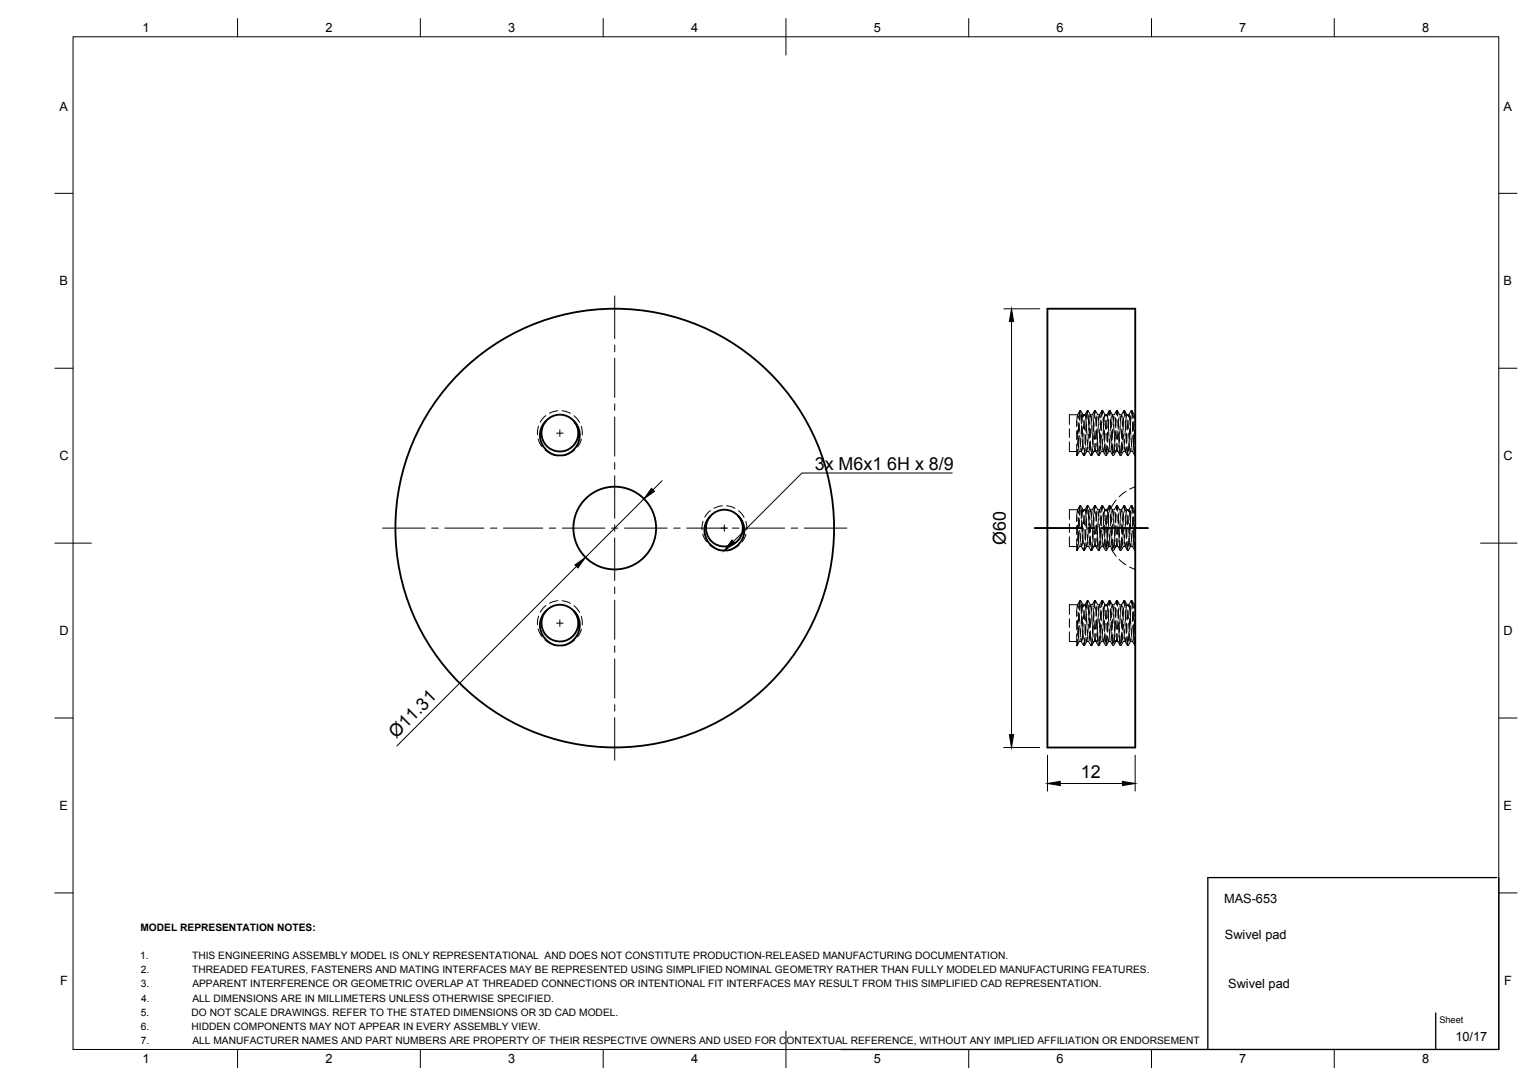
ISO-10303-21;
HEADER;
/* Generated by software containing ST-Developer
 * from STEP Tools, Inc. (www.steptools.com) 
 */

FILE_DESCRIPTION(
/* description */ ('Independent compact industrial fixture table, bolted aluminum worktop
 on connected adjustable support base. Whole-mm nominal dimensions. No
 load rating assigned.'),
/* implementation_level */ '2;1');

FILE_NAME(
/* name */ 'Swivel pad.step',
/* time_stamp */ '2026-11-07T17:47:58-08:00',
/* author */ (''),
/* organization */ (''),
/* preprocessor_version */ 'ST-DEVELOPER v20.2',
/* originating_system */ 'Autodesk Translation Framework v15.17.0.0',
/* authorisation */ '');

FILE_SCHEMA (('AUTOMOTIVE_DESIGN { 1 0 10303 214 3 1 1 }'));
ENDSEC;

DATA;
#10=MECHANICAL_DESIGN_GEOMETRIC_PRESENTATION_REPRESENTATION('',(#2259),#97475);
#11=SPHERICAL_SURFACE('',#22780,6.);
#350=B_SPLINE_SURFACE_WITH_KNOTS('',3,3,((#58329,#58330,#58331,#58332,#58333,
#58334,#58335,#58336,#58337,#58338,#58339,#58340,#58341,#58342,#58343,#58344,
#58345,#58346,#58347,#58348,#58349,#58350,#58351,#58352,#58353,#58354,#58355,
#58356,#58357,#58358,#58359,#58360,#58361,#58362,#58363,#58364,#58365,#58366,
#58367,#58368,#58369,#58370,#58371,#58372,#58373,#58374,#58375,#58376,#58377,
#58378,#58379,#58380,#58381,#58382,#58383,#58384),(#58385,#58386,#58387,
#58388,#58389,#58390,#58391,#58392,#58393,#58394,#58395,#58396,#58397,#58398,
#58399,#58400,#58401,#58402,#58403,#58404,#58405,#58406,#58407,#58408,#58409,
#58410,#58411,#58412,#58413,#58414,#58415,#58416,#58417,#58418,#58419,#58420,
#58421,#58422,#58423,#58424,#58425,#58426,#58427,#58428,#58429,#58430,#58431,
#58432,#58433,#58434,#58435,#58436,#58437,#58438,#58439,#58440),(#58441,
#58442,#58443,#58444,#58445,#58446,#58447,#58448,#58449,#58450,#58451,#58452,
#58453,#58454,#58455,#58456,#58457,#58458,#58459,#58460,#58461,#58462,#58463,
#58464,#58465,#58466,#58467,#58468,#58469,#58470,#58471,#58472,#58473,#58474,
#58475,#58476,#58477,#58478,#58479,#58480,#58481,#58482,#58483,#58484,#58485,
#58486,#58487,#58488,#58489,#58490,#58491,#58492,#58493,#58494,#58495,#58496),
(#58497,#58498,#58499,#58500,#58501,#58502,#58503,#58504,#58505,#58506,
#58507,#58508,#58509,#58510,#58511,#58512,#58513,#58514,#58515,#58516,#58517,
#58518,#58519,#58520,#58521,#58522,#58523,#58524,#58525,#58526,#58527,#58528,
#58529,#58530,#58531,#58532,#58533,#58534,#58535,#58536,#58537,#58538,#58539,
#58540,#58541,#58542,#58543,#58544,#58545,#58546,#58547,#58548,#58549,#58550,
#58551,#58552)),.UNSPECIFIED.,.F.,.F.,.F.,(4,4),(4,1,1,1,1,1,1,1,1,1,1,
1,1,1,1,1,1,1,1,1,1,1,1,1,1,1,1,1,1,1,1,1,1,1,1,1,1,1,1,1,1,1,1,1,1,1,1,
1,1,1,1,1,1,4),(0.,0.0642013499338863),(11.8589888623078,12.8454497557128,
13.8319106491178,14.8183715425228,15.8048324359278,16.7912933293328,17.7777542227378,
18.7642151161429,19.7506760095479,20.7371369029529,21.7235977963579,22.7100586897629,
23.6965195831679,24.6829804765729,25.6694413699779,26.6559022633829,27.6423631567879,
28.6288240501929,29.6152849435979,30.6017458370029,31.5882067304079,32.5746676238129,
33.5611285172179,34.5475894106229,35.5340503040279,36.5205111974329,37.5069720908379,
38.4934329842429,39.4798938776479,40.4663547710529,41.4528156644579,42.4392765578629,
43.4257374512679,44.4121983446729,45.3986592380779,46.3851201314829,47.3715810248879,
48.3580419182929,49.3445028116979,50.3309637051029,51.3174245985079,52.3038854919129,
53.2903463853179,54.2768072787229,55.2632681721279,56.2497290655329,57.2361899589379,
58.222650852343,59.209111745748,60.195572639153,61.182033532558,62.168494425963,
63.154955319368,64.141416212773),.UNSPECIFIED.);
#351=B_SPLINE_SURFACE_WITH_KNOTS('',3,3,((#58669,#58670,#58671,#58672,#58673,
#58674,#58675,#58676,#58677,#58678,#58679,#58680,#58681,#58682,#58683,#58684,
#58685,#58686,#58687,#58688,#58689,#58690,#58691,#58692,#58693,#58694,#58695,
#58696,#58697,#58698,#58699,#58700,#58701,#58702,#58703,#58704,#58705,#58706,
#58707,#58708,#58709,#58710,#58711,#58712,#58713,#58714,#58715,#58716,#58717,
#58718,#58719,#58720,#58721,#58722,#58723,#58724),(#58725,#58726,#58727,
#58728,#58729,#58730,#58731,#58732,#58733,#58734,#58735,#58736,#58737,#58738,
#58739,#58740,#58741,#58742,#58743,#58744,#58745,#58746,#58747,#58748,#58749,
#58750,#58751,#58752,#58753,#58754,#58755,#58756,#58757,#58758,#58759,#58760,
#58761,#58762,#58763,#58764,#58765,#58766,#58767,#58768,#58769,#58770,#58771,
#58772,#58773,#58774,#58775,#58776,#58777,#58778,#58779,#58780),(#58781,
#58782,#58783,#58784,#58785,#58786,#58787,#58788,#58789,#58790,#58791,#58792,
#58793,#58794,#58795,#58796,#58797,#58798,#58799,#58800,#58801,#58802,#58803,
#58804,#58805,#58806,#58807,#58808,#58809,#58810,#58811,#58812,#58813,#58814,
#58815,#58816,#58817,#58818,#58819,#58820,#58821,#58822,#58823,#58824,#58825,
#58826,#58827,#58828,#58829,#58830,#58831,#58832,#58833,#58834,#58835,#58836),
(#58837,#58838,#58839,#58840,#58841,#58842,#58843,#58844,#58845,#58846,
#58847,#58848,#58849,#58850,#58851,#58852,#58853,#58854,#58855,#58856,#58857,
#58858,#58859,#58860,#58861,#58862,#58863,#58864,#58865,#58866,#58867,#58868,
#58869,#58870,#58871,#58872,#58873,#58874,#58875,#58876,#58877,#58878,#58879,
#58880,#58881,#58882,#58883,#58884,#58885,#58886,#58887,#58888,#58889,#58890,
#58891,#58892)),.UNSPECIFIED.,.F.,.F.,.F.,(4,4),(4,1,1,1,1,1,1,1,1,1,1,
1,1,1,1,1,1,1,1,1,1,1,1,1,1,1,1,1,1,1,1,1,1,1,1,1,1,1,1,1,1,1,1,1,1,1,1,
1,1,1,1,1,1,4),(0.,0.0642013499338863),(14.3984001269719,15.3848610203769,
16.3713219137819,17.3577828071869,18.3442437005919,19.3307045939969,20.3171654874019,
21.3036263808069,22.2900872742119,23.2765481676169,24.2630090610219,25.2494699544269,
26.2359308478319,27.2223917412369,28.2088526346419,29.1953135280469,30.1817744214519,
31.1682353148569,32.1546962082619,33.1411571016669,34.1276179950719,35.1140788884769,
36.1005397818819,37.0870006752869,38.0734615686919,39.0599224620969,40.0463833555019,
41.0328442489069,42.0193051423119,43.0057660357169,43.9922269291219,44.978687822527,
45.965148715932,46.951609609337,47.938070502742,48.924531396147,49.910992289552,
50.897453182957,51.883914076362,52.870374969767,53.856835863172,54.843296756577,
55.829757649982,56.816218543387,57.802679436792,58.789140330197,59.775601223602,
60.762062117007,61.748523010412,62.734983903817,63.721444797222,64.707905690627,
65.694366584032,66.680827477437),.UNSPECIFIED.);
#352=B_SPLINE_SURFACE_WITH_KNOTS('',3,3,((#59221,#59222,#59223,#59224,#59225,
#59226,#59227,#59228,#59229,#59230,#59231,#59232,#59233,#59234,#59235,#59236,
#59237,#59238,#59239,#59240,#59241,#59242,#59243,#59244,#59245,#59246,#59247,
#59248,#59249,#59250,#59251,#59252,#59253,#59254,#59255,#59256,#59257,#59258,
#59259,#59260,#59261,#59262,#59263,#59264,#59265,#59266,#59267,#59268,#59269,
#59270,#59271,#59272,#59273,#59274,#59275,#59276),(#59277,#59278,#59279,
#59280,#59281,#59282,#59283,#59284,#59285,#59286,#59287,#59288,#59289,#59290,
#59291,#59292,#59293,#59294,#59295,#59296,#59297,#59298,#59299,#59300,#59301,
#59302,#59303,#59304,#59305,#59306,#59307,#59308,#59309,#59310,#59311,#59312,
#59313,#59314,#59315,#59316,#59317,#59318,#59319,#59320,#59321,#59322,#59323,
#59324,#59325,#59326,#59327,#59328,#59329,#59330,#59331,#59332),(#59333,
#59334,#59335,#59336,#59337,#59338,#59339,#59340,#59341,#59342,#59343,#59344,
#59345,#59346,#59347,#59348,#59349,#59350,#59351,#59352,#59353,#59354,#59355,
#59356,#59357,#59358,#59359,#59360,#59361,#59362,#59363,#59364,#59365,#59366,
#59367,#59368,#59369,#59370,#59371,#59372,#59373,#59374,#59375,#59376,#59377,
#59378,#59379,#59380,#59381,#59382,#59383,#59384,#59385,#59386,#59387,#59388),
(#59389,#59390,#59391,#59392,#59393,#59394,#59395,#59396,#59397,#59398,
#59399,#59400,#59401,#59402,#59403,#59404,#59405,#59406,#59407,#59408,#59409,
#59410,#59411,#59412,#59413,#59414,#59415,#59416,#59417,#59418,#59419,#59420,
#59421,#59422,#59423,#59424,#59425,#59426,#59427,#59428,#59429,#59430,#59431,
#59432,#59433,#59434,#59435,#59436,#59437,#59438,#59439,#59440,#59441,#59442,
#59443,#59444)),.UNSPECIFIED.,.F.,.F.,.F.,(4,4),(4,1,1,1,1,1,1,1,1,1,1,
1,1,1,1,1,1,1,1,1,1,1,1,1,1,1,1,1,1,1,1,1,1,1,1,1,1,1,1,1,1,1,1,1,1,1,1,
1,1,1,1,1,1,4),(0.,0.0642013499338863),(11.8589888623078,12.8454497557128,
13.8319106491178,14.8183715425228,15.8048324359278,16.7912933293328,17.7777542227378,
18.7642151161428,19.7506760095478,20.7371369029528,21.7235977963578,22.7100586897628,
23.6965195831678,24.6829804765729,25.6694413699779,26.6559022633829,27.6423631567879,
28.6288240501929,29.6152849435979,30.6017458370029,31.5882067304079,32.5746676238129,
33.5611285172179,34.5475894106229,35.5340503040279,36.5205111974329,37.5069720908379,
38.4934329842429,39.4798938776479,40.4663547710529,41.4528156644579,42.4392765578629,
43.4257374512679,44.4121983446729,45.3986592380779,46.3851201314829,47.3715810248879,
48.3580419182929,49.3445028116979,50.3309637051029,51.3174245985079,52.3038854919129,
53.2903463853179,54.2768072787229,55.2632681721279,56.2497290655329,57.2361899589379,
58.2226508523429,59.2091117457479,60.1955726391529,61.1820335325579,62.1684944259629,
63.154955319368,64.141416212773),.UNSPECIFIED.);
#353=B_SPLINE_SURFACE_WITH_KNOTS('',3,3,((#59561,#59562,#59563,#59564,#59565,
#59566,#59567,#59568,#59569,#59570,#59571,#59572,#59573,#59574,#59575,#59576,
#59577,#59578,#59579,#59580,#59581,#59582,#59583,#59584,#59585,#59586,#59587,
#59588,#59589,#59590,#59591,#59592,#59593,#59594,#59595,#59596,#59597,#59598,
#59599,#59600,#59601,#59602,#59603,#59604,#59605,#59606,#59607,#59608,#59609,
#59610,#59611,#59612,#59613,#59614,#59615,#59616),(#59617,#59618,#59619,
#59620,#59621,#59622,#59623,#59624,#59625,#59626,#59627,#59628,#59629,#59630,
#59631,#59632,#59633,#59634,#59635,#59636,#59637,#59638,#59639,#59640,#59641,
#59642,#59643,#59644,#59645,#59646,#59647,#59648,#59649,#59650,#59651,#59652,
#59653,#59654,#59655,#59656,#59657,#59658,#59659,#59660,#59661,#59662,#59663,
#59664,#59665,#59666,#59667,#59668,#59669,#59670,#59671,#59672),(#59673,
#59674,#59675,#59676,#59677,#59678,#59679,#59680,#59681,#59682,#59683,#59684,
#59685,#59686,#59687,#59688,#59689,#59690,#59691,#59692,#59693,#59694,#59695,
#59696,#59697,#59698,#59699,#59700,#59701,#59702,#59703,#59704,#59705,#59706,
#59707,#59708,#59709,#59710,#59711,#59712,#59713,#59714,#59715,#59716,#59717,
#59718,#59719,#59720,#59721,#59722,#59723,#59724,#59725,#59726,#59727,#59728),
(#59729,#59730,#59731,#59732,#59733,#59734,#59735,#59736,#59737,#59738,
#59739,#59740,#59741,#59742,#59743,#59744,#59745,#59746,#59747,#59748,#59749,
#59750,#59751,#59752,#59753,#59754,#59755,#59756,#59757,#59758,#59759,#59760,
#59761,#59762,#59763,#59764,#59765,#59766,#59767,#59768,#59769,#59770,#59771,
#59772,#59773,#59774,#59775,#59776,#59777,#59778,#59779,#59780,#59781,#59782,
#59783,#59784)),.UNSPECIFIED.,.F.,.F.,.F.,(4,4),(4,1,1,1,1,1,1,1,1,1,1,
1,1,1,1,1,1,1,1,1,1,1,1,1,1,1,1,1,1,1,1,1,1,1,1,1,1,1,1,1,1,1,1,1,1,1,1,
1,1,1,1,1,1,4),(0.,0.0642013499338863),(14.3984001269719,15.3848610203769,
16.3713219137819,17.3577828071869,18.3442437005919,19.3307045939969,20.3171654874019,
21.3036263808069,22.2900872742119,23.2765481676169,24.2630090610219,25.2494699544269,
26.2359308478319,27.2223917412369,28.2088526346419,29.1953135280469,30.1817744214519,
31.1682353148569,32.1546962082619,33.1411571016669,34.1276179950719,35.1140788884769,
36.1005397818819,37.0870006752869,38.0734615686919,39.0599224620969,40.0463833555019,
41.0328442489069,42.0193051423119,43.0057660357169,43.9922269291219,44.9786878225269,
45.9651487159319,46.9516096093369,47.9380705027419,48.9245313961469,49.9109922895519,
50.897453182957,51.883914076362,52.870374969767,53.856835863172,54.843296756577,
55.829757649982,56.816218543387,57.802679436792,58.789140330197,59.775601223602,
60.762062117007,61.748523010412,62.734983903817,63.721444797222,64.707905690627,
65.694366584032,66.680827477437),.UNSPECIFIED.);
#354=B_SPLINE_SURFACE_WITH_KNOTS('',3,3,((#60113,#60114,#60115,#60116,#60117,
#60118,#60119,#60120,#60121,#60122,#60123,#60124,#60125,#60126,#60127,#60128,
#60129,#60130,#60131,#60132,#60133,#60134,#60135,#60136,#60137,#60138,#60139,
#60140,#60141,#60142,#60143,#60144,#60145,#60146,#60147,#60148,#60149,#60150,
#60151,#60152,#60153,#60154,#60155,#60156,#60157,#60158,#60159,#60160,#60161,
#60162,#60163,#60164,#60165,#60166,#60167,#60168),(#60169,#60170,#60171,
#60172,#60173,#60174,#60175,#60176,#60177,#60178,#60179,#60180,#60181,#60182,
#60183,#60184,#60185,#60186,#60187,#60188,#60189,#60190,#60191,#60192,#60193,
#60194,#60195,#60196,#60197,#60198,#60199,#60200,#60201,#60202,#60203,#60204,
#60205,#60206,#60207,#60208,#60209,#60210,#60211,#60212,#60213,#60214,#60215,
#60216,#60217,#60218,#60219,#60220,#60221,#60222,#60223,#60224),(#60225,
#60226,#60227,#60228,#60229,#60230,#60231,#60232,#60233,#60234,#60235,#60236,
#60237,#60238,#60239,#60240,#60241,#60242,#60243,#60244,#60245,#60246,#60247,
#60248,#60249,#60250,#60251,#60252,#60253,#60254,#60255,#60256,#60257,#60258,
#60259,#60260,#60261,#60262,#60263,#60264,#60265,#60266,#60267,#60268,#60269,
#60270,#60271,#60272,#60273,#60274,#60275,#60276,#60277,#60278,#60279,#60280),
(#60281,#60282,#60283,#60284,#60285,#60286,#60287,#60288,#60289,#60290,
#60291,#60292,#60293,#60294,#60295,#60296,#60297,#60298,#60299,#60300,#60301,
#60302,#60303,#60304,#60305,#60306,#60307,#60308,#60309,#60310,#60311,#60312,
#60313,#60314,#60315,#60316,#60317,#60318,#60319,#60320,#60321,#60322,#60323,
#60324,#60325,#60326,#60327,#60328,#60329,#60330,#60331,#60332,#60333,#60334,
#60335,#60336)),.UNSPECIFIED.,.F.,.F.,.F.,(4,4),(4,1,1,1,1,1,1,1,1,1,1,
1,1,1,1,1,1,1,1,1,1,1,1,1,1,1,1,1,1,1,1,1,1,1,1,1,1,1,1,1,1,1,1,1,1,1,1,
1,1,1,1,1,1,4),(0.,0.0642013499338865),(11.8589888623078,12.8454497557128,
13.8319106491178,14.8183715425228,15.8048324359278,16.7912933293328,17.7777542227378,
18.7642151161428,19.7506760095478,20.7371369029528,21.7235977963578,22.7100586897628,
23.6965195831678,24.6829804765729,25.6694413699779,26.6559022633829,27.6423631567879,
28.6288240501929,29.6152849435979,30.6017458370029,31.5882067304079,32.5746676238129,
33.5611285172179,34.5475894106229,35.5340503040279,36.5205111974329,37.5069720908379,
38.4934329842429,39.4798938776479,40.4663547710529,41.4528156644579,42.4392765578629,
43.4257374512679,44.4121983446729,45.3986592380779,46.3851201314829,47.3715810248879,
48.3580419182929,49.3445028116979,50.3309637051029,51.3174245985079,52.3038854919129,
53.2903463853179,54.2768072787229,55.2632681721279,56.2497290655329,57.2361899589379,
58.2226508523429,59.2091117457479,60.1955726391529,61.1820335325579,62.1684944259629,
63.154955319368,64.141416212773),.UNSPECIFIED.);
#355=B_SPLINE_SURFACE_WITH_KNOTS('',3,3,((#60453,#60454,#60455,#60456,#60457,
#60458,#60459,#60460,#60461,#60462,#60463,#60464,#60465,#60466,#60467,#60468,
#60469,#60470,#60471,#60472,#60473,#60474,#60475,#60476,#60477,#60478,#60479,
#60480,#60481,#60482,#60483,#60484,#60485,#60486,#60487,#60488,#60489,#60490,
#60491,#60492,#60493,#60494,#60495,#60496,#60497,#60498,#60499,#60500,#60501,
#60502,#60503,#60504,#60505,#60506,#60507,#60508),(#60509,#60510,#60511,
#60512,#60513,#60514,#60515,#60516,#60517,#60518,#60519,#60520,#60521,#60522,
#60523,#60524,#60525,#60526,#60527,#60528,#60529,#60530,#60531,#60532,#60533,
#60534,#60535,#60536,#60537,#60538,#60539,#60540,#60541,#60542,#60543,#60544,
#60545,#60546,#60547,#60548,#60549,#60550,#60551,#60552,#60553,#60554,#60555,
#60556,#60557,#60558,#60559,#60560,#60561,#60562,#60563,#60564),(#60565,
#60566,#60567,#60568,#60569,#60570,#60571,#60572,#60573,#60574,#60575,#60576,
#60577,#60578,#60579,#60580,#60581,#60582,#60583,#60584,#60585,#60586,#60587,
#60588,#60589,#60590,#60591,#60592,#60593,#60594,#60595,#60596,#60597,#60598,
#60599,#60600,#60601,#60602,#60603,#60604,#60605,#60606,#60607,#60608,#60609,
#60610,#60611,#60612,#60613,#60614,#60615,#60616,#60617,#60618,#60619,#60620),
(#60621,#60622,#60623,#60624,#60625,#60626,#60627,#60628,#60629,#60630,
#60631,#60632,#60633,#60634,#60635,#60636,#60637,#60638,#60639,#60640,#60641,
#60642,#60643,#60644,#60645,#60646,#60647,#60648,#60649,#60650,#60651,#60652,
#60653,#60654,#60655,#60656,#60657,#60658,#60659,#60660,#60661,#60662,#60663,
#60664,#60665,#60666,#60667,#60668,#60669,#60670,#60671,#60672,#60673,#60674,
#60675,#60676)),.UNSPECIFIED.,.F.,.F.,.F.,(4,4),(4,1,1,1,1,1,1,1,1,1,1,
1,1,1,1,1,1,1,1,1,1,1,1,1,1,1,1,1,1,1,1,1,1,1,1,1,1,1,1,1,1,1,1,1,1,1,1,
1,1,1,1,1,1,4),(0.,0.0642013499338865),(14.3984001269719,15.3848610203769,
16.3713219137819,17.3577828071869,18.3442437005919,19.3307045939969,20.3171654874019,
21.3036263808069,22.2900872742119,23.2765481676169,24.2630090610219,25.2494699544269,
26.2359308478319,27.2223917412369,28.2088526346419,29.1953135280469,30.1817744214519,
31.1682353148569,32.1546962082619,33.1411571016669,34.1276179950719,35.1140788884769,
36.1005397818819,37.0870006752869,38.0734615686919,39.0599224620969,40.0463833555019,
41.0328442489069,42.0193051423119,43.0057660357169,43.9922269291219,44.9786878225269,
45.9651487159319,46.9516096093369,47.9380705027419,48.9245313961469,49.9109922895519,
50.897453182957,51.883914076362,52.870374969767,53.856835863172,54.843296756577,
55.829757649982,56.816218543387,57.802679436792,58.789140330197,59.775601223602,
60.762062117007,61.748523010412,62.734983903817,63.721444797222,64.707905690627,
65.694366584032,66.680827477437),.UNSPECIFIED.);
#1002=B_SPLINE_CURVE_WITH_KNOTS('',3,(#56458,#56459,#56460,#56461),
 .UNSPECIFIED.,.F.,.F.,(4,4),(51.5750455984138,52.2824273504651),
 .UNSPECIFIED.);
#1003=B_SPLINE_CURVE_WITH_KNOTS('',3,(#56469,#56470,#56471,#56472,#56473,
#56474,#56475,#56476,#56477,#56478),.UNSPECIFIED.,.F.,.F.,(4,3,3,4),(-50.2654824574367,
-49.3230446702501,-48.3365837768451,-47.8312715558982),.UNSPECIFIED.);
#1004=B_SPLINE_CURVE_WITH_KNOTS('',3,(#56483,#56484,#56485,#56486,#56487,
#56488,#56489,#56490,#56491,#56492,#56493,#56494,#56495,#56496,#56497,#56498,
#56499,#56500,#56501,#56502,#56503,#56504,#56505,#56506,#56507),
 .UNSPECIFIED.,.F.,.F.,(4,3,3,3,3,3,3,3,4),(45.2918602912342,45.3772010966301,
46.3636619900351,47.3501228834401,48.3365837768451,49.3230446702501,50.3095055636551,
51.2959664570601,51.5750455984138),.UNSPECIFIED.);
#1005=B_SPLINE_CURVE_WITH_KNOTS('',3,(#56508,#56509,#56510,#56511,#56512,
#56513,#56514,#56515,#56516,#56517,#56518,#56519,#56520,#56521,#56522,#56523,
#56524,#56525,#56526,#56527,#56528,#56529),.UNSPECIFIED.,.F.,.F.,(4,3,3,
3,3,3,3,4),(-47.8312715558982,-47.3501228834401,-46.3636619900351,-45.3772010966301,
-44.3907402032251,-43.4042793098201,-42.4178184164151,-41.5480862487186),
 .UNSPECIFIED.);
#1006=B_SPLINE_CURVE_WITH_KNOTS('',3,(#56534,#56535,#56536,#56537,#56538,
#56539,#56540,#56541,#56542,#56543,#56544,#56545,#56546,#56547,#56548,#56549,
#56550,#56551,#56552,#56553,#56554,#56555),.UNSPECIFIED.,.F.,.F.,(4,3,3,
3,3,3,3,4),(39.0086749840546,39.4584357362001,40.4448966296051,41.4313575230101,
42.4178184164151,43.4042793098201,44.3907402032251,45.2918602912342),
 .UNSPECIFIED.);
#1007=B_SPLINE_CURVE_WITH_KNOTS('',3,(#56556,#56557,#56558,#56559,#56560,
#56561,#56562,#56563,#56564,#56565,#56566,#56567,#56568,#56569,#56570,#56571,
#56572,#56573,#56574,#56575,#56576,#56577,#56578,#56579,#56580),
 .UNSPECIFIED.,.F.,.F.,(4,3,3,3,3,3,3,3,4),(-41.5480862487186,-41.4313575230101,
-40.4448966296051,-39.4584357362001,-38.4719748427951,-37.4855139493901,
-36.4990530559851,-35.5125921625801,-35.2649009415391),.UNSPECIFIED.);
#1008=B_SPLINE_CURVE_WITH_KNOTS('',3,(#56585,#56586,#56587,#56588,#56589,
#56590,#56591,#56592,#56593,#56594,#56595,#56596,#56597,#56598,#56599,#56600,
#56601,#56602,#56603,#56604,#56605,#56606),.UNSPECIFIED.,.F.,.F.,(4,3,3,
3,3,3,3,4),(32.725489676875,33.5396703757701,34.5261312691751,35.5125921625801,
36.4990530559851,37.4855139493901,38.4719748427951,39.0086749840546),
 .UNSPECIFIED.);
#1009=B_SPLINE_CURVE_WITH_KNOTS('',3,(#56607,#56608,#56609,#56610,#56611,
#56612,#56613,#56614,#56615,#56616,#56617,#56618,#56619,#56620,#56621,#56622,
#56623,#56624,#56625,#56626,#56627,#56628),.UNSPECIFIED.,.F.,.F.,(4,3,3,
3,3,3,3,4),(-35.2649009415391,-34.5261312691751,-33.5396703757701,-32.5532094823651,
-31.5667485889601,-30.5802876955551,-29.5938268021501,-28.9817156343595),
 .UNSPECIFIED.);
#1010=B_SPLINE_CURVE_WITH_KNOTS('',3,(#56633,#56634,#56635,#56636,#56637,
#56638,#56639,#56640,#56641,#56642,#56643,#56644,#56645,#56646,#56647,#56648,
#56649,#56650,#56651,#56652,#56653,#56654,#56655,#56656,#56657),
 .UNSPECIFIED.,.F.,.F.,(4,3,3,3,3,3,3,3,4),(26.4423043696954,26.6344441219351,
27.6209050153401,28.6073659087451,29.5938268021501,30.5802876955551,31.5667485889601,
32.5532094823651,32.725489676875),.UNSPECIFIED.);
#1011=B_SPLINE_CURVE_WITH_KNOTS('',3,(#56658,#56659,#56660,#56661,#56662,
#56663,#56664,#56665,#56666,#56667,#56668,#56669,#56670,#56671,#56672,#56673,
#56674,#56675,#56676,#56677,#56678,#56679),.UNSPECIFIED.,.F.,.F.,(4,3,3,
3,3,3,3,4),(-28.9817156343595,-28.6073659087451,-27.6209050153401,-26.6344441219351,
-25.6479832285301,-24.6615223351251,-23.6750614417201,-22.6985303271799),
 .UNSPECIFIED.);
#1012=B_SPLINE_CURVE_WITH_KNOTS('',3,(#56684,#56685,#56686,#56687,#56688,
#56689,#56690,#56691,#56692,#56693,#56694,#56695,#56696,#56697,#56698,#56699,
#56700,#56701,#56702,#56703,#56704,#56705),.UNSPECIFIED.,.F.,.F.,(4,3,3,
3,3,3,3,4),(20.1591190625158,20.7156787615051,21.7021396549101,22.6886005483151,
23.6750614417201,24.6615223351251,25.6479832285301,26.4423043696954),
 .UNSPECIFIED.);
#1013=B_SPLINE_CURVE_WITH_KNOTS('',3,(#56706,#56707,#56708,#56709,#56710,
#56711,#56712,#56713,#56714,#56715,#56716,#56717,#56718,#56719,#56720,#56721,
#56722,#56723,#56724,#56725,#56726,#56727,#56728,#56729,#56730),
 .UNSPECIFIED.,.F.,.F.,(4,3,3,3,3,3,3,3,4),(-22.6985303271799,-22.6886005483151,
-21.7021396549101,-20.7156787615051,-19.7292178681001,-18.742756974695,
-17.75629608129,-16.769835187885,-16.4153450200003),.UNSPECIFIED.);
#1014=B_SPLINE_CURVE_WITH_KNOTS('',3,(#56735,#56736,#56737,#56738,#56739,
#56740,#56741,#56742,#56743,#56744,#56745,#56746,#56747,#56748,#56749,#56750,
#56751,#56752,#56753,#56754,#56755,#56756),.UNSPECIFIED.,.F.,.F.,(4,3,3,
3,3,3,3,4),(13.8759337553362,14.796913401075,15.78337429448,16.769835187885,
17.75629608129,18.7427569746951,19.7292178681001,20.1591190625158),
 .UNSPECIFIED.);
#1015=B_SPLINE_CURVE_WITH_KNOTS('',3,(#56757,#56758,#56759,#56760,#56761,
#56762,#56763,#56764,#56765,#56766,#56767,#56768,#56769,#56770,#56771,#56772,
#56773,#56774,#56775,#56776,#56777,#56778),.UNSPECIFIED.,.F.,.F.,(4,3,3,
3,3,3,3,4),(-16.4153450200003,-15.78337429448,-14.796913401075,-13.81045250767,
-12.823991614265,-11.83753072086,-10.851069827455,-10.1321597128207),
 .UNSPECIFIED.);
#1016=B_SPLINE_CURVE_WITH_KNOTS('',3,(#56784,#56785,#56786,#56787,#56788,
#56789,#56790,#56791,#56792,#56793,#56794,#56795,#56796),.UNSPECIFIED.,
 .F.,.F.,(4,3,3,3,4),(-3.84897440564113,-2.95938268021501,-1.97292178681001,
-0.986460893405003,0.),.UNSPECIFIED.);
#1017=B_SPLINE_CURVE_WITH_KNOTS('',3,(#56799,#56800,#56801,#56802,#56803,
#56804,#56805,#56806,#56807,#56808,#56809,#56810,#56811,#56812,#56813,#56814,
#56815,#56816,#56817),.UNSPECIFIED.,.F.,.F.,(4,3,3,3,3,3,4),(2.01694489302845,
2.95938268021501,3.94584357362001,4.93230446702502,5.91876536043002,6.90522625383502,
7.59274844815666),.UNSPECIFIED.);
#1018=B_SPLINE_CURVE_WITH_KNOTS('',3,(#56823,#56824,#56825,#56826,#56827,
#56828,#56829,#56830),.UNSPECIFIED.,.F.,.F.,(4,1,1,1,1,4),(59.6902604182061,
60.1955726391529,61.1820335325579,62.1684944259629,63.154955319368,64.141416212773),
 .UNSPECIFIED.);
#1019=B_SPLINE_CURVE_WITH_KNOTS('',3,(#56833,#56834,#56835,#56836,#56837,
#56838,#56839,#56840,#56841),.UNSPECIFIED.,.F.,.F.,(4,1,1,1,1,1,4),(59.6902604182061,
59.775601223602,60.762062117007,61.748523010412,62.734983903817,63.721444797222,
64.6638825844085),.UNSPECIFIED.);
#1020=B_SPLINE_CURVE_WITH_KNOTS('',3,(#56846,#56847,#56848,#56849,#56850,
#56851,#56852,#56853,#56854,#56855),.UNSPECIFIED.,.F.,.F.,(4,1,1,1,1,1,
1,4),(53.4070751110265,54.2768072787229,55.2632681721279,56.2497290655329,
57.2361899589379,58.2226508523429,59.2091117457479,59.6902604182061),
 .UNSPECIFIED.);
#1021=B_SPLINE_CURVE_WITH_KNOTS('',3,(#56856,#56857,#56858,#56859,#56860,
#56861,#56862,#56863,#56864,#56865),.UNSPECIFIED.,.F.,.F.,(4,1,1,1,1,1,
1,4),(53.4070751110265,53.856835863172,54.843296756577,55.829757649982,
56.816218543387,57.802679436792,58.789140330197,59.6902604182061),
 .UNSPECIFIED.);
#1022=B_SPLINE_CURVE_WITH_KNOTS('',3,(#56870,#56871,#56872,#56873,#56874,
#56875,#56876,#56877,#56878,#56879,#56880),.UNSPECIFIED.,.F.,.F.,(4,1,1,
1,1,1,1,1,4),(47.1238898038469,47.3715810248879,48.3580419182929,49.3445028116979,
50.3309637051029,51.3174245985079,52.3038854919129,53.2903463853179,53.4070751110265),
 .UNSPECIFIED.);
#1023=B_SPLINE_CURVE_WITH_KNOTS('',3,(#56881,#56882,#56883,#56884,#56885,
#56886,#56887,#56888,#56889,#56890),.UNSPECIFIED.,.F.,.F.,(4,1,1,1,1,1,
1,4),(47.1238898038469,47.9380705027419,48.9245313961469,49.9109922895519,
50.897453182957,51.883914076362,52.870374969767,53.4070751110265),
 .UNSPECIFIED.);
#1024=B_SPLINE_CURVE_WITH_KNOTS('',3,(#56895,#56896,#56897,#56898,#56899,
#56900,#56901,#56902,#56903,#56904),.UNSPECIFIED.,.F.,.F.,(4,1,1,1,1,1,
1,4),(40.8407044966673,41.4528156644579,42.4392765578629,43.4257374512679,
44.4121983446729,45.3986592380779,46.3851201314829,47.1238898038469),
 .UNSPECIFIED.);
#1025=B_SPLINE_CURVE_WITH_KNOTS('',3,(#56905,#56906,#56907,#56908,#56909,
#56910,#56911,#56912,#56913,#56914,#56915),.UNSPECIFIED.,.F.,.F.,(4,1,1,
1,1,1,1,1,4),(40.8407044966673,41.0328442489069,42.0193051423119,43.0057660357169,
43.9922269291219,44.9786878225269,45.9651487159319,46.9516096093369,47.1238898038469),
 .UNSPECIFIED.);
#1026=B_SPLINE_CURVE_WITH_KNOTS('',3,(#56920,#56921,#56922,#56923,#56924,
#56925,#56926,#56927,#56928,#56929),.UNSPECIFIED.,.F.,.F.,(4,1,1,1,1,1,
1,4),(34.5575191894877,35.5340503040279,36.5205111974329,37.5069720908379,
38.4934329842429,39.4798938776479,40.4663547710529,40.8407044966673),
 .UNSPECIFIED.);
#1027=B_SPLINE_CURVE_WITH_KNOTS('',3,(#56930,#56931,#56932,#56933,#56934,
#56935,#56936,#56937,#56938,#56939),.UNSPECIFIED.,.F.,.F.,(4,1,1,1,1,1,
1,4),(34.5575191894877,35.1140788884769,36.1005397818819,37.0870006752869,
38.0734615686919,39.0599224620969,40.0463833555019,40.8407044966673),
 .UNSPECIFIED.);
#1028=B_SPLINE_CURVE_WITH_KNOTS('',3,(#56944,#56945,#56946,#56947,#56948,
#56949,#56950,#56951,#56952,#56953,#56954),.UNSPECIFIED.,.F.,.F.,(4,1,1,
1,1,1,1,1,4),(28.2743338823081,28.6288240501929,29.6152849435979,30.6017458370029,
31.5882067304079,32.5746676238129,33.5611285172179,34.5475894106229,34.5575191894877),
 .UNSPECIFIED.);
#1029=B_SPLINE_CURVE_WITH_KNOTS('',3,(#56955,#56956,#56957,#56958,#56959,
#56960,#56961,#56962,#56963,#56964),.UNSPECIFIED.,.F.,.F.,(4,1,1,1,1,1,
1,4),(28.2743338823081,29.1953135280469,30.1817744214519,31.1682353148569,
32.1546962082619,33.1411571016669,34.1276179950719,34.5575191894877),
 .UNSPECIFIED.);
#1030=B_SPLINE_CURVE_WITH_KNOTS('',3,(#56969,#56970,#56971,#56972,#56973,
#56974,#56975,#56976,#56977,#56978),.UNSPECIFIED.,.F.,.F.,(4,1,1,1,1,1,
1,4),(21.9911485751285,22.7100586897628,23.6965195831678,24.6829804765729,
25.6694413699779,26.6559022633829,27.6423631567879,28.2743338823081),
 .UNSPECIFIED.);
#1031=B_SPLINE_CURVE_WITH_KNOTS('',3,(#56979,#56980,#56981,#56982,#56983,
#56984,#56985,#56986,#56987,#56988,#56989),.UNSPECIFIED.,.F.,.F.,(4,1,1,
1,1,1,1,1,4),(21.9911485751285,22.2900872742119,23.2765481676169,24.2630090610219,
25.2494699544269,26.2359308478319,27.2223917412369,28.2088526346419,28.2743338823081),
 .UNSPECIFIED.);
#1032=B_SPLINE_CURVE_WITH_KNOTS('',3,(#56995,#56996,#56997,#56998,#56999),
 .UNSPECIFIED.,.F.,.F.,(4,1,4),(14.3984001269719,15.3848610203769,15.7079632679489),
 .UNSPECIFIED.);
#1033=B_SPLINE_CURVE_WITH_KNOTS('',3,(#57002,#57003,#57004,#57005,#57006),
 .UNSPECIFIED.,.F.,.F.,(4,1,4),(13.8759337553363,14.8183715425228,15.7079632679489),
 .UNSPECIFIED.);
#1034=B_SPLINE_CURVE_WITH_KNOTS('',3,(#57012,#57013,#57014,#57015),
 .UNSPECIFIED.,.F.,.F.,(4,4),(51.5750455984138,52.2824273504651),
 .UNSPECIFIED.);
#1035=B_SPLINE_CURVE_WITH_KNOTS('',3,(#57023,#57024,#57025,#57026,#57027,
#57028,#57029,#57030,#57031,#57032),.UNSPECIFIED.,.F.,.F.,(4,3,3,4),(-50.2654824574367,
-49.3230446702501,-48.3365837768451,-47.8312715558982),.UNSPECIFIED.);
#1036=B_SPLINE_CURVE_WITH_KNOTS('',3,(#57037,#57038,#57039,#57040,#57041,
#57042,#57043,#57044,#57045,#57046,#57047,#57048,#57049,#57050,#57051,#57052,
#57053,#57054,#57055,#57056,#57057,#57058,#57059,#57060,#57061),
 .UNSPECIFIED.,.F.,.F.,(4,3,3,3,3,3,3,3,4),(45.2918602912342,45.3772010966301,
46.3636619900351,47.3501228834401,48.3365837768451,49.3230446702501,50.3095055636551,
51.2959664570601,51.5750455984138),.UNSPECIFIED.);
#1037=B_SPLINE_CURVE_WITH_KNOTS('',3,(#57062,#57063,#57064,#57065,#57066,
#57067,#57068,#57069,#57070,#57071,#57072,#57073,#57074,#57075,#57076,#57077,
#57078,#57079,#57080,#57081,#57082,#57083),.UNSPECIFIED.,.F.,.F.,(4,3,3,
3,3,3,3,4),(-47.8312715558982,-47.3501228834401,-46.3636619900351,-45.3772010966301,
-44.3907402032251,-43.4042793098201,-42.4178184164151,-41.5480862487186),
 .UNSPECIFIED.);
#1038=B_SPLINE_CURVE_WITH_KNOTS('',3,(#57088,#57089,#57090,#57091,#57092,
#57093,#57094,#57095,#57096,#57097,#57098,#57099,#57100,#57101,#57102,#57103,
#57104,#57105,#57106,#57107,#57108,#57109),.UNSPECIFIED.,.F.,.F.,(4,3,3,
3,3,3,3,4),(39.0086749840546,39.4584357362001,40.4448966296051,41.4313575230101,
42.4178184164151,43.4042793098201,44.3907402032251,45.2918602912342),
 .UNSPECIFIED.);
#1039=B_SPLINE_CURVE_WITH_KNOTS('',3,(#57110,#57111,#57112,#57113,#57114,
#57115,#57116,#57117,#57118,#57119,#57120,#57121,#57122,#57123,#57124,#57125,
#57126,#57127,#57128,#57129,#57130,#57131,#57132,#57133,#57134),
 .UNSPECIFIED.,.F.,.F.,(4,3,3,3,3,3,3,3,4),(-41.5480862487186,-41.4313575230101,
-40.4448966296051,-39.4584357362001,-38.4719748427951,-37.4855139493901,
-36.4990530559851,-35.5125921625801,-35.2649009415391),.UNSPECIFIED.);
#1040=B_SPLINE_CURVE_WITH_KNOTS('',3,(#57139,#57140,#57141,#57142,#57143,
#57144,#57145,#57146,#57147,#57148,#57149,#57150,#57151,#57152,#57153,#57154,
#57155,#57156,#57157,#57158,#57159,#57160),.UNSPECIFIED.,.F.,.F.,(4,3,3,
3,3,3,3,4),(32.725489676875,33.5396703757701,34.5261312691751,35.5125921625801,
36.4990530559851,37.4855139493901,38.4719748427951,39.0086749840546),
 .UNSPECIFIED.);
#1041=B_SPLINE_CURVE_WITH_KNOTS('',3,(#57161,#57162,#57163,#57164,#57165,
#57166,#57167,#57168,#57169,#57170,#57171,#57172,#57173,#57174,#57175,#57176,
#57177,#57178,#57179,#57180,#57181,#57182),.UNSPECIFIED.,.F.,.F.,(4,3,3,
3,3,3,3,4),(-35.2649009415391,-34.5261312691751,-33.5396703757701,-32.5532094823651,
-31.5667485889601,-30.5802876955551,-29.5938268021501,-28.9817156343595),
 .UNSPECIFIED.);
#1042=B_SPLINE_CURVE_WITH_KNOTS('',3,(#57187,#57188,#57189,#57190,#57191,
#57192,#57193,#57194,#57195,#57196,#57197,#57198,#57199,#57200,#57201,#57202,
#57203,#57204,#57205,#57206,#57207,#57208,#57209,#57210,#57211),
 .UNSPECIFIED.,.F.,.F.,(4,3,3,3,3,3,3,3,4),(26.4423043696954,26.6344441219351,
27.6209050153401,28.6073659087451,29.5938268021501,30.5802876955551,31.5667485889601,
32.5532094823651,32.725489676875),.UNSPECIFIED.);
#1043=B_SPLINE_CURVE_WITH_KNOTS('',3,(#57212,#57213,#57214,#57215,#57216,
#57217,#57218,#57219,#57220,#57221,#57222,#57223,#57224,#57225,#57226,#57227,
#57228,#57229,#57230,#57231,#57232,#57233),.UNSPECIFIED.,.F.,.F.,(4,3,3,
3,3,3,3,4),(-28.9817156343595,-28.6073659087451,-27.6209050153401,-26.6344441219351,
-25.6479832285301,-24.6615223351251,-23.6750614417201,-22.6985303271799),
 .UNSPECIFIED.);
#1044=B_SPLINE_CURVE_WITH_KNOTS('',3,(#57238,#57239,#57240,#57241,#57242,
#57243,#57244,#57245,#57246,#57247,#57248,#57249,#57250,#57251,#57252,#57253,
#57254,#57255,#57256,#57257,#57258,#57259),.UNSPECIFIED.,.F.,.F.,(4,3,3,
3,3,3,3,4),(20.1591190625158,20.7156787615051,21.7021396549101,22.6886005483151,
23.6750614417201,24.6615223351251,25.6479832285301,26.4423043696954),
 .UNSPECIFIED.);
#1045=B_SPLINE_CURVE_WITH_KNOTS('',3,(#57260,#57261,#57262,#57263,#57264,
#57265,#57266,#57267,#57268,#57269,#57270,#57271,#57272,#57273,#57274,#57275,
#57276,#57277,#57278,#57279,#57280,#57281,#57282,#57283,#57284),
 .UNSPECIFIED.,.F.,.F.,(4,3,3,3,3,3,3,3,4),(-22.6985303271799,-22.6886005483151,
-21.70213965491,-20.715678761505,-19.7292178681,-18.742756974695,-17.75629608129,
-16.769835187885,-16.4153450200003),.UNSPECIFIED.);
#1046=B_SPLINE_CURVE_WITH_KNOTS('',3,(#57289,#57290,#57291,#57292,#57293,
#57294,#57295,#57296,#57297,#57298,#57299,#57300,#57301,#57302,#57303,#57304,
#57305,#57306,#57307,#57308,#57309,#57310),.UNSPECIFIED.,.F.,.F.,(4,3,3,
3,3,3,3,4),(13.8759337553362,14.796913401075,15.78337429448,16.769835187885,
17.7562960812901,18.7427569746951,19.7292178681001,20.1591190625158),
 .UNSPECIFIED.);
#1047=B_SPLINE_CURVE_WITH_KNOTS('',3,(#57311,#57312,#57313,#57314,#57315,
#57316,#57317,#57318,#57319,#57320,#57321,#57322,#57323,#57324,#57325,#57326,
#57327,#57328,#57329,#57330,#57331,#57332),.UNSPECIFIED.,.F.,.F.,(4,3,3,
3,3,3,3,4),(-16.4153450200003,-15.78337429448,-14.796913401075,-13.81045250767,
-12.823991614265,-11.83753072086,-10.851069827455,-10.1321597128207),
 .UNSPECIFIED.);
#1048=B_SPLINE_CURVE_WITH_KNOTS('',3,(#57338,#57339,#57340,#57341,#57342,
#57343,#57344,#57345,#57346,#57347,#57348,#57349,#57350),.UNSPECIFIED.,
 .F.,.F.,(4,3,3,3,4),(-3.84897440564113,-2.95938268021501,-1.97292178681,
-0.986460893405001,0.),.UNSPECIFIED.);
#1049=B_SPLINE_CURVE_WITH_KNOTS('',3,(#57353,#57354,#57355,#57356,#57357,
#57358,#57359,#57360,#57361,#57362,#57363,#57364,#57365,#57366,#57367,#57368,
#57369,#57370,#57371),.UNSPECIFIED.,.F.,.F.,(4,3,3,3,3,3,4),(2.01694489302845,
2.95938268021501,3.94584357362001,4.93230446702501,5.91876536043002,6.90522625383501,
7.59274844815666),.UNSPECIFIED.);
#1050=B_SPLINE_CURVE_WITH_KNOTS('',3,(#57377,#57378,#57379,#57380,#57381,
#57382,#57383,#57384),.UNSPECIFIED.,.F.,.F.,(4,1,1,1,1,4),(59.6902604182061,
60.1955726391529,61.1820335325579,62.1684944259629,63.154955319368,64.141416212773),
 .UNSPECIFIED.);
#1051=B_SPLINE_CURVE_WITH_KNOTS('',3,(#57387,#57388,#57389,#57390,#57391,
#57392,#57393,#57394,#57395),.UNSPECIFIED.,.F.,.F.,(4,1,1,1,1,1,4),(59.6902604182061,
59.775601223602,60.762062117007,61.748523010412,62.734983903817,63.721444797222,
64.6638825844085),.UNSPECIFIED.);
#1052=B_SPLINE_CURVE_WITH_KNOTS('',3,(#57400,#57401,#57402,#57403,#57404,
#57405,#57406,#57407,#57408,#57409),.UNSPECIFIED.,.F.,.F.,(4,1,1,1,1,1,
1,4),(53.4070751110265,54.2768072787229,55.2632681721279,56.2497290655329,
57.2361899589379,58.2226508523429,59.2091117457479,59.6902604182061),
 .UNSPECIFIED.);
#1053=B_SPLINE_CURVE_WITH_KNOTS('',3,(#57410,#57411,#57412,#57413,#57414,
#57415,#57416,#57417,#57418,#57419),.UNSPECIFIED.,.F.,.F.,(4,1,1,1,1,1,
1,4),(53.4070751110265,53.856835863172,54.843296756577,55.829757649982,
56.816218543387,57.802679436792,58.789140330197,59.6902604182061),
 .UNSPECIFIED.);
#1054=B_SPLINE_CURVE_WITH_KNOTS('',3,(#57424,#57425,#57426,#57427,#57428,
#57429,#57430,#57431,#57432,#57433,#57434),.UNSPECIFIED.,.F.,.F.,(4,1,1,
1,1,1,1,1,4),(47.1238898038469,47.3715810248879,48.3580419182929,49.3445028116979,
50.3309637051029,51.3174245985079,52.3038854919129,53.2903463853179,53.4070751110265),
 .UNSPECIFIED.);
#1055=B_SPLINE_CURVE_WITH_KNOTS('',3,(#57435,#57436,#57437,#57438,#57439,
#57440,#57441,#57442,#57443,#57444),.UNSPECIFIED.,.F.,.F.,(4,1,1,1,1,1,
1,4),(47.1238898038469,47.9380705027419,48.9245313961469,49.9109922895519,
50.897453182957,51.883914076362,52.870374969767,53.4070751110265),
 .UNSPECIFIED.);
#1056=B_SPLINE_CURVE_WITH_KNOTS('',3,(#57449,#57450,#57451,#57452,#57453,
#57454,#57455,#57456,#57457,#57458),.UNSPECIFIED.,.F.,.F.,(4,1,1,1,1,1,
1,4),(40.8407044966673,41.4528156644579,42.4392765578629,43.4257374512679,
44.4121983446729,45.3986592380779,46.3851201314829,47.1238898038469),
 .UNSPECIFIED.);
#1057=B_SPLINE_CURVE_WITH_KNOTS('',3,(#57459,#57460,#57461,#57462,#57463,
#57464,#57465,#57466,#57467,#57468,#57469),.UNSPECIFIED.,.F.,.F.,(4,1,1,
1,1,1,1,1,4),(40.8407044966673,41.0328442489069,42.0193051423119,43.0057660357169,
43.9922269291219,44.9786878225269,45.9651487159319,46.9516096093369,47.1238898038469),
 .UNSPECIFIED.);
#1058=B_SPLINE_CURVE_WITH_KNOTS('',3,(#57474,#57475,#57476,#57477,#57478,
#57479,#57480,#57481,#57482,#57483),.UNSPECIFIED.,.F.,.F.,(4,1,1,1,1,1,
1,4),(34.5575191894877,35.5340503040279,36.5205111974329,37.5069720908379,
38.4934329842429,39.4798938776479,40.4663547710529,40.8407044966673),
 .UNSPECIFIED.);
#1059=B_SPLINE_CURVE_WITH_KNOTS('',3,(#57484,#57485,#57486,#57487,#57488,
#57489,#57490,#57491,#57492,#57493),.UNSPECIFIED.,.F.,.F.,(4,1,1,1,1,1,
1,4),(34.5575191894877,35.1140788884769,36.1005397818819,37.0870006752869,
38.0734615686919,39.0599224620969,40.0463833555019,40.8407044966673),
 .UNSPECIFIED.);
#1060=B_SPLINE_CURVE_WITH_KNOTS('',3,(#57498,#57499,#57500,#57501,#57502,
#57503,#57504,#57505,#57506,#57507,#57508),.UNSPECIFIED.,.F.,.F.,(4,1,1,
1,1,1,1,1,4),(28.2743338823081,28.6288240501929,29.6152849435979,30.6017458370029,
31.5882067304079,32.5746676238129,33.5611285172179,34.5475894106229,34.5575191894877),
 .UNSPECIFIED.);
#1061=B_SPLINE_CURVE_WITH_KNOTS('',3,(#57509,#57510,#57511,#57512,#57513,
#57514,#57515,#57516,#57517,#57518),.UNSPECIFIED.,.F.,.F.,(4,1,1,1,1,1,
1,4),(28.2743338823081,29.1953135280469,30.1817744214519,31.1682353148569,
32.1546962082619,33.1411571016669,34.1276179950719,34.5575191894877),
 .UNSPECIFIED.);
#1062=B_SPLINE_CURVE_WITH_KNOTS('',3,(#57523,#57524,#57525,#57526,#57527,
#57528,#57529,#57530,#57531,#57532),.UNSPECIFIED.,.F.,.F.,(4,1,1,1,1,1,
1,4),(21.9911485751285,22.7100586897628,23.6965195831678,24.6829804765729,
25.6694413699779,26.6559022633829,27.6423631567879,28.2743338823081),
 .UNSPECIFIED.);
#1063=B_SPLINE_CURVE_WITH_KNOTS('',3,(#57533,#57534,#57535,#57536,#57537,
#57538,#57539,#57540,#57541,#57542,#57543),.UNSPECIFIED.,.F.,.F.,(4,1,1,
1,1,1,1,1,4),(21.9911485751285,22.2900872742119,23.2765481676169,24.2630090610219,
25.2494699544269,26.2359308478319,27.2223917412369,28.2088526346419,28.2743338823081),
 .UNSPECIFIED.);
#1064=B_SPLINE_CURVE_WITH_KNOTS('',3,(#57549,#57550,#57551,#57552,#57553),
 .UNSPECIFIED.,.F.,.F.,(4,1,4),(14.3984001269719,15.3848610203769,15.7079632679489),
 .UNSPECIFIED.);
#1065=B_SPLINE_CURVE_WITH_KNOTS('',3,(#57556,#57557,#57558,#57559,#57560),
 .UNSPECIFIED.,.F.,.F.,(4,1,4),(13.8759337553363,14.8183715425228,15.7079632679489),
 .UNSPECIFIED.);
#1066=B_SPLINE_CURVE_WITH_KNOTS('',3,(#57566,#57567,#57568,#57569),
 .UNSPECIFIED.,.F.,.F.,(4,4),(51.5750455984138,52.2824273504651),
 .UNSPECIFIED.);
#1067=B_SPLINE_CURVE_WITH_KNOTS('',3,(#57577,#57578,#57579,#57580,#57581,
#57582,#57583,#57584,#57585,#57586),.UNSPECIFIED.,.F.,.F.,(4,3,3,4),(-50.2654824574367,
-49.3230446702501,-48.3365837768451,-47.8312715558982),.UNSPECIFIED.);
#1068=B_SPLINE_CURVE_WITH_KNOTS('',3,(#57591,#57592,#57593,#57594,#57595,
#57596,#57597,#57598,#57599,#57600,#57601,#57602,#57603,#57604,#57605,#57606,
#57607,#57608,#57609,#57610,#57611,#57612,#57613,#57614,#57615),
 .UNSPECIFIED.,.F.,.F.,(4,3,3,3,3,3,3,3,4),(45.2918602912342,45.3772010966301,
46.3636619900351,47.3501228834401,48.3365837768451,49.3230446702501,50.3095055636551,
51.2959664570601,51.5750455984138),.UNSPECIFIED.);
#1069=B_SPLINE_CURVE_WITH_KNOTS('',3,(#57616,#57617,#57618,#57619,#57620,
#57621,#57622,#57623,#57624,#57625,#57626,#57627,#57628,#57629,#57630,#57631,
#57632,#57633,#57634,#57635,#57636,#57637),.UNSPECIFIED.,.F.,.F.,(4,3,3,
3,3,3,3,4),(-47.8312715558982,-47.3501228834401,-46.3636619900351,-45.3772010966301,
-44.3907402032251,-43.4042793098201,-42.4178184164151,-41.5480862487186),
 .UNSPECIFIED.);
#1070=B_SPLINE_CURVE_WITH_KNOTS('',3,(#57642,#57643,#57644,#57645,#57646,
#57647,#57648,#57649,#57650,#57651,#57652,#57653,#57654,#57655,#57656,#57657,
#57658,#57659,#57660,#57661,#57662,#57663),.UNSPECIFIED.,.F.,.F.,(4,3,3,
3,3,3,3,4),(39.0086749840546,39.4584357362001,40.4448966296051,41.4313575230101,
42.4178184164151,43.4042793098201,44.3907402032251,45.2918602912342),
 .UNSPECIFIED.);
#1071=B_SPLINE_CURVE_WITH_KNOTS('',3,(#57664,#57665,#57666,#57667,#57668,
#57669,#57670,#57671,#57672,#57673,#57674,#57675,#57676,#57677,#57678,#57679,
#57680,#57681,#57682,#57683,#57684,#57685,#57686,#57687,#57688),
 .UNSPECIFIED.,.F.,.F.,(4,3,3,3,3,3,3,3,4),(-41.5480862487186,-41.4313575230101,
-40.4448966296051,-39.4584357362001,-38.4719748427951,-37.4855139493901,
-36.4990530559851,-35.5125921625801,-35.264900941539),.UNSPECIFIED.);
#1072=B_SPLINE_CURVE_WITH_KNOTS('',3,(#57693,#57694,#57695,#57696,#57697,
#57698,#57699,#57700,#57701,#57702,#57703,#57704,#57705,#57706,#57707,#57708,
#57709,#57710,#57711,#57712,#57713,#57714),.UNSPECIFIED.,.F.,.F.,(4,3,3,
3,3,3,3,4),(32.725489676875,33.5396703757701,34.5261312691751,35.5125921625801,
36.4990530559851,37.4855139493901,38.4719748427951,39.0086749840546),
 .UNSPECIFIED.);
#1073=B_SPLINE_CURVE_WITH_KNOTS('',3,(#57715,#57716,#57717,#57718,#57719,
#57720,#57721,#57722,#57723,#57724,#57725,#57726,#57727,#57728,#57729,#57730,
#57731,#57732,#57733,#57734,#57735,#57736),.UNSPECIFIED.,.F.,.F.,(4,3,3,
3,3,3,3,4),(-35.264900941539,-34.5261312691751,-33.5396703757701,-32.5532094823651,
-31.5667485889601,-30.5802876955551,-29.5938268021501,-28.9817156343595),
 .UNSPECIFIED.);
#1074=B_SPLINE_CURVE_WITH_KNOTS('',3,(#57741,#57742,#57743,#57744,#57745,
#57746,#57747,#57748,#57749,#57750,#57751,#57752,#57753,#57754,#57755,#57756,
#57757,#57758,#57759,#57760,#57761,#57762,#57763,#57764,#57765),
 .UNSPECIFIED.,.F.,.F.,(4,3,3,3,3,3,3,3,4),(26.4423043696954,26.6344441219351,
27.6209050153401,28.6073659087451,29.5938268021501,30.5802876955551,31.5667485889601,
32.5532094823651,32.725489676875),.UNSPECIFIED.);
#1075=B_SPLINE_CURVE_WITH_KNOTS('',3,(#57766,#57767,#57768,#57769,#57770,
#57771,#57772,#57773,#57774,#57775,#57776,#57777,#57778,#57779,#57780,#57781,
#57782,#57783,#57784,#57785,#57786,#57787),.UNSPECIFIED.,.F.,.F.,(4,3,3,
3,3,3,3,4),(-28.9817156343595,-28.6073659087451,-27.6209050153401,-26.6344441219351,
-25.6479832285301,-24.6615223351251,-23.6750614417201,-22.6985303271799),
 .UNSPECIFIED.);
#1076=B_SPLINE_CURVE_WITH_KNOTS('',3,(#57792,#57793,#57794,#57795,#57796,
#57797,#57798,#57799,#57800,#57801,#57802,#57803,#57804,#57805,#57806,#57807,
#57808,#57809,#57810,#57811,#57812,#57813),.UNSPECIFIED.,.F.,.F.,(4,3,3,
3,3,3,3,4),(20.1591190625158,20.7156787615051,21.7021396549101,22.6886005483151,
23.6750614417201,24.6615223351251,25.6479832285301,26.4423043696954),
 .UNSPECIFIED.);
#1077=B_SPLINE_CURVE_WITH_KNOTS('',3,(#57814,#57815,#57816,#57817,#57818,
#57819,#57820,#57821,#57822,#57823,#57824,#57825,#57826,#57827,#57828,#57829,
#57830,#57831,#57832,#57833,#57834,#57835,#57836,#57837,#57838),
 .UNSPECIFIED.,.F.,.F.,(4,3,3,3,3,3,3,3,4),(-22.6985303271799,-22.6886005483151,
-21.7021396549101,-20.7156787615051,-19.7292178681001,-18.7427569746951,
-17.75629608129,-16.769835187885,-16.4153450200003),.UNSPECIFIED.);
#1078=B_SPLINE_CURVE_WITH_KNOTS('',3,(#57843,#57844,#57845,#57846,#57847,
#57848,#57849,#57850,#57851,#57852,#57853,#57854,#57855,#57856,#57857,#57858,
#57859,#57860,#57861,#57862,#57863,#57864),.UNSPECIFIED.,.F.,.F.,(4,3,3,
3,3,3,3,4),(13.8759337553362,14.796913401075,15.78337429448,16.769835187885,
17.75629608129,18.7427569746951,19.7292178681001,20.1591190625158),
 .UNSPECIFIED.);
#1079=B_SPLINE_CURVE_WITH_KNOTS('',3,(#57865,#57866,#57867,#57868,#57869,
#57870,#57871,#57872,#57873,#57874,#57875,#57876,#57877,#57878,#57879,#57880,
#57881,#57882,#57883,#57884,#57885,#57886),.UNSPECIFIED.,.F.,.F.,(4,3,3,
3,3,3,3,4),(-16.4153450200003,-15.78337429448,-14.796913401075,-13.81045250767,
-12.823991614265,-11.83753072086,-10.851069827455,-10.1321597128207),
 .UNSPECIFIED.);
#1080=B_SPLINE_CURVE_WITH_KNOTS('',3,(#57892,#57893,#57894,#57895,#57896,
#57897,#57898,#57899,#57900,#57901,#57902,#57903,#57904),.UNSPECIFIED.,
 .F.,.F.,(4,3,3,3,4),(-3.84897440564112,-2.95938268021501,-1.97292178681001,
-0.986460893405003,0.),.UNSPECIFIED.);
#1081=B_SPLINE_CURVE_WITH_KNOTS('',3,(#57907,#57908,#57909,#57910,#57911,
#57912,#57913,#57914,#57915,#57916,#57917,#57918,#57919,#57920,#57921,#57922,
#57923,#57924,#57925),.UNSPECIFIED.,.F.,.F.,(4,3,3,3,3,3,4),(2.01694489302844,
2.95938268021501,3.94584357362001,4.93230446702501,5.91876536043001,6.90522625383502,
7.59274844815664),.UNSPECIFIED.);
#1082=B_SPLINE_CURVE_WITH_KNOTS('',3,(#57931,#57932,#57933,#57934,#57935,
#57936,#57937,#57938),.UNSPECIFIED.,.F.,.F.,(4,1,1,1,1,4),(59.6902604182061,
60.195572639153,61.182033532558,62.168494425963,63.154955319368,64.141416212773),
 .UNSPECIFIED.);
#1083=B_SPLINE_CURVE_WITH_KNOTS('',3,(#57941,#57942,#57943,#57944,#57945,
#57946,#57947,#57948,#57949),.UNSPECIFIED.,.F.,.F.,(4,1,1,1,1,1,4),(59.6902604182061,
59.775601223602,60.762062117007,61.748523010412,62.734983903817,63.721444797222,
64.6638825844085),.UNSPECIFIED.);
#1084=B_SPLINE_CURVE_WITH_KNOTS('',3,(#57954,#57955,#57956,#57957,#57958,
#57959,#57960,#57961,#57962,#57963),.UNSPECIFIED.,.F.,.F.,(4,1,1,1,1,1,
1,4),(53.4070751110265,54.2768072787229,55.2632681721279,56.2497290655329,
57.2361899589379,58.222650852343,59.209111745748,59.6902604182061),
 .UNSPECIFIED.);
#1085=B_SPLINE_CURVE_WITH_KNOTS('',3,(#57964,#57965,#57966,#57967,#57968,
#57969,#57970,#57971,#57972,#57973),.UNSPECIFIED.,.F.,.F.,(4,1,1,1,1,1,
1,4),(53.4070751110265,53.856835863172,54.843296756577,55.829757649982,
56.816218543387,57.802679436792,58.789140330197,59.6902604182061),
 .UNSPECIFIED.);
#1086=B_SPLINE_CURVE_WITH_KNOTS('',3,(#57978,#57979,#57980,#57981,#57982,
#57983,#57984,#57985,#57986,#57987,#57988),.UNSPECIFIED.,.F.,.F.,(4,1,1,
1,1,1,1,1,4),(47.1238898038469,47.3715810248879,48.3580419182929,49.3445028116979,
50.3309637051029,51.3174245985079,52.3038854919129,53.2903463853179,53.4070751110265),
 .UNSPECIFIED.);
#1087=B_SPLINE_CURVE_WITH_KNOTS('',3,(#57989,#57990,#57991,#57992,#57993,
#57994,#57995,#57996,#57997,#57998),.UNSPECIFIED.,.F.,.F.,(4,1,1,1,1,1,
1,4),(47.1238898038469,47.938070502742,48.924531396147,49.910992289552,
50.897453182957,51.883914076362,52.870374969767,53.4070751110265),
 .UNSPECIFIED.);
#1088=B_SPLINE_CURVE_WITH_KNOTS('',3,(#58003,#58004,#58005,#58006,#58007,
#58008,#58009,#58010,#58011,#58012),.UNSPECIFIED.,.F.,.F.,(4,1,1,1,1,1,
1,4),(40.8407044966673,41.4528156644579,42.4392765578629,43.4257374512679,
44.4121983446729,45.3986592380779,46.3851201314829,47.1238898038469),
 .UNSPECIFIED.);
#1089=B_SPLINE_CURVE_WITH_KNOTS('',3,(#58013,#58014,#58015,#58016,#58017,
#58018,#58019,#58020,#58021,#58022,#58023),.UNSPECIFIED.,.F.,.F.,(4,1,1,
1,1,1,1,1,4),(40.8407044966673,41.0328442489069,42.0193051423119,43.0057660357169,
43.9922269291219,44.978687822527,45.965148715932,46.951609609337,47.1238898038469),
 .UNSPECIFIED.);
#1090=B_SPLINE_CURVE_WITH_KNOTS('',3,(#58028,#58029,#58030,#58031,#58032,
#58033,#58034,#58035,#58036,#58037),.UNSPECIFIED.,.F.,.F.,(4,1,1,1,1,1,
1,4),(34.5575191894877,35.5340503040279,36.5205111974329,37.5069720908379,
38.4934329842429,39.4798938776479,40.4663547710529,40.8407044966673),
 .UNSPECIFIED.);
#1091=B_SPLINE_CURVE_WITH_KNOTS('',3,(#58038,#58039,#58040,#58041,#58042,
#58043,#58044,#58045,#58046,#58047),.UNSPECIFIED.,.F.,.F.,(4,1,1,1,1,1,
1,4),(34.5575191894877,35.1140788884769,36.1005397818819,37.0870006752869,
38.0734615686919,39.0599224620969,40.0463833555019,40.8407044966673),
 .UNSPECIFIED.);
#1092=B_SPLINE_CURVE_WITH_KNOTS('',3,(#58052,#58053,#58054,#58055,#58056,
#58057,#58058,#58059,#58060,#58061,#58062),.UNSPECIFIED.,.F.,.F.,(4,1,1,
1,1,1,1,1,4),(28.2743338823081,28.6288240501929,29.6152849435979,30.6017458370029,
31.5882067304079,32.5746676238129,33.5611285172179,34.5475894106229,34.5575191894877),
 .UNSPECIFIED.);
#1093=B_SPLINE_CURVE_WITH_KNOTS('',3,(#58063,#58064,#58065,#58066,#58067,
#58068,#58069,#58070,#58071,#58072),.UNSPECIFIED.,.F.,.F.,(4,1,1,1,1,1,
1,4),(28.2743338823081,29.1953135280469,30.1817744214519,31.1682353148569,
32.1546962082619,33.1411571016669,34.1276179950719,34.5575191894877),
 .UNSPECIFIED.);
#1094=B_SPLINE_CURVE_WITH_KNOTS('',3,(#58077,#58078,#58079,#58080,#58081,
#58082,#58083,#58084,#58085,#58086),.UNSPECIFIED.,.F.,.F.,(4,1,1,1,1,1,
1,4),(21.9911485751285,22.7100586897629,23.6965195831679,24.6829804765729,
25.6694413699779,26.6559022633829,27.6423631567879,28.2743338823081),
 .UNSPECIFIED.);
#1095=B_SPLINE_CURVE_WITH_KNOTS('',3,(#58087,#58088,#58089,#58090,#58091,
#58092,#58093,#58094,#58095,#58096,#58097),.UNSPECIFIED.,.F.,.F.,(4,1,1,
1,1,1,1,1,4),(21.9911485751285,22.2900872742119,23.2765481676169,24.2630090610219,
25.2494699544269,26.2359308478319,27.2223917412369,28.2088526346419,28.2743338823081),
 .UNSPECIFIED.);
#1096=B_SPLINE_CURVE_WITH_KNOTS('',3,(#58103,#58104,#58105,#58106,#58107),
 .UNSPECIFIED.,.F.,.F.,(4,1,4),(14.3984001269719,15.3848610203769,15.7079632679489),
 .UNSPECIFIED.);
#1097=B_SPLINE_CURVE_WITH_KNOTS('',3,(#58110,#58111,#58112,#58113,#58114),
 .UNSPECIFIED.,.F.,.F.,(4,1,4),(13.8759337553363,14.8183715425228,15.7079632679489),
 .UNSPECIFIED.);
#1098=B_SPLINE_CURVE_WITH_KNOTS('',3,(#58116,#58117,#58118,#58119,#58120,
#58121,#58122,#58123,#58124,#58125,#58126,#58127,#58128,#58129,#58130,#58131,
#58132,#58133,#58134,#58135,#58136,#58137,#58138,#58139,#58140,#58141,#58142,
#58143,#58144,#58145,#58146,#58147,#58148,#58149,#58150,#58151,#58152,#58153,
#58154,#58155,#58156,#58157,#58158,#58159,#58160,#58161,#58162,#58163,#58164,
#58165,#58166,#58167,#58168,#58169,#58170,#58171,#58172,#58173,#58174,#58175,
#58176,#58177,#58178,#58179,#58180,#58181,#58182,#58183,#58184,#58185,#58186,
#58187,#58188,#58189,#58190,#58191,#58192,#58193,#58194,#58195,#58196,#58197,
#58198,#58199,#58200,#58201,#58202,#58203,#58204,#58205,#58206,#58207,#58208,
#58209),.UNSPECIFIED.,.F.,.F.,(4,3,3,3,3,3,3,3,3,3,3,3,3,3,3,3,3,3,3,3,
3,3,3,3,3,3,3,3,3,3,3,4),(-0.569248610399439,-0.54356321026788,-0.51725177755219,
-0.510354554433286,-0.504796969238609,-0.477731405971173,-0.456105549235436,
-0.448989007169752,-0.44252634525638,-0.41479354371395,-0.386635764628684,
-0.358697147124577,-0.345203998364752,-0.340863871144016,-0.336326749475397,
-0.307401033120815,-0.304724552085278,-0.27693747898326,-0.248513803621531,
-0.232656005969356,-0.228221175977861,-0.199230005786307,-0.169667310992576,
-0.139872005633123,-0.124084622535551,-0.117720237608985,-0.113355273030534,
-0.0828138353231538,-0.052246421283799,-0.0222710285652406,-0.0135729408525455,
0.),.UNSPECIFIED.);
#1099=B_SPLINE_CURVE_WITH_KNOTS('',3,(#58210,#58211,#58212,#58213,#58214,
#58215,#58216,#58217,#58218,#58219,#58220,#58221,#58222,#58223,#58224,#58225,
#58226,#58227,#58228,#58229,#58230,#58231,#58232,#58233,#58234,#58235,#58236,
#58237,#58238,#58239,#58240,#58241,#58242,#58243,#58244,#58245,#58246,#58247,
#58248,#58249,#58250,#58251,#58252,#58253,#58254,#58255,#58256,#58257,#58258,
#58259,#58260,#58261,#58262,#58263,#58264,#58265,#58266,#58267,#58268,#58269,
#58270,#58271,#58272,#58273,#58274,#58275,#58276,#58277,#58278,#58279,#58280,
#58281,#58282,#58283,#58284,#58285,#58286,#58287,#58288,#58289,#58290,#58291,
#58292,#58293,#58294,#58295,#58296,#58297,#58298,#58299,#58300,#58301,#58302,
#58303,#58304,#58305,#58306),.UNSPECIFIED.,.F.,.F.,(4,3,3,3,3,3,3,3,3,3,
3,3,3,3,3,3,3,3,3,3,3,3,3,3,3,3,3,3,3,3,3,3,4),(-0.566847306048084,-0.536659061903649,
-0.506054167513983,-0.49735931415594,-0.490469774907708,-0.46032717525434,
-0.437299554635119,-0.425273742105126,-0.42037664994689,-0.390957260822939,
-0.362078927205336,-0.333750616169337,-0.319339514702147,-0.312267662800037,
-0.308232039095118,-0.280241121737425,-0.276106210300576,-0.247648675773662,
-0.218090819684273,-0.209492296602851,-0.204738459070877,-0.200614645085577,
-0.172781389578512,-0.145026433045361,-0.117750656382618,-0.10443005271711,
-0.100025234036307,-0.0958388284225397,-0.0691738510173895,-0.0429555684736812,
-0.0175134533592336,-0.0111858270585534,0.),.UNSPECIFIED.);
#1100=B_SPLINE_CURVE_WITH_KNOTS('',3,(#58308,#58309,#58310,#58311,#58312,
#58313,#58314,#58315,#58316,#58317,#58318),.UNSPECIFIED.,.F.,.F.,(4,1,1,
1,1,1,1,1,4),(15.7079632679489,15.8048324359278,16.7912933293328,17.7777542227378,
18.7642151161429,19.7506760095479,20.7371369029529,21.7235977963579,21.9911485751285),
 .UNSPECIFIED.);
#1101=B_SPLINE_CURVE_WITH_KNOTS('',3,(#58319,#58320,#58321,#58322,#58323,
#58324,#58325,#58326,#58327,#58328),.UNSPECIFIED.,.F.,.F.,(4,1,1,1,1,1,
1,4),(15.7079632679489,16.3713219137819,17.3577828071869,18.3442437005919,
19.3307045939969,20.3171654874019,21.3036263808069,21.9911485751285),
 .UNSPECIFIED.);
#1102=B_SPLINE_CURVE_WITH_KNOTS('',3,(#58553,#58554,#58555,#58556,#58557,
#58558,#58559,#58560,#58561,#58562,#58563,#58564,#58565,#58566,#58567,#58568,
#58569,#58570,#58571,#58572,#58573,#58574,#58575,#58576,#58577,#58578,#58579,
#58580,#58581,#58582,#58583,#58584,#58585,#58586,#58587,#58588,#58589,#58590,
#58591,#58592,#58593,#58594,#58595,#58596,#58597,#58598,#58599,#58600,#58601,
#58602,#58603,#58604,#58605,#58606,#58607,#58608,#58609,#58610,#58611,#58612,
#58613,#58614,#58615,#58616,#58617,#58618,#58619,#58620,#58621,#58622,#58623,
#58624,#58625,#58626,#58627,#58628,#58629,#58630,#58631,#58632,#58633,#58634,
#58635,#58636,#58637,#58638,#58639,#58640,#58641,#58642,#58643),
 .UNSPECIFIED.,.F.,.F.,(4,3,3,3,3,3,3,3,3,3,3,3,3,3,3,3,3,3,3,3,3,3,3,3,
3,3,3,3,3,3,4),(0.,0.0253749761808373,0.0514202453857712,0.0779566483534038,
0.0899762183904566,0.0968038784409555,0.102648429733812,0.129953030321501,
0.157704740391969,0.184206422575685,0.195897654370316,0.20134852299372,
0.206600979641336,0.235231099301492,0.263711469126832,0.291580654157613,
0.307940063613124,0.312151264914525,0.340175958120619,0.369258857874792,
0.398694885878799,0.418024425824675,0.423205607838508,0.428149011920458,
0.459444560301794,0.482916221587795,0.491343691753009,0.498388187388185,
0.528903379110968,0.553331205445801,0.566847306048077),.UNSPECIFIED.);
#1103=B_SPLINE_CURVE_WITH_KNOTS('',3,(#58644,#58645,#58646,#58647,#58648,
#58649,#58650,#58651,#58652,#58653,#58654,#58655,#58656,#58657,#58658,#58659,
#58660,#58661,#58662,#58663,#58664,#58665,#58666,#58667,#58668),
 .UNSPECIFIED.,.F.,.F.,(4,3,3,3,3,3,3,3,4),(-10.1321597128207,-9.86460893405003,
-8.87814804064503,-7.89168714724002,-6.90522625383502,-5.91876536043002,
-4.93230446702501,-3.94584357362001,-3.84897440564112),.UNSPECIFIED.);
#1104=B_SPLINE_CURVE_WITH_KNOTS('',3,(#58893,#58894,#58895,#58896,#58897,
#58898,#58899,#58900,#58901,#58902,#58903,#58904,#58905,#58906,#58907,#58908,
#58909,#58910,#58911,#58912,#58913,#58914,#58915,#58916,#58917),
 .UNSPECIFIED.,.F.,.F.,(4,3,3,3,3,3,3,3,4),(7.59274844815664,7.89168714724002,
8.87814804064502,9.86460893405003,10.851069827455,11.83753072086,12.823991614265,
13.81045250767,13.8759337553362),.UNSPECIFIED.);
#1105=B_SPLINE_CURVE_WITH_KNOTS('',3,(#58918,#58919,#58920,#58921,#58922,
#58923,#58924,#58925,#58926,#58927,#58928,#58929,#58930,#58931,#58932,#58933,
#58934,#58935,#58936,#58937,#58938,#58939,#58940,#58941,#58942,#58943,#58944,
#58945,#58946,#58947,#58948,#58949,#58950,#58951,#58952,#58953,#58954,#58955,
#58956,#58957,#58958,#58959,#58960,#58961,#58962,#58963,#58964,#58965,#58966,
#58967,#58968,#58969,#58970,#58971,#58972,#58973,#58974,#58975,#58976,#58977,
#58978,#58979,#58980,#58981,#58982,#58983,#58984,#58985,#58986,#58987,#58988,
#58989,#58990,#58991,#58992,#58993,#58994,#58995,#58996,#58997,#58998,#58999,
#59000,#59001,#59002,#59003,#59004,#59005),.UNSPECIFIED.,.F.,.F.,(4,3,3,
3,3,3,3,3,3,3,3,3,3,3,3,3,3,3,3,3,3,3,3,3,3,3,3,3,3,4),(0.,0.0297343552567438,
0.0601207256243431,0.0891402780188099,0.114532386363968,0.120626668225237,
0.150381699187288,0.179970351010139,0.208047049452624,0.230390915983779,
0.234467415790057,0.263372280285067,0.292277144780078,0.321216399233671,
0.336017014192979,0.340284510578769,0.344592048040137,0.372696731227283,
0.400818676768978,0.428516493390579,0.439577089903316,0.445404908685826,
0.450327814198675,0.477288785913009,0.497473149080406,0.505236433644848,
0.511959475796908,0.537908351627998,0.558026238582596,0.569248610399449),
 .UNSPECIFIED.);
#1106=B_SPLINE_CURVE_WITH_KNOTS('',3,(#59008,#59009,#59010,#59011,#59012,
#59013,#59014,#59015,#59016,#59017,#59018,#59019,#59020,#59021,#59022,#59023,
#59024,#59025,#59026,#59027,#59028,#59029,#59030,#59031,#59032,#59033,#59034,
#59035,#59036,#59037,#59038,#59039,#59040,#59041,#59042,#59043,#59044,#59045,
#59046,#59047,#59048,#59049,#59050,#59051,#59052,#59053,#59054,#59055,#59056,
#59057,#59058,#59059,#59060,#59061,#59062,#59063,#59064,#59065,#59066,#59067,
#59068,#59069,#59070,#59071,#59072,#59073,#59074,#59075,#59076,#59077,#59078,
#59079,#59080,#59081,#59082,#59083,#59084,#59085,#59086,#59087,#59088,#59089,
#59090,#59091,#59092,#59093,#59094,#59095,#59096,#59097,#59098,#59099,#59100,
#59101),.UNSPECIFIED.,.F.,.F.,(4,3,3,3,3,3,3,3,3,3,3,3,3,3,3,3,3,3,3,3,
3,3,3,3,3,3,3,3,3,3,3,4),(-0.569248610399449,-0.543563182261633,-0.517251726319563,
-0.510354426439678,-0.50479695498386,-0.477731372271303,-0.456105519748053,
-0.448988869091777,-0.442526350881559,-0.414793531524841,-0.386635753667763,
-0.358697146614525,-0.34520399798222,-0.340863870845798,-0.33632674866549,
-0.307401034118885,-0.304724552085303,-0.276937498904782,-0.248513836066906,
-0.232656079580101,-0.228221193819419,-0.199230039362694,-0.1696673522492,
-0.139872047864531,-0.124084659488033,-0.117720027272243,-0.113355233265148,
-0.0828137979174933,-0.0522463837565239,-0.0222709947806455,-0.0135729408525504,
0.),.UNSPECIFIED.);
#1107=B_SPLINE_CURVE_WITH_KNOTS('',3,(#59102,#59103,#59104,#59105,#59106,
#59107,#59108,#59109,#59110,#59111,#59112,#59113,#59114,#59115,#59116,#59117,
#59118,#59119,#59120,#59121,#59122,#59123,#59124,#59125,#59126,#59127,#59128,
#59129,#59130,#59131,#59132,#59133,#59134,#59135,#59136,#59137,#59138,#59139,
#59140,#59141,#59142,#59143,#59144,#59145,#59146,#59147,#59148,#59149,#59150,
#59151,#59152,#59153,#59154,#59155,#59156,#59157,#59158,#59159,#59160,#59161,
#59162,#59163,#59164,#59165,#59166,#59167,#59168,#59169,#59170,#59171,#59172,
#59173,#59174,#59175,#59176,#59177,#59178,#59179,#59180,#59181,#59182,#59183,
#59184,#59185,#59186,#59187,#59188,#59189,#59190,#59191,#59192,#59193,#59194,
#59195,#59196,#59197,#59198),.UNSPECIFIED.,.F.,.F.,(4,3,3,3,3,3,3,3,3,3,
3,3,3,3,3,3,3,3,3,3,3,3,3,3,3,3,3,3,3,3,3,3,4),(-0.566847306048093,-0.536659041927388,
-0.506054142756331,-0.497359284644658,-0.490469768799004,-0.460327170439997,
-0.43729955042257,-0.425273732599625,-0.420376646332479,-0.390957260247852,
-0.362078935948881,-0.333750632250775,-0.319339526763226,-0.312267682102884,
-0.308232073167884,-0.280241164390834,-0.276106210300581,-0.247648676940529,
-0.218090820705282,-0.209492305755956,-0.204738428044034,-0.200614618605046,
-0.172781361973988,-0.145026407762726,-0.11775064123255,-0.1044300394608,
-0.100025210256123,-0.0958388268874492,-0.0691738559200647,-0.0429555864020897,
-0.0175134923892686,-0.011185827058555,0.),.UNSPECIFIED.);
#1108=B_SPLINE_CURVE_WITH_KNOTS('',3,(#59200,#59201,#59202,#59203,#59204,
#59205,#59206,#59207,#59208,#59209,#59210),.UNSPECIFIED.,.F.,.F.,(4,1,1,
1,1,1,1,1,4),(15.7079632679489,15.8048324359278,16.7912933293328,17.7777542227378,
18.7642151161428,19.7506760095478,20.7371369029528,21.7235977963578,21.9911485751285),
 .UNSPECIFIED.);
#1109=B_SPLINE_CURVE_WITH_KNOTS('',3,(#59211,#59212,#59213,#59214,#59215,
#59216,#59217,#59218,#59219,#59220),.UNSPECIFIED.,.F.,.F.,(4,1,1,1,1,1,
1,4),(15.7079632679489,16.3713219137819,17.3577828071869,18.3442437005919,
19.3307045939969,20.3171654874019,21.3036263808069,21.9911485751285),
 .UNSPECIFIED.);
#1110=B_SPLINE_CURVE_WITH_KNOTS('',3,(#59445,#59446,#59447,#59448,#59449,
#59450,#59451,#59452,#59453,#59454,#59455,#59456,#59457,#59458,#59459,#59460,
#59461,#59462,#59463,#59464,#59465,#59466,#59467,#59468,#59469,#59470,#59471,
#59472,#59473,#59474,#59475,#59476,#59477,#59478,#59479,#59480,#59481,#59482,
#59483,#59484,#59485,#59486,#59487,#59488,#59489,#59490,#59491,#59492,#59493,
#59494,#59495,#59496,#59497,#59498,#59499,#59500,#59501,#59502,#59503,#59504,
#59505,#59506,#59507,#59508,#59509,#59510,#59511,#59512,#59513,#59514,#59515,
#59516,#59517,#59518,#59519,#59520,#59521,#59522,#59523,#59524,#59525,#59526,
#59527,#59528,#59529,#59530,#59531,#59532,#59533,#59534,#59535),
 .UNSPECIFIED.,.F.,.F.,(4,3,3,3,3,3,3,3,3,3,3,3,3,3,3,3,3,3,3,3,3,3,3,3,
3,3,3,3,3,3,4),(0.,0.0253750087516075,0.0514203072172438,0.0779567024559424,
0.0899762332180016,0.0968038780381036,0.10264843024679,0.129953053284425,
0.157704773943122,0.18420644773905,0.195897666391424,0.201348497446843,
0.206600974226724,0.235231090538335,0.263711469126833,0.291580637154729,
0.307940047672921,0.312151253621455,0.340175922185425,0.369258810210864,
0.398694834915773,0.418024381232026,0.42320553295956,0.428148997028943,
0.459444549133158,0.482916213211318,0.491343671374895,0.498388182075807,
0.528903373982295,0.5533312054458,0.566847306048075),.UNSPECIFIED.);
#1111=B_SPLINE_CURVE_WITH_KNOTS('',3,(#59536,#59537,#59538,#59539,#59540,
#59541,#59542,#59543,#59544,#59545,#59546,#59547,#59548,#59549,#59550,#59551,
#59552,#59553,#59554,#59555,#59556,#59557,#59558,#59559,#59560),
 .UNSPECIFIED.,.F.,.F.,(4,3,3,3,3,3,3,3,4),(-10.1321597128207,-9.86460893405002,
-8.87814804064502,-7.89168714724002,-6.90522625383502,-5.91876536043002,
-4.93230446702501,-3.94584357362001,-3.84897440564113),.UNSPECIFIED.);
#1112=B_SPLINE_CURVE_WITH_KNOTS('',3,(#59785,#59786,#59787,#59788,#59789,
#59790,#59791,#59792,#59793,#59794,#59795,#59796,#59797,#59798,#59799,#59800,
#59801,#59802,#59803,#59804,#59805,#59806,#59807,#59808,#59809),
 .UNSPECIFIED.,.F.,.F.,(4,3,3,3,3,3,3,3,4),(7.59274844815666,7.89168714724002,
8.87814804064502,9.86460893405003,10.851069827455,11.83753072086,12.823991614265,
13.81045250767,13.8759337553362),.UNSPECIFIED.);
#1113=B_SPLINE_CURVE_WITH_KNOTS('',3,(#59810,#59811,#59812,#59813,#59814,
#59815,#59816,#59817,#59818,#59819,#59820,#59821,#59822,#59823,#59824,#59825,
#59826,#59827,#59828,#59829,#59830,#59831,#59832,#59833,#59834,#59835,#59836,
#59837,#59838,#59839,#59840,#59841,#59842,#59843,#59844,#59845,#59846,#59847,
#59848,#59849,#59850,#59851,#59852,#59853,#59854,#59855,#59856,#59857,#59858,
#59859,#59860,#59861,#59862,#59863,#59864,#59865,#59866,#59867,#59868,#59869,
#59870,#59871,#59872,#59873,#59874,#59875,#59876,#59877,#59878,#59879,#59880,
#59881,#59882,#59883,#59884,#59885,#59886,#59887,#59888,#59889,#59890,#59891,
#59892,#59893,#59894,#59895,#59896,#59897),.UNSPECIFIED.,.F.,.F.,(4,3,3,
3,3,3,3,3,3,3,3,3,3,3,3,3,3,3,3,3,3,3,3,3,3,3,3,3,3,4),(0.,0.0297343797035864,
0.060120761877283,0.0891403097401323,0.114532414120125,0.120626668186271,
0.150381698992516,0.17997034368319,0.208047043957412,0.230390900373193,
0.234467387186734,0.263372265983406,0.292277144780078,0.32121640004702,
0.336017014955494,0.340284508571086,0.34459204647613,0.372696730262498,
0.400818675119593,0.428516484798209,0.439577058767134,0.445404835481582,
0.450327801888399,0.477288765031749,0.497473133419461,0.505236404100872,
0.511959471749983,0.53790833305976,0.558026238582597,0.56924861039945),
 .UNSPECIFIED.);
#1114=B_SPLINE_CURVE_WITH_KNOTS('',3,(#59900,#59901,#59902,#59903,#59904,
#59905,#59906,#59907,#59908,#59909,#59910,#59911,#59912,#59913,#59914,#59915,
#59916,#59917,#59918,#59919,#59920,#59921,#59922,#59923,#59924,#59925,#59926,
#59927,#59928,#59929,#59930,#59931,#59932,#59933,#59934,#59935,#59936,#59937,
#59938,#59939,#59940,#59941,#59942,#59943,#59944,#59945,#59946,#59947,#59948,
#59949,#59950,#59951,#59952,#59953,#59954,#59955,#59956,#59957,#59958,#59959,
#59960,#59961,#59962,#59963,#59964,#59965,#59966,#59967,#59968,#59969,#59970,
#59971,#59972,#59973,#59974,#59975,#59976,#59977,#59978,#59979,#59980,#59981,
#59982,#59983,#59984,#59985,#59986,#59987,#59988,#59989,#59990,#59991,#59992,
#59993),.UNSPECIFIED.,.F.,.F.,(4,3,3,3,3,3,3,3,3,3,3,3,3,3,3,3,3,3,3,3,
3,3,3,3,3,3,3,3,3,3,3,4),(-0.569248610399453,-0.543562558043411,-0.517250584660783,
-0.510351573265488,-0.504796629765234,-0.477730613871864,-0.456104856148543,
-0.448985761186696,-0.442526474182097,-0.414793258161359,-0.386635508597981,
-0.358697135593994,-0.34520398971682,-0.340863862860947,-0.336326730527656,
-0.307401056922635,-0.304724552085299,-0.276937944371136,-0.248514561286397,
-0.23265772508323,-0.228221590562879,-0.199230787763733,-0.169668272024871,
-0.139872989252767,-0.12408548320274,-0.117715318700335,-0.113354339820942,
-0.0828129568830819,-0.0522455401301121,-0.022270235741096,-0.0135729408525504,
0.),.UNSPECIFIED.);
#1115=B_SPLINE_CURVE_WITH_KNOTS('',3,(#59994,#59995,#59996,#59997,#59998,
#59999,#60000,#60001,#60002,#60003,#60004,#60005,#60006,#60007,#60008,#60009,
#60010,#60011,#60012,#60013,#60014,#60015,#60016,#60017,#60018,#60019,#60020,
#60021,#60022,#60023,#60024,#60025,#60026,#60027,#60028,#60029,#60030,#60031,
#60032,#60033,#60034,#60035,#60036,#60037,#60038,#60039,#60040,#60041,#60042,
#60043,#60044,#60045,#60046,#60047,#60048,#60049,#60050,#60051,#60052,#60053,
#60054,#60055,#60056,#60057,#60058,#60059,#60060,#60061,#60062,#60063,#60064,
#60065,#60066,#60067,#60068,#60069,#60070,#60071,#60072,#60073,#60074,#60075,
#60076,#60077,#60078,#60079,#60080,#60081,#60082,#60083,#60084,#60085,#60086,
#60087,#60088,#60089,#60090),.UNSPECIFIED.,.F.,.F.,(4,3,3,3,3,3,3,3,3,3,
3,3,3,3,3,3,3,3,3,3,3,3,3,3,3,3,3,3,3,3,3,3,4),(-0.566847306048093,-0.536658716403432,
-0.50605373953314,-0.497358803993733,-0.490469668716376,-0.460327091817824,
-0.43729948162817,-0.425273577512184,-0.420376587364543,-0.390957251202536,
-0.362079079161669,-0.333750895422636,-0.319339724142124,-0.312267998605923,
-0.308232630749578,-0.280241862158672,-0.276106210300586,-0.247648696044962,
-0.218090837421661,-0.209492455589693,-0.204737921056362,-0.200614185310069,
-0.172780910553805,-0.145025994944757,-0.117750394973387,-0.104429823984033,
-0.100024823328952,-0.0958388020470428,-0.0691739371857627,-0.0429558817167698,
-0.017514133983365,-0.0111858270585532,0.),.UNSPECIFIED.);
#1116=B_SPLINE_CURVE_WITH_KNOTS('',3,(#60092,#60093,#60094,#60095,#60096,
#60097,#60098,#60099,#60100,#60101,#60102),.UNSPECIFIED.,.F.,.F.,(4,1,1,
1,1,1,1,1,4),(15.7079632679489,15.8048324359278,16.7912933293328,17.7777542227378,
18.7642151161428,19.7506760095478,20.7371369029528,21.7235977963578,21.9911485751285),
 .UNSPECIFIED.);
#1117=B_SPLINE_CURVE_WITH_KNOTS('',3,(#60103,#60104,#60105,#60106,#60107,
#60108,#60109,#60110,#60111,#60112),.UNSPECIFIED.,.F.,.F.,(4,1,1,1,1,1,
1,4),(15.7079632679489,16.3713219137819,17.3577828071869,18.3442437005919,
19.3307045939969,20.3171654874019,21.3036263808069,21.9911485751285),
 .UNSPECIFIED.);
#1118=B_SPLINE_CURVE_WITH_KNOTS('',3,(#60337,#60338,#60339,#60340,#60341,
#60342,#60343,#60344,#60345,#60346,#60347,#60348,#60349,#60350,#60351,#60352,
#60353,#60354,#60355,#60356,#60357,#60358,#60359,#60360,#60361,#60362,#60363,
#60364,#60365,#60366,#60367,#60368,#60369,#60370,#60371,#60372,#60373,#60374,
#60375,#60376,#60377,#60378,#60379,#60380,#60381,#60382,#60383,#60384,#60385,
#60386,#60387,#60388,#60389,#60390,#60391,#60392,#60393,#60394,#60395,#60396,
#60397,#60398,#60399,#60400,#60401,#60402,#60403,#60404,#60405,#60406,#60407,
#60408,#60409,#60410,#60411,#60412,#60413,#60414,#60415,#60416,#60417,#60418,
#60419,#60420,#60421,#60422,#60423,#60424,#60425,#60426,#60427),
 .UNSPECIFIED.,.F.,.F.,(4,3,3,3,3,3,3,3,3,3,3,3,3,3,3,3,3,3,3,3,3,3,3,3,
3,3,3,3,3,3,4),(0.,0.0253755398454445,0.0514213153132464,0.077957584539944,
0.0899764747654525,0.096803871475702,0.102648438541228,0.129953427359202,
0.157705320199216,0.184206857431119,0.195897861719558,0.201348082731475,
0.206600886453667,0.235230947526492,0.263711469126827,0.291580359310597,
0.307939787194046,0.312151069047901,0.340175334720984,0.369258031218753,
0.398694002185391,0.41802365259294,0.423204309536776,0.428148753834381,
0.459444366737233,0.482916076414372,0.491343338637999,0.498388095452059,
0.528903290158942,0.553331205445788,0.566847306048063),.UNSPECIFIED.);
#1119=B_SPLINE_CURVE_WITH_KNOTS('',3,(#60428,#60429,#60430,#60431,#60432,
#60433,#60434,#60435,#60436,#60437,#60438,#60439,#60440,#60441,#60442,#60443,
#60444,#60445,#60446,#60447,#60448,#60449,#60450,#60451,#60452),
 .UNSPECIFIED.,.F.,.F.,(4,3,3,3,3,3,3,3,4),(-10.1321597128207,-9.86460893405002,
-8.87814804064502,-7.89168714724002,-6.90522625383502,-5.91876536043002,
-4.93230446702501,-3.94584357362001,-3.84897440564113),.UNSPECIFIED.);
#1120=B_SPLINE_CURVE_WITH_KNOTS('',3,(#60677,#60678,#60679,#60680,#60681,
#60682,#60683,#60684,#60685,#60686,#60687,#60688,#60689,#60690,#60691,#60692,
#60693,#60694,#60695,#60696,#60697,#60698,#60699,#60700,#60701),
 .UNSPECIFIED.,.F.,.F.,(4,3,3,3,3,3,3,3,4),(7.59274844815666,7.89168714724002,
8.87814804064503,9.86460893405003,10.851069827455,11.83753072086,12.823991614265,
13.81045250767,13.8759337553362),.UNSPECIFIED.);
#1121=B_SPLINE_CURVE_WITH_KNOTS('',3,(#60702,#60703,#60704,#60705,#60706,
#60707,#60708,#60709,#60710,#60711,#60712,#60713,#60714,#60715,#60716,#60717,
#60718,#60719,#60720,#60721,#60722,#60723,#60724,#60725,#60726,#60727,#60728,
#60729,#60730,#60731,#60732,#60733,#60734,#60735,#60736,#60737,#60738,#60739,
#60740,#60741,#60742,#60743,#60744,#60745,#60746,#60747,#60748,#60749,#60750,
#60751,#60752,#60753,#60754,#60755,#60756,#60757,#60758,#60759,#60760,#60761,
#60762,#60763,#60764,#60765,#60766,#60767,#60768,#60769,#60770,#60771,#60772,
#60773,#60774,#60775,#60776,#60777,#60778,#60779,#60780,#60781,#60782,#60783,
#60784,#60785,#60786,#60787,#60788,#60789),.UNSPECIFIED.,.F.,.F.,(4,3,3,
3,3,3,3,3,3,3,3,3,3,3,3,3,3,3,3,3,3,3,3,3,3,3,3,3,3,4),(0.,0.0297349244535721,
0.060121569348429,0.0891410162773849,0.114533032340221,0.120626667476319,
0.15038169425931,0.17997017941563,0.208046920756741,0.230390549968388,0.234466744960236,
0.263371944870156,0.292277144780076,0.321216417936983,0.336017031727334,
0.340284462229876,0.344592011030409,0.372696707961539,0.400818636707195,
0.428516289762568,0.439576354164994,0.44540318305,0.450327524863458,0.477288294894219,
0.497472780816313,0.505235740104314,0.511959381000542,0.537907915849272,
0.558026238582596,0.569248610399449),.UNSPECIFIED.);
#2221=SHAPE_REPRESENTATION_RELATIONSHIP('SRR','None',#97615,#2240);
#2240=ADVANCED_BREP_SHAPE_REPRESENTATION('',(#2278),#97465);
#2259=STYLED_ITEM('',(#97722),#2278);
#2278=MANIFOLD_SOLID_BREP('Body1',#21820);
#2341=FACE_BOUND('',#4284,.T.);
#2342=FACE_BOUND('',#4285,.T.);
#2343=FACE_BOUND('',#4286,.T.);
#2344=FACE_BOUND('',#4287,.T.);
#2478=PLANE('',#22768);
#2479=PLANE('',#22771);
#2480=PLANE('',#22774);
#2481=PLANE('',#22777);
#2482=PLANE('',#22778);
#2483=PLANE('',#22779);
#2484=PLANE('',#22786);
#2485=PLANE('',#22787);
#3008=FACE_OUTER_BOUND('',#4215,.T.);
#3009=FACE_OUTER_BOUND('',#4216,.T.);
#3010=FACE_OUTER_BOUND('',#4217,.T.);
#3011=FACE_OUTER_BOUND('',#4218,.T.);
#3012=FACE_OUTER_BOUND('',#4219,.T.);
#3013=FACE_OUTER_BOUND('',#4220,.T.);
#3014=FACE_OUTER_BOUND('',#4221,.T.);
#3015=FACE_OUTER_BOUND('',#4222,.T.);
#3016=FACE_OUTER_BOUND('',#4223,.T.);
#3017=FACE_OUTER_BOUND('',#4224,.T.);
#3018=FACE_OUTER_BOUND('',#4225,.T.);
#3019=FACE_OUTER_BOUND('',#4226,.T.);
#3020=FACE_OUTER_BOUND('',#4227,.T.);
#3021=FACE_OUTER_BOUND('',#4228,.T.);
#3022=FACE_OUTER_BOUND('',#4229,.T.);
#3023=FACE_OUTER_BOUND('',#4230,.T.);
#3024=FACE_OUTER_BOUND('',#4231,.T.);
#3025=FACE_OUTER_BOUND('',#4232,.T.);
#3026=FACE_OUTER_BOUND('',#4233,.T.);
#3027=FACE_OUTER_BOUND('',#4234,.T.);
#3028=FACE_OUTER_BOUND('',#4235,.T.);
#3029=FACE_OUTER_BOUND('',#4236,.T.);
#3030=FACE_OUTER_BOUND('',#4237,.T.);
#3031=FACE_OUTER_BOUND('',#4238,.T.);
#3032=FACE_OUTER_BOUND('',#4239,.T.);
#3033=FACE_OUTER_BOUND('',#4240,.T.);
#3034=FACE_OUTER_BOUND('',#4241,.T.);
#3035=FACE_OUTER_BOUND('',#4242,.T.);
#3036=FACE_OUTER_BOUND('',#4243,.T.);
#3037=FACE_OUTER_BOUND('',#4244,.T.);
#3038=FACE_OUTER_BOUND('',#4245,.T.);
#3039=FACE_OUTER_BOUND('',#4246,.T.);
#3040=FACE_OUTER_BOUND('',#4247,.T.);
#3041=FACE_OUTER_BOUND('',#4248,.T.);
#3042=FACE_OUTER_BOUND('',#4249,.T.);
#3043=FACE_OUTER_BOUND('',#4250,.T.);
#3044=FACE_OUTER_BOUND('',#4251,.T.);
#3045=FACE_OUTER_BOUND('',#4252,.T.);
#3046=FACE_OUTER_BOUND('',#4253,.T.);
#3047=FACE_OUTER_BOUND('',#4254,.T.);
#3048=FACE_OUTER_BOUND('',#4255,.T.);
#3049=FACE_OUTER_BOUND('',#4256,.T.);
#3050=FACE_OUTER_BOUND('',#4257,.T.);
#3051=FACE_OUTER_BOUND('',#4258,.T.);
#3052=FACE_OUTER_BOUND('',#4259,.T.);
#3053=FACE_OUTER_BOUND('',#4260,.T.);
#3054=FACE_OUTER_BOUND('',#4261,.T.);
#3055=FACE_OUTER_BOUND('',#4262,.T.);
#3056=FACE_OUTER_BOUND('',#4263,.T.);
#3057=FACE_OUTER_BOUND('',#4264,.T.);
#3058=FACE_OUTER_BOUND('',#4265,.T.);
#3059=FACE_OUTER_BOUND('',#4266,.T.);
#3060=FACE_OUTER_BOUND('',#4267,.T.);
#3061=FACE_OUTER_BOUND('',#4268,.T.);
#3062=FACE_OUTER_BOUND('',#4269,.T.);
#3063=FACE_OUTER_BOUND('',#4270,.T.);
#3064=FACE_OUTER_BOUND('',#4271,.T.);
#3065=FACE_OUTER_BOUND('',#4272,.T.);
#3066=FACE_OUTER_BOUND('',#4273,.T.);
#3067=FACE_OUTER_BOUND('',#4274,.T.);
#3068=FACE_OUTER_BOUND('',#4275,.T.);
#3069=FACE_OUTER_BOUND('',#4276,.T.);
#3070=FACE_OUTER_BOUND('',#4277,.T.);
#3071=FACE_OUTER_BOUND('',#4278,.T.);
#3072=FACE_OUTER_BOUND('',#4279,.T.);
#3073=FACE_OUTER_BOUND('',#4280,.T.);
#3074=FACE_OUTER_BOUND('',#4281,.T.);
#3075=FACE_OUTER_BOUND('',#4282,.T.);
#3076=FACE_OUTER_BOUND('',#4283,.T.);
#3077=FACE_OUTER_BOUND('',#4288,.T.);
#4215=EDGE_LOOP('',(#15788,#15789,#15790,#15791,#15792,#15793,#15794,#15795));
#4216=EDGE_LOOP('',(#15796,#15797,#15798,#15799));
#4217=EDGE_LOOP('',(#15800,#15801,#15802,#15803));
#4218=EDGE_LOOP('',(#15804,#15805,#15806,#15807));
#4219=EDGE_LOOP('',(#15808,#15809,#15810,#15811));
#4220=EDGE_LOOP('',(#15812,#15813,#15814,#15815));
#4221=EDGE_LOOP('',(#15816,#15817,#15818,#15819));
#4222=EDGE_LOOP('',(#15820,#15821,#15822,#15823));
#4223=EDGE_LOOP('',(#15824,#15825,#15826,#15827));
#4224=EDGE_LOOP('',(#15828,#15829,#15830,#15831));
#4225=EDGE_LOOP('',(#15832,#15833,#15834,#15835));
#4226=EDGE_LOOP('',(#15836,#15837,#15838,#15839));
#4227=EDGE_LOOP('',(#15840,#15841,#15842,#15843));
#4228=EDGE_LOOP('',(#15844,#15845,#15846,#15847));
#4229=EDGE_LOOP('',(#15848,#15849,#15850,#15851));
#4230=EDGE_LOOP('',(#15852,#15853,#15854,#15855));
#4231=EDGE_LOOP('',(#15856,#15857,#15858,#15859,#15860,#15861,#15862,#15863));
#4232=EDGE_LOOP('',(#15864,#15865,#15866,#15867));
#4233=EDGE_LOOP('',(#15868,#15869,#15870,#15871));
#4234=EDGE_LOOP('',(#15872,#15873,#15874,#15875));
#4235=EDGE_LOOP('',(#15876,#15877,#15878,#15879));
#4236=EDGE_LOOP('',(#15880,#15881,#15882,#15883));
#4237=EDGE_LOOP('',(#15884,#15885,#15886,#15887));
#4238=EDGE_LOOP('',(#15888,#15889,#15890,#15891));
#4239=EDGE_LOOP('',(#15892,#15893,#15894,#15895));
#4240=EDGE_LOOP('',(#15896,#15897,#15898,#15899));
#4241=EDGE_LOOP('',(#15900,#15901,#15902,#15903));
#4242=EDGE_LOOP('',(#15904,#15905,#15906,#15907));
#4243=EDGE_LOOP('',(#15908,#15909,#15910,#15911));
#4244=EDGE_LOOP('',(#15912,#15913,#15914,#15915));
#4245=EDGE_LOOP('',(#15916,#15917,#15918,#15919));
#4246=EDGE_LOOP('',(#15920,#15921,#15922,#15923));
#4247=EDGE_LOOP('',(#15924,#15925,#15926,#15927,#15928,#15929,#15930,#15931));
#4248=EDGE_LOOP('',(#15932,#15933,#15934,#15935));
#4249=EDGE_LOOP('',(#15936,#15937,#15938,#15939));
#4250=EDGE_LOOP('',(#15940,#15941,#15942,#15943));
#4251=EDGE_LOOP('',(#15944,#15945,#15946,#15947));
#4252=EDGE_LOOP('',(#15948,#15949,#15950,#15951));
#4253=EDGE_LOOP('',(#15952,#15953,#15954,#15955));
#4254=EDGE_LOOP('',(#15956,#15957,#15958,#15959));
#4255=EDGE_LOOP('',(#15960,#15961,#15962,#15963));
#4256=EDGE_LOOP('',(#15964,#15965,#15966,#15967));
#4257=EDGE_LOOP('',(#15968,#15969,#15970,#15971));
#4258=EDGE_LOOP('',(#15972,#15973,#15974,#15975));
#4259=EDGE_LOOP('',(#15976,#15977,#15978,#15979));
#4260=EDGE_LOOP('',(#15980,#15981,#15982,#15983));
#4261=EDGE_LOOP('',(#15984,#15985,#15986,#15987));
#4262=EDGE_LOOP('',(#15988,#15989,#15990,#15991));
#4263=EDGE_LOOP('',(#15992,#15993,#15994,#15995,#15996));
#4264=EDGE_LOOP('',(#15997,#15998,#15999,#16000));
#4265=EDGE_LOOP('',(#16001,#16002,#16003,#16004,#16005,#16006,#16007,#16008,
#16009,#16010,#16011,#16012,#16013,#16014,#16015,#16016,#16017,#16018,#16019,
#16020));
#4266=EDGE_LOOP('',(#16021,#16022,#16023,#16024,#16025,#16026,#16027,#16028,
#16029,#16030,#16031,#16032,#16033,#16034,#16035,#16036,#16037,#16038,#16039,
#16040));
#4267=EDGE_LOOP('',(#16041,#16042,#16043,#16044));
#4268=EDGE_LOOP('',(#16045,#16046,#16047,#16048,#16049));
#4269=EDGE_LOOP('',(#16050,#16051,#16052,#16053));
#4270=EDGE_LOOP('',(#16054,#16055,#16056,#16057,#16058,#16059,#16060,#16061,
#16062,#16063,#16064,#16065,#16066,#16067,#16068,#16069,#16070,#16071,#16072,
#16073));
#4271=EDGE_LOOP('',(#16074,#16075,#16076,#16077,#16078,#16079,#16080,#16081,
#16082,#16083,#16084,#16085,#16086,#16087,#16088,#16089,#16090,#16091,#16092,
#16093));
#4272=EDGE_LOOP('',(#16094,#16095,#16096,#16097));
#4273=EDGE_LOOP('',(#16098,#16099,#16100,#16101,#16102));
#4274=EDGE_LOOP('',(#16103,#16104,#16105,#16106));
#4275=EDGE_LOOP('',(#16107,#16108,#16109,#16110,#16111,#16112,#16113,#16114,
#16115,#16116,#16117,#16118,#16119,#16120,#16121,#16122,#16123,#16124,#16125,
#16126));
#4276=EDGE_LOOP('',(#16127,#16128,#16129,#16130,#16131,#16132,#16133,#16134,
#16135,#16136,#16137,#16138,#16139,#16140,#16141,#16142,#16143,#16144,#16145,
#16146));
#4277=EDGE_LOOP('',(#16147,#16148,#16149,#16150));
#4278=EDGE_LOOP('',(#16151));
#4279=EDGE_LOOP('',(#16152));
#4280=EDGE_LOOP('',(#16153));
#4281=EDGE_LOOP('',(#16154,#16155,#16156));
#4282=EDGE_LOOP('',(#16157,#16158,#16159,#16160));
#4283=EDGE_LOOP('',(#16161));
#4284=EDGE_LOOP('',(#16162,#16163,#16164,#16165));
#4285=EDGE_LOOP('',(#16166,#16167,#16168,#16169));
#4286=EDGE_LOOP('',(#16170,#16171,#16172,#16173));
#4287=EDGE_LOOP('',(#16174));
#4288=EDGE_LOOP('',(#16175));
#5494=LINE('',#56456,#6708);
#5495=LINE('',#56465,#6709);
#5496=LINE('',#56482,#6710);
#5497=LINE('',#56533,#6711);
#5498=LINE('',#56584,#6712);
#5499=LINE('',#56632,#6713);
#5500=LINE('',#56683,#6714);
#5501=LINE('',#56734,#6715);
#5502=LINE('',#56782,#6716);
#5503=LINE('',#56821,#6717);
#5504=LINE('',#56845,#6718);
#5505=LINE('',#56869,#6719);
#5506=LINE('',#56894,#6720);
#5507=LINE('',#56919,#6721);
#5508=LINE('',#56943,#6722);
#5509=LINE('',#56968,#6723);
#5510=LINE('',#56993,#6724);
#5511=LINE('',#57010,#6725);
#5512=LINE('',#57019,#6726);
#5513=LINE('',#57036,#6727);
#5514=LINE('',#57087,#6728);
#5515=LINE('',#57138,#6729);
#5516=LINE('',#57186,#6730);
#5517=LINE('',#57237,#6731);
#5518=LINE('',#57288,#6732);
#5519=LINE('',#57336,#6733);
#5520=LINE('',#57375,#6734);
#5521=LINE('',#57399,#6735);
#5522=LINE('',#57423,#6736);
#5523=LINE('',#57448,#6737);
#5524=LINE('',#57473,#6738);
#5525=LINE('',#57497,#6739);
#5526=LINE('',#57522,#6740);
#5527=LINE('',#57547,#6741);
#5528=LINE('',#57564,#6742);
#5529=LINE('',#57573,#6743);
#5530=LINE('',#57590,#6744);
#5531=LINE('',#57641,#6745);
#5532=LINE('',#57692,#6746);
#5533=LINE('',#57740,#6747);
#5534=LINE('',#57791,#6748);
#5535=LINE('',#57842,#6749);
#5536=LINE('',#57890,#6750);
#5537=LINE('',#57929,#6751);
#5538=LINE('',#57953,#6752);
#5539=LINE('',#57977,#6753);
#5540=LINE('',#58002,#6754);
#5541=LINE('',#58027,#6755);
#5542=LINE('',#58051,#6756);
#5543=LINE('',#58076,#6757);
#5544=LINE('',#58101,#6758);
#5545=LINE('',#60803,#6759);
#6708=VECTOR('',#25386,3.);
#6709=VECTOR('',#25389,3.);
#6710=VECTOR('',#25396,3.);
#6711=VECTOR('',#25399,3.);
#6712=VECTOR('',#25402,3.);
#6713=VECTOR('',#25405,3.);
#6714=VECTOR('',#25408,3.);
#6715=VECTOR('',#25411,3.);
#6716=VECTOR('',#25414,3.);
#6717=VECTOR('',#25419,3.0735);
#6718=VECTOR('',#25424,3.0735);
#6719=VECTOR('',#25427,3.0735);
#6720=VECTOR('',#25430,3.0735);
#6721=VECTOR('',#25433,3.0735);
#6722=VECTOR('',#25436,3.0735);
#6723=VECTOR('',#25439,3.0735);
#6724=VECTOR('',#25442,3.0735);
#6725=VECTOR('',#25447,3.);
#6726=VECTOR('',#25450,3.);
#6727=VECTOR('',#25457,3.);
#6728=VECTOR('',#25460,3.);
#6729=VECTOR('',#25463,3.);
#6730=VECTOR('',#25466,3.);
#6731=VECTOR('',#25469,3.);
#6732=VECTOR('',#25472,3.);
#6733=VECTOR('',#25475,3.);
#6734=VECTOR('',#25480,3.0735);
#6735=VECTOR('',#25485,3.0735);
#6736=VECTOR('',#25488,3.0735);
#6737=VECTOR('',#25491,3.0735);
#6738=VECTOR('',#25494,3.0735);
#6739=VECTOR('',#25497,3.0735);
#6740=VECTOR('',#25500,3.0735);
#6741=VECTOR('',#25503,3.0735);
#6742=VECTOR('',#25508,3.);
#6743=VECTOR('',#25511,3.);
#6744=VECTOR('',#25518,3.);
#6745=VECTOR('',#25521,3.);
#6746=VECTOR('',#25524,3.);
#6747=VECTOR('',#25527,3.);
#6748=VECTOR('',#25530,3.);
#6749=VECTOR('',#25533,3.);
#6750=VECTOR('',#25536,3.);
#6751=VECTOR('',#25541,3.0735);
#6752=VECTOR('',#25546,3.0735);
#6753=VECTOR('',#25549,3.0735);
#6754=VECTOR('',#25552,3.0735);
#6755=VECTOR('',#25555,3.0735);
#6756=VECTOR('',#25558,3.0735);
#6757=VECTOR('',#25561,3.0735);
#6758=VECTOR('',#25564,3.0735);
#6759=VECTOR('',#25601,30.);
#7518=CIRCLE('',#22703,2.5175);
#7519=CIRCLE('',#22704,2.5175);
#7520=CIRCLE('',#22705,2.5175);
#7521=CIRCLE('',#22713,2.5175);
#7522=CIRCLE('',#22715,3.0735);
#7523=CIRCLE('',#22723,3.0735);
#7524=CIRCLE('',#22725,2.5175);
#7525=CIRCLE('',#22726,2.5175);
#7526=CIRCLE('',#22727,2.5175);
#7527=CIRCLE('',#22735,2.5175);
#7528=CIRCLE('',#22737,3.0735);
#7529=CIRCLE('',#22745,3.0735);
#7530=CIRCLE('',#22747,2.5175);
#7531=CIRCLE('',#22748,2.5175);
#7532=CIRCLE('',#22749,2.5175);
#7533=CIRCLE('',#22757,2.5175);
#7534=CIRCLE('',#22759,3.0735);
#7535=CIRCLE('',#22767,3.0735);
#7536=CIRCLE('',#22781,5.65685424949238);
#7537=CIRCLE('',#22782,6.);
#7538=CIRCLE('',#22784,30.);
#7539=CIRCLE('',#22785,30.);
#8505=VERTEX_POINT('',#56454);
#8506=VERTEX_POINT('',#56455);
#8507=VERTEX_POINT('',#56457);
#8508=VERTEX_POINT('',#56462);
#8509=VERTEX_POINT('',#56464);
#8510=VERTEX_POINT('',#56467);
#8511=VERTEX_POINT('',#56480);
#8512=VERTEX_POINT('',#56481);
#8513=VERTEX_POINT('',#56531);
#8514=VERTEX_POINT('',#56532);
#8515=VERTEX_POINT('',#56582);
#8516=VERTEX_POINT('',#56583);
#8517=VERTEX_POINT('',#56630);
#8518=VERTEX_POINT('',#56631);
#8519=VERTEX_POINT('',#56681);
#8520=VERTEX_POINT('',#56682);
#8521=VERTEX_POINT('',#56732);
#8522=VERTEX_POINT('',#56733);
#8523=VERTEX_POINT('',#56780);
#8524=VERTEX_POINT('',#56781);
#8525=VERTEX_POINT('',#56783);
#8526=VERTEX_POINT('',#56797);
#8527=VERTEX_POINT('',#56819);
#8528=VERTEX_POINT('',#56820);
#8529=VERTEX_POINT('',#56822);
#8530=VERTEX_POINT('',#56831);
#8531=VERTEX_POINT('',#56843);
#8532=VERTEX_POINT('',#56844);
#8533=VERTEX_POINT('',#56867);
#8534=VERTEX_POINT('',#56868);
#8535=VERTEX_POINT('',#56892);
#8536=VERTEX_POINT('',#56893);
#8537=VERTEX_POINT('',#56917);
#8538=VERTEX_POINT('',#56918);
#8539=VERTEX_POINT('',#56941);
#8540=VERTEX_POINT('',#56942);
#8541=VERTEX_POINT('',#56966);
#8542=VERTEX_POINT('',#56967);
#8543=VERTEX_POINT('',#56991);
#8544=VERTEX_POINT('',#56992);
#8545=VERTEX_POINT('',#56994);
#8546=VERTEX_POINT('',#57000);
#8547=VERTEX_POINT('',#57008);
#8548=VERTEX_POINT('',#57009);
#8549=VERTEX_POINT('',#57011);
#8550=VERTEX_POINT('',#57016);
#8551=VERTEX_POINT('',#57018);
#8552=VERTEX_POINT('',#57021);
#8553=VERTEX_POINT('',#57034);
#8554=VERTEX_POINT('',#57035);
#8555=VERTEX_POINT('',#57085);
#8556=VERTEX_POINT('',#57086);
#8557=VERTEX_POINT('',#57136);
#8558=VERTEX_POINT('',#57137);
#8559=VERTEX_POINT('',#57184);
#8560=VERTEX_POINT('',#57185);
#8561=VERTEX_POINT('',#57235);
#8562=VERTEX_POINT('',#57236);
#8563=VERTEX_POINT('',#57286);
#8564=VERTEX_POINT('',#57287);
#8565=VERTEX_POINT('',#57334);
#8566=VERTEX_POINT('',#57335);
#8567=VERTEX_POINT('',#57337);
#8568=VERTEX_POINT('',#57351);
#8569=VERTEX_POINT('',#57373);
#8570=VERTEX_POINT('',#57374);
#8571=VERTEX_POINT('',#57376);
#8572=VERTEX_POINT('',#57385);
#8573=VERTEX_POINT('',#57397);
#8574=VERTEX_POINT('',#57398);
#8575=VERTEX_POINT('',#57421);
#8576=VERTEX_POINT('',#57422);
#8577=VERTEX_POINT('',#57446);
#8578=VERTEX_POINT('',#57447);
#8579=VERTEX_POINT('',#57471);
#8580=VERTEX_POINT('',#57472);
#8581=VERTEX_POINT('',#57495);
#8582=VERTEX_POINT('',#57496);
#8583=VERTEX_POINT('',#57520);
#8584=VERTEX_POINT('',#57521);
#8585=VERTEX_POINT('',#57545);
#8586=VERTEX_POINT('',#57546);
#8587=VERTEX_POINT('',#57548);
#8588=VERTEX_POINT('',#57554);
#8589=VERTEX_POINT('',#57562);
#8590=VERTEX_POINT('',#57563);
#8591=VERTEX_POINT('',#57565);
#8592=VERTEX_POINT('',#57570);
#8593=VERTEX_POINT('',#57572);
#8594=VERTEX_POINT('',#57575);
#8595=VERTEX_POINT('',#57588);
#8596=VERTEX_POINT('',#57589);
#8597=VERTEX_POINT('',#57639);
#8598=VERTEX_POINT('',#57640);
#8599=VERTEX_POINT('',#57690);
#8600=VERTEX_POINT('',#57691);
#8601=VERTEX_POINT('',#57738);
#8602=VERTEX_POINT('',#57739);
#8603=VERTEX_POINT('',#57789);
#8604=VERTEX_POINT('',#57790);
#8605=VERTEX_POINT('',#57840);
#8606=VERTEX_POINT('',#57841);
#8607=VERTEX_POINT('',#57888);
#8608=VERTEX_POINT('',#57889);
#8609=VERTEX_POINT('',#57891);
#8610=VERTEX_POINT('',#57905);
#8611=VERTEX_POINT('',#57927);
#8612=VERTEX_POINT('',#57928);
#8613=VERTEX_POINT('',#57930);
#8614=VERTEX_POINT('',#57939);
#8615=VERTEX_POINT('',#57951);
#8616=VERTEX_POINT('',#57952);
#8617=VERTEX_POINT('',#57975);
#8618=VERTEX_POINT('',#57976);
#8619=VERTEX_POINT('',#58000);
#8620=VERTEX_POINT('',#58001);
#8621=VERTEX_POINT('',#58025);
#8622=VERTEX_POINT('',#58026);
#8623=VERTEX_POINT('',#58049);
#8624=VERTEX_POINT('',#58050);
#8625=VERTEX_POINT('',#58074);
#8626=VERTEX_POINT('',#58075);
#8627=VERTEX_POINT('',#58099);
#8628=VERTEX_POINT('',#58100);
#8629=VERTEX_POINT('',#58102);
#8630=VERTEX_POINT('',#58108);
#8631=VERTEX_POINT('',#60795);
#8632=VERTEX_POINT('',#60797);
#8633=VERTEX_POINT('',#60800);
#8634=VERTEX_POINT('',#60802);
#11151=EDGE_CURVE('',#8505,#8506,#5494,.T.);
#11152=EDGE_CURVE('',#8506,#8507,#1002,.T.);
#11153=EDGE_CURVE('',#8507,#8508,#7518,.T.);
#11154=EDGE_CURVE('',#8508,#8509,#5495,.T.);
#11155=EDGE_CURVE('',#8509,#8509,#7519,.F.);
#11156=EDGE_CURVE('',#8508,#8510,#7520,.T.);
#11157=EDGE_CURVE('',#8510,#8505,#1003,.T.);
#11158=EDGE_CURVE('',#8511,#8512,#5496,.T.);
#11159=EDGE_CURVE('',#8512,#8506,#1004,.T.);
#11160=EDGE_CURVE('',#8505,#8511,#1005,.T.);
#11161=EDGE_CURVE('',#8513,#8514,#5497,.T.);
#11162=EDGE_CURVE('',#8514,#8512,#1006,.T.);
#11163=EDGE_CURVE('',#8511,#8513,#1007,.T.);
#11164=EDGE_CURVE('',#8515,#8516,#5498,.T.);
#11165=EDGE_CURVE('',#8516,#8514,#1008,.T.);
#11166=EDGE_CURVE('',#8513,#8515,#1009,.T.);
#11167=EDGE_CURVE('',#8517,#8518,#5499,.T.);
#11168=EDGE_CURVE('',#8518,#8516,#1010,.T.);
#11169=EDGE_CURVE('',#8515,#8517,#1011,.T.);
#11170=EDGE_CURVE('',#8519,#8520,#5500,.T.);
#11171=EDGE_CURVE('',#8520,#8518,#1012,.T.);
#11172=EDGE_CURVE('',#8517,#8519,#1013,.T.);
#11173=EDGE_CURVE('',#8521,#8522,#5501,.T.);
#11174=EDGE_CURVE('',#8522,#8520,#1014,.T.);
#11175=EDGE_CURVE('',#8519,#8521,#1015,.T.);
#11176=EDGE_CURVE('',#8523,#8524,#5502,.T.);
#11177=EDGE_CURVE('',#8523,#8525,#1016,.T.);
#11178=EDGE_CURVE('',#8526,#8525,#7521,.T.);
#11179=EDGE_CURVE('',#8526,#8524,#1017,.T.);
#11180=EDGE_CURVE('',#8527,#8528,#5503,.T.);
#11181=EDGE_CURVE('',#8528,#8529,#1018,.T.);
#11182=EDGE_CURVE('',#8530,#8529,#7522,.T.);
#11183=EDGE_CURVE('',#8527,#8530,#1019,.T.);
#11184=EDGE_CURVE('',#8531,#8532,#5504,.T.);
#11185=EDGE_CURVE('',#8532,#8528,#1020,.T.);
#11186=EDGE_CURVE('',#8531,#8527,#1021,.T.);
#11187=EDGE_CURVE('',#8533,#8534,#5505,.T.);
#11188=EDGE_CURVE('',#8534,#8532,#1022,.T.);
#11189=EDGE_CURVE('',#8533,#8531,#1023,.T.);
#11190=EDGE_CURVE('',#8535,#8536,#5506,.T.);
#11191=EDGE_CURVE('',#8536,#8534,#1024,.T.);
#11192=EDGE_CURVE('',#8535,#8533,#1025,.T.);
#11193=EDGE_CURVE('',#8537,#8538,#5507,.T.);
#11194=EDGE_CURVE('',#8538,#8536,#1026,.T.);
#11195=EDGE_CURVE('',#8537,#8535,#1027,.T.);
#11196=EDGE_CURVE('',#8539,#8540,#5508,.T.);
#11197=EDGE_CURVE('',#8540,#8538,#1028,.T.);
#11198=EDGE_CURVE('',#8539,#8537,#1029,.T.);
#11199=EDGE_CURVE('',#8541,#8542,#5509,.T.);
#11200=EDGE_CURVE('',#8542,#8540,#1030,.T.);
#11201=EDGE_CURVE('',#8541,#8539,#1031,.T.);
#11202=EDGE_CURVE('',#8543,#8544,#5510,.T.);
#11203=EDGE_CURVE('',#8545,#8543,#1032,.T.);
#11204=EDGE_CURVE('',#8546,#8545,#7523,.T.);
#11205=EDGE_CURVE('',#8546,#8544,#1033,.T.);
#11206=EDGE_CURVE('',#8547,#8548,#5511,.T.);
#11207=EDGE_CURVE('',#8548,#8549,#1034,.T.);
#11208=EDGE_CURVE('',#8549,#8550,#7524,.T.);
#11209=EDGE_CURVE('',#8550,#8551,#5512,.T.);
#11210=EDGE_CURVE('',#8551,#8551,#7525,.F.);
#11211=EDGE_CURVE('',#8550,#8552,#7526,.T.);
#11212=EDGE_CURVE('',#8552,#8547,#1035,.T.);
#11213=EDGE_CURVE('',#8553,#8554,#5513,.T.);
#11214=EDGE_CURVE('',#8554,#8548,#1036,.T.);
#11215=EDGE_CURVE('',#8547,#8553,#1037,.T.);
#11216=EDGE_CURVE('',#8555,#8556,#5514,.T.);
#11217=EDGE_CURVE('',#8556,#8554,#1038,.T.);
#11218=EDGE_CURVE('',#8553,#8555,#1039,.T.);
#11219=EDGE_CURVE('',#8557,#8558,#5515,.T.);
#11220=EDGE_CURVE('',#8558,#8556,#1040,.T.);
#11221=EDGE_CURVE('',#8555,#8557,#1041,.T.);
#11222=EDGE_CURVE('',#8559,#8560,#5516,.T.);
#11223=EDGE_CURVE('',#8560,#8558,#1042,.T.);
#11224=EDGE_CURVE('',#8557,#8559,#1043,.T.);
#11225=EDGE_CURVE('',#8561,#8562,#5517,.T.);
#11226=EDGE_CURVE('',#8562,#8560,#1044,.T.);
#11227=EDGE_CURVE('',#8559,#8561,#1045,.T.);
#11228=EDGE_CURVE('',#8563,#8564,#5518,.T.);
#11229=EDGE_CURVE('',#8564,#8562,#1046,.T.);
#11230=EDGE_CURVE('',#8561,#8563,#1047,.T.);
#11231=EDGE_CURVE('',#8565,#8566,#5519,.T.);
#11232=EDGE_CURVE('',#8565,#8567,#1048,.T.);
#11233=EDGE_CURVE('',#8568,#8567,#7527,.T.);
#11234=EDGE_CURVE('',#8568,#8566,#1049,.T.);
#11235=EDGE_CURVE('',#8569,#8570,#5520,.T.);
#11236=EDGE_CURVE('',#8570,#8571,#1050,.T.);
#11237=EDGE_CURVE('',#8572,#8571,#7528,.T.);
#11238=EDGE_CURVE('',#8569,#8572,#1051,.T.);
#11239=EDGE_CURVE('',#8573,#8574,#5521,.T.);
#11240=EDGE_CURVE('',#8574,#8570,#1052,.T.);
#11241=EDGE_CURVE('',#8573,#8569,#1053,.T.);
#11242=EDGE_CURVE('',#8575,#8576,#5522,.T.);
#11243=EDGE_CURVE('',#8576,#8574,#1054,.T.);
#11244=EDGE_CURVE('',#8575,#8573,#1055,.T.);
#11245=EDGE_CURVE('',#8577,#8578,#5523,.T.);
#11246=EDGE_CURVE('',#8578,#8576,#1056,.T.);
#11247=EDGE_CURVE('',#8577,#8575,#1057,.T.);
#11248=EDGE_CURVE('',#8579,#8580,#5524,.T.);
#11249=EDGE_CURVE('',#8580,#8578,#1058,.T.);
#11250=EDGE_CURVE('',#8579,#8577,#1059,.T.);
#11251=EDGE_CURVE('',#8581,#8582,#5525,.T.);
#11252=EDGE_CURVE('',#8582,#8580,#1060,.T.);
#11253=EDGE_CURVE('',#8581,#8579,#1061,.T.);
#11254=EDGE_CURVE('',#8583,#8584,#5526,.T.);
#11255=EDGE_CURVE('',#8584,#8582,#1062,.T.);
#11256=EDGE_CURVE('',#8583,#8581,#1063,.T.);
#11257=EDGE_CURVE('',#8585,#8586,#5527,.T.);
#11258=EDGE_CURVE('',#8587,#8585,#1064,.T.);
#11259=EDGE_CURVE('',#8588,#8587,#7529,.T.);
#11260=EDGE_CURVE('',#8588,#8586,#1065,.T.);
#11261=EDGE_CURVE('',#8589,#8590,#5528,.T.);
#11262=EDGE_CURVE('',#8590,#8591,#1066,.T.);
#11263=EDGE_CURVE('',#8591,#8592,#7530,.T.);
#11264=EDGE_CURVE('',#8592,#8593,#5529,.T.);
#11265=EDGE_CURVE('',#8593,#8593,#7531,.F.);
#11266=EDGE_CURVE('',#8592,#8594,#7532,.T.);
#11267=EDGE_CURVE('',#8594,#8589,#1067,.T.);
#11268=EDGE_CURVE('',#8595,#8596,#5530,.T.);
#11269=EDGE_CURVE('',#8596,#8590,#1068,.T.);
#11270=EDGE_CURVE('',#8589,#8595,#1069,.T.);
#11271=EDGE_CURVE('',#8597,#8598,#5531,.T.);
#11272=EDGE_CURVE('',#8598,#8596,#1070,.T.);
#11273=EDGE_CURVE('',#8595,#8597,#1071,.T.);
#11274=EDGE_CURVE('',#8599,#8600,#5532,.T.);
#11275=EDGE_CURVE('',#8600,#8598,#1072,.T.);
#11276=EDGE_CURVE('',#8597,#8599,#1073,.T.);
#11277=EDGE_CURVE('',#8601,#8602,#5533,.T.);
#11278=EDGE_CURVE('',#8602,#8600,#1074,.T.);
#11279=EDGE_CURVE('',#8599,#8601,#1075,.T.);
#11280=EDGE_CURVE('',#8603,#8604,#5534,.T.);
#11281=EDGE_CURVE('',#8604,#8602,#1076,.T.);
#11282=EDGE_CURVE('',#8601,#8603,#1077,.T.);
#11283=EDGE_CURVE('',#8605,#8606,#5535,.T.);
#11284=EDGE_CURVE('',#8606,#8604,#1078,.T.);
#11285=EDGE_CURVE('',#8603,#8605,#1079,.T.);
#11286=EDGE_CURVE('',#8607,#8608,#5536,.T.);
#11287=EDGE_CURVE('',#8607,#8609,#1080,.T.);
#11288=EDGE_CURVE('',#8610,#8609,#7533,.T.);
#11289=EDGE_CURVE('',#8610,#8608,#1081,.T.);
#11290=EDGE_CURVE('',#8611,#8612,#5537,.T.);
#11291=EDGE_CURVE('',#8612,#8613,#1082,.T.);
#11292=EDGE_CURVE('',#8614,#8613,#7534,.T.);
#11293=EDGE_CURVE('',#8611,#8614,#1083,.T.);
#11294=EDGE_CURVE('',#8615,#8616,#5538,.T.);
#11295=EDGE_CURVE('',#8616,#8612,#1084,.T.);
#11296=EDGE_CURVE('',#8615,#8611,#1085,.T.);
#11297=EDGE_CURVE('',#8617,#8618,#5539,.T.);
#11298=EDGE_CURVE('',#8618,#8616,#1086,.T.);
#11299=EDGE_CURVE('',#8617,#8615,#1087,.T.);
#11300=EDGE_CURVE('',#8619,#8620,#5540,.T.);
#11301=EDGE_CURVE('',#8620,#8618,#1088,.T.);
#11302=EDGE_CURVE('',#8619,#8617,#1089,.T.);
#11303=EDGE_CURVE('',#8621,#8622,#5541,.T.);
#11304=EDGE_CURVE('',#8622,#8620,#1090,.T.);
#11305=EDGE_CURVE('',#8621,#8619,#1091,.T.);
#11306=EDGE_CURVE('',#8623,#8624,#5542,.T.);
#11307=EDGE_CURVE('',#8624,#8622,#1092,.T.);
#11308=EDGE_CURVE('',#8623,#8621,#1093,.T.);
#11309=EDGE_CURVE('',#8625,#8626,#5543,.T.);
#11310=EDGE_CURVE('',#8626,#8624,#1094,.T.);
#11311=EDGE_CURVE('',#8625,#8623,#1095,.T.);
#11312=EDGE_CURVE('',#8627,#8628,#5544,.T.);
#11313=EDGE_CURVE('',#8629,#8627,#1096,.T.);
#11314=EDGE_CURVE('',#8630,#8629,#7535,.T.);
#11315=EDGE_CURVE('',#8630,#8628,#1097,.T.);
#11316=EDGE_CURVE('',#8591,#8614,#1098,.T.);
#11317=EDGE_CURVE('',#8613,#8594,#1099,.T.);
#11318=EDGE_CURVE('',#8628,#8626,#1100,.T.);
#11319=EDGE_CURVE('',#8627,#8625,#1101,.T.);
#11320=EDGE_CURVE('',#8609,#8630,#1102,.T.);
#11321=EDGE_CURVE('',#8605,#8607,#1103,.T.);
#11322=EDGE_CURVE('',#8608,#8606,#1104,.T.);
#11323=EDGE_CURVE('',#8629,#8610,#1105,.T.);
#11324=EDGE_CURVE('',#8549,#8572,#1106,.T.);
#11325=EDGE_CURVE('',#8571,#8552,#1107,.T.);
#11326=EDGE_CURVE('',#8586,#8584,#1108,.T.);
#11327=EDGE_CURVE('',#8585,#8583,#1109,.T.);
#11328=EDGE_CURVE('',#8567,#8588,#1110,.T.);
#11329=EDGE_CURVE('',#8563,#8565,#1111,.T.);
#11330=EDGE_CURVE('',#8566,#8564,#1112,.T.);
#11331=EDGE_CURVE('',#8587,#8568,#1113,.T.);
#11332=EDGE_CURVE('',#8507,#8530,#1114,.T.);
#11333=EDGE_CURVE('',#8529,#8510,#1115,.T.);
#11334=EDGE_CURVE('',#8544,#8542,#1116,.T.);
#11335=EDGE_CURVE('',#8543,#8541,#1117,.T.);
#11336=EDGE_CURVE('',#8525,#8546,#1118,.T.);
#11337=EDGE_CURVE('',#8521,#8523,#1119,.T.);
#11338=EDGE_CURVE('',#8524,#8522,#1120,.T.);
#11339=EDGE_CURVE('',#8545,#8526,#1121,.T.);
#11340=EDGE_CURVE('',#8631,#8631,#7536,.T.);
#11341=EDGE_CURVE('',#8632,#8631,#7537,.T.);
#11342=EDGE_CURVE('',#8633,#8633,#7538,.T.);
#11343=EDGE_CURVE('',#8633,#8634,#5545,.T.);
#11344=EDGE_CURVE('',#8634,#8634,#7539,.T.);
#15788=ORIENTED_EDGE('',*,*,#11151,.T.);
#15789=ORIENTED_EDGE('',*,*,#11152,.T.);
#15790=ORIENTED_EDGE('',*,*,#11153,.T.);
#15791=ORIENTED_EDGE('',*,*,#11154,.T.);
#15792=ORIENTED_EDGE('',*,*,#11155,.T.);
#15793=ORIENTED_EDGE('',*,*,#11154,.F.);
#15794=ORIENTED_EDGE('',*,*,#11156,.T.);
#15795=ORIENTED_EDGE('',*,*,#11157,.T.);
#15796=ORIENTED_EDGE('',*,*,#11158,.T.);
#15797=ORIENTED_EDGE('',*,*,#11159,.T.);
#15798=ORIENTED_EDGE('',*,*,#11151,.F.);
#15799=ORIENTED_EDGE('',*,*,#11160,.T.);
#15800=ORIENTED_EDGE('',*,*,#11161,.T.);
#15801=ORIENTED_EDGE('',*,*,#11162,.T.);
#15802=ORIENTED_EDGE('',*,*,#11158,.F.);
#15803=ORIENTED_EDGE('',*,*,#11163,.T.);
#15804=ORIENTED_EDGE('',*,*,#11164,.T.);
#15805=ORIENTED_EDGE('',*,*,#11165,.T.);
#15806=ORIENTED_EDGE('',*,*,#11161,.F.);
#15807=ORIENTED_EDGE('',*,*,#11166,.T.);
#15808=ORIENTED_EDGE('',*,*,#11167,.T.);
#15809=ORIENTED_EDGE('',*,*,#11168,.T.);
#15810=ORIENTED_EDGE('',*,*,#11164,.F.);
#15811=ORIENTED_EDGE('',*,*,#11169,.T.);
#15812=ORIENTED_EDGE('',*,*,#11170,.T.);
#15813=ORIENTED_EDGE('',*,*,#11171,.T.);
#15814=ORIENTED_EDGE('',*,*,#11167,.F.);
#15815=ORIENTED_EDGE('',*,*,#11172,.T.);
#15816=ORIENTED_EDGE('',*,*,#11173,.T.);
#15817=ORIENTED_EDGE('',*,*,#11174,.T.);
#15818=ORIENTED_EDGE('',*,*,#11170,.F.);
#15819=ORIENTED_EDGE('',*,*,#11175,.T.);
#15820=ORIENTED_EDGE('',*,*,#11176,.F.);
#15821=ORIENTED_EDGE('',*,*,#11177,.T.);
#15822=ORIENTED_EDGE('',*,*,#11178,.F.);
#15823=ORIENTED_EDGE('',*,*,#11179,.T.);
#15824=ORIENTED_EDGE('',*,*,#11180,.T.);
#15825=ORIENTED_EDGE('',*,*,#11181,.T.);
#15826=ORIENTED_EDGE('',*,*,#11182,.F.);
#15827=ORIENTED_EDGE('',*,*,#11183,.F.);
#15828=ORIENTED_EDGE('',*,*,#11184,.T.);
#15829=ORIENTED_EDGE('',*,*,#11185,.T.);
#15830=ORIENTED_EDGE('',*,*,#11180,.F.);
#15831=ORIENTED_EDGE('',*,*,#11186,.F.);
#15832=ORIENTED_EDGE('',*,*,#11187,.T.);
#15833=ORIENTED_EDGE('',*,*,#11188,.T.);
#15834=ORIENTED_EDGE('',*,*,#11184,.F.);
#15835=ORIENTED_EDGE('',*,*,#11189,.F.);
#15836=ORIENTED_EDGE('',*,*,#11190,.T.);
#15837=ORIENTED_EDGE('',*,*,#11191,.T.);
#15838=ORIENTED_EDGE('',*,*,#11187,.F.);
#15839=ORIENTED_EDGE('',*,*,#11192,.F.);
#15840=ORIENTED_EDGE('',*,*,#11193,.T.);
#15841=ORIENTED_EDGE('',*,*,#11194,.T.);
#15842=ORIENTED_EDGE('',*,*,#11190,.F.);
#15843=ORIENTED_EDGE('',*,*,#11195,.F.);
#15844=ORIENTED_EDGE('',*,*,#11196,.T.);
#15845=ORIENTED_EDGE('',*,*,#11197,.T.);
#15846=ORIENTED_EDGE('',*,*,#11193,.F.);
#15847=ORIENTED_EDGE('',*,*,#11198,.F.);
#15848=ORIENTED_EDGE('',*,*,#11199,.T.);
#15849=ORIENTED_EDGE('',*,*,#11200,.T.);
#15850=ORIENTED_EDGE('',*,*,#11196,.F.);
#15851=ORIENTED_EDGE('',*,*,#11201,.F.);
#15852=ORIENTED_EDGE('',*,*,#11202,.F.);
#15853=ORIENTED_EDGE('',*,*,#11203,.F.);
#15854=ORIENTED_EDGE('',*,*,#11204,.F.);
#15855=ORIENTED_EDGE('',*,*,#11205,.T.);
#15856=ORIENTED_EDGE('',*,*,#11206,.T.);
#15857=ORIENTED_EDGE('',*,*,#11207,.T.);
#15858=ORIENTED_EDGE('',*,*,#11208,.T.);
#15859=ORIENTED_EDGE('',*,*,#11209,.T.);
#15860=ORIENTED_EDGE('',*,*,#11210,.T.);
#15861=ORIENTED_EDGE('',*,*,#11209,.F.);
#15862=ORIENTED_EDGE('',*,*,#11211,.T.);
#15863=ORIENTED_EDGE('',*,*,#11212,.T.);
#15864=ORIENTED_EDGE('',*,*,#11213,.T.);
#15865=ORIENTED_EDGE('',*,*,#11214,.T.);
#15866=ORIENTED_EDGE('',*,*,#11206,.F.);
#15867=ORIENTED_EDGE('',*,*,#11215,.T.);
#15868=ORIENTED_EDGE('',*,*,#11216,.T.);
#15869=ORIENTED_EDGE('',*,*,#11217,.T.);
#15870=ORIENTED_EDGE('',*,*,#11213,.F.);
#15871=ORIENTED_EDGE('',*,*,#11218,.T.);
#15872=ORIENTED_EDGE('',*,*,#11219,.T.);
#15873=ORIENTED_EDGE('',*,*,#11220,.T.);
#15874=ORIENTED_EDGE('',*,*,#11216,.F.);
#15875=ORIENTED_EDGE('',*,*,#11221,.T.);
#15876=ORIENTED_EDGE('',*,*,#11222,.T.);
#15877=ORIENTED_EDGE('',*,*,#11223,.T.);
#15878=ORIENTED_EDGE('',*,*,#11219,.F.);
#15879=ORIENTED_EDGE('',*,*,#11224,.T.);
#15880=ORIENTED_EDGE('',*,*,#11225,.T.);
#15881=ORIENTED_EDGE('',*,*,#11226,.T.);
#15882=ORIENTED_EDGE('',*,*,#11222,.F.);
#15883=ORIENTED_EDGE('',*,*,#11227,.T.);
#15884=ORIENTED_EDGE('',*,*,#11228,.T.);
#15885=ORIENTED_EDGE('',*,*,#11229,.T.);
#15886=ORIENTED_EDGE('',*,*,#11225,.F.);
#15887=ORIENTED_EDGE('',*,*,#11230,.T.);
#15888=ORIENTED_EDGE('',*,*,#11231,.F.);
#15889=ORIENTED_EDGE('',*,*,#11232,.T.);
#15890=ORIENTED_EDGE('',*,*,#11233,.F.);
#15891=ORIENTED_EDGE('',*,*,#11234,.T.);
#15892=ORIENTED_EDGE('',*,*,#11235,.T.);
#15893=ORIENTED_EDGE('',*,*,#11236,.T.);
#15894=ORIENTED_EDGE('',*,*,#11237,.F.);
#15895=ORIENTED_EDGE('',*,*,#11238,.F.);
#15896=ORIENTED_EDGE('',*,*,#11239,.T.);
#15897=ORIENTED_EDGE('',*,*,#11240,.T.);
#15898=ORIENTED_EDGE('',*,*,#11235,.F.);
#15899=ORIENTED_EDGE('',*,*,#11241,.F.);
#15900=ORIENTED_EDGE('',*,*,#11242,.T.);
#15901=ORIENTED_EDGE('',*,*,#11243,.T.);
#15902=ORIENTED_EDGE('',*,*,#11239,.F.);
#15903=ORIENTED_EDGE('',*,*,#11244,.F.);
#15904=ORIENTED_EDGE('',*,*,#11245,.T.);
#15905=ORIENTED_EDGE('',*,*,#11246,.T.);
#15906=ORIENTED_EDGE('',*,*,#11242,.F.);
#15907=ORIENTED_EDGE('',*,*,#11247,.F.);
#15908=ORIENTED_EDGE('',*,*,#11248,.T.);
#15909=ORIENTED_EDGE('',*,*,#11249,.T.);
#15910=ORIENTED_EDGE('',*,*,#11245,.F.);
#15911=ORIENTED_EDGE('',*,*,#11250,.F.);
#15912=ORIENTED_EDGE('',*,*,#11251,.T.);
#15913=ORIENTED_EDGE('',*,*,#11252,.T.);
#15914=ORIENTED_EDGE('',*,*,#11248,.F.);
#15915=ORIENTED_EDGE('',*,*,#11253,.F.);
#15916=ORIENTED_EDGE('',*,*,#11254,.T.);
#15917=ORIENTED_EDGE('',*,*,#11255,.T.);
#15918=ORIENTED_EDGE('',*,*,#11251,.F.);
#15919=ORIENTED_EDGE('',*,*,#11256,.F.);
#15920=ORIENTED_EDGE('',*,*,#11257,.F.);
#15921=ORIENTED_EDGE('',*,*,#11258,.F.);
#15922=ORIENTED_EDGE('',*,*,#11259,.F.);
#15923=ORIENTED_EDGE('',*,*,#11260,.T.);
#15924=ORIENTED_EDGE('',*,*,#11261,.T.);
#15925=ORIENTED_EDGE('',*,*,#11262,.T.);
#15926=ORIENTED_EDGE('',*,*,#11263,.T.);
#15927=ORIENTED_EDGE('',*,*,#11264,.T.);
#15928=ORIENTED_EDGE('',*,*,#11265,.T.);
#15929=ORIENTED_EDGE('',*,*,#11264,.F.);
#15930=ORIENTED_EDGE('',*,*,#11266,.T.);
#15931=ORIENTED_EDGE('',*,*,#11267,.T.);
#15932=ORIENTED_EDGE('',*,*,#11268,.T.);
#15933=ORIENTED_EDGE('',*,*,#11269,.T.);
#15934=ORIENTED_EDGE('',*,*,#11261,.F.);
#15935=ORIENTED_EDGE('',*,*,#11270,.T.);
#15936=ORIENTED_EDGE('',*,*,#11271,.T.);
#15937=ORIENTED_EDGE('',*,*,#11272,.T.);
#15938=ORIENTED_EDGE('',*,*,#11268,.F.);
#15939=ORIENTED_EDGE('',*,*,#11273,.T.);
#15940=ORIENTED_EDGE('',*,*,#11274,.T.);
#15941=ORIENTED_EDGE('',*,*,#11275,.T.);
#15942=ORIENTED_EDGE('',*,*,#11271,.F.);
#15943=ORIENTED_EDGE('',*,*,#11276,.T.);
#15944=ORIENTED_EDGE('',*,*,#11277,.T.);
#15945=ORIENTED_EDGE('',*,*,#11278,.T.);
#15946=ORIENTED_EDGE('',*,*,#11274,.F.);
#15947=ORIENTED_EDGE('',*,*,#11279,.T.);
#15948=ORIENTED_EDGE('',*,*,#11280,.T.);
#15949=ORIENTED_EDGE('',*,*,#11281,.T.);
#15950=ORIENTED_EDGE('',*,*,#11277,.F.);
#15951=ORIENTED_EDGE('',*,*,#11282,.T.);
#15952=ORIENTED_EDGE('',*,*,#11283,.T.);
#15953=ORIENTED_EDGE('',*,*,#11284,.T.);
#15954=ORIENTED_EDGE('',*,*,#11280,.F.);
#15955=ORIENTED_EDGE('',*,*,#11285,.T.);
#15956=ORIENTED_EDGE('',*,*,#11286,.F.);
#15957=ORIENTED_EDGE('',*,*,#11287,.T.);
#15958=ORIENTED_EDGE('',*,*,#11288,.F.);
#15959=ORIENTED_EDGE('',*,*,#11289,.T.);
#15960=ORIENTED_EDGE('',*,*,#11290,.T.);
#15961=ORIENTED_EDGE('',*,*,#11291,.T.);
#15962=ORIENTED_EDGE('',*,*,#11292,.F.);
#15963=ORIENTED_EDGE('',*,*,#11293,.F.);
#15964=ORIENTED_EDGE('',*,*,#11294,.T.);
#15965=ORIENTED_EDGE('',*,*,#11295,.T.);
#15966=ORIENTED_EDGE('',*,*,#11290,.F.);
#15967=ORIENTED_EDGE('',*,*,#11296,.F.);
#15968=ORIENTED_EDGE('',*,*,#11297,.T.);
#15969=ORIENTED_EDGE('',*,*,#11298,.T.);
#15970=ORIENTED_EDGE('',*,*,#11294,.F.);
#15971=ORIENTED_EDGE('',*,*,#11299,.F.);
#15972=ORIENTED_EDGE('',*,*,#11300,.T.);
#15973=ORIENTED_EDGE('',*,*,#11301,.T.);
#15974=ORIENTED_EDGE('',*,*,#11297,.F.);
#15975=ORIENTED_EDGE('',*,*,#11302,.F.);
#15976=ORIENTED_EDGE('',*,*,#11303,.T.);
#15977=ORIENTED_EDGE('',*,*,#11304,.T.);
#15978=ORIENTED_EDGE('',*,*,#11300,.F.);
#15979=ORIENTED_EDGE('',*,*,#11305,.F.);
#15980=ORIENTED_EDGE('',*,*,#11306,.T.);
#15981=ORIENTED_EDGE('',*,*,#11307,.T.);
#15982=ORIENTED_EDGE('',*,*,#11303,.F.);
#15983=ORIENTED_EDGE('',*,*,#11308,.F.);
#15984=ORIENTED_EDGE('',*,*,#11309,.T.);
#15985=ORIENTED_EDGE('',*,*,#11310,.T.);
#15986=ORIENTED_EDGE('',*,*,#11306,.F.);
#15987=ORIENTED_EDGE('',*,*,#11311,.F.);
#15988=ORIENTED_EDGE('',*,*,#11312,.F.);
#15989=ORIENTED_EDGE('',*,*,#11313,.F.);
#15990=ORIENTED_EDGE('',*,*,#11314,.F.);
#15991=ORIENTED_EDGE('',*,*,#11315,.T.);
#15992=ORIENTED_EDGE('',*,*,#11263,.F.);
#15993=ORIENTED_EDGE('',*,*,#11316,.T.);
#15994=ORIENTED_EDGE('',*,*,#11292,.T.);
#15995=ORIENTED_EDGE('',*,*,#11317,.T.);
#15996=ORIENTED_EDGE('',*,*,#11266,.F.);
#15997=ORIENTED_EDGE('',*,*,#11312,.T.);
#15998=ORIENTED_EDGE('',*,*,#11318,.T.);
#15999=ORIENTED_EDGE('',*,*,#11309,.F.);
#16000=ORIENTED_EDGE('',*,*,#11319,.F.);
#16001=ORIENTED_EDGE('',*,*,#11317,.F.);
#16002=ORIENTED_EDGE('',*,*,#11291,.F.);
#16003=ORIENTED_EDGE('',*,*,#11295,.F.);
#16004=ORIENTED_EDGE('',*,*,#11298,.F.);
#16005=ORIENTED_EDGE('',*,*,#11301,.F.);
#16006=ORIENTED_EDGE('',*,*,#11304,.F.);
#16007=ORIENTED_EDGE('',*,*,#11307,.F.);
#16008=ORIENTED_EDGE('',*,*,#11310,.F.);
#16009=ORIENTED_EDGE('',*,*,#11318,.F.);
#16010=ORIENTED_EDGE('',*,*,#11315,.F.);
#16011=ORIENTED_EDGE('',*,*,#11320,.F.);
#16012=ORIENTED_EDGE('',*,*,#11287,.F.);
#16013=ORIENTED_EDGE('',*,*,#11321,.F.);
#16014=ORIENTED_EDGE('',*,*,#11285,.F.);
#16015=ORIENTED_EDGE('',*,*,#11282,.F.);
#16016=ORIENTED_EDGE('',*,*,#11279,.F.);
#16017=ORIENTED_EDGE('',*,*,#11276,.F.);
#16018=ORIENTED_EDGE('',*,*,#11273,.F.);
#16019=ORIENTED_EDGE('',*,*,#11270,.F.);
#16020=ORIENTED_EDGE('',*,*,#11267,.F.);
#16021=ORIENTED_EDGE('',*,*,#11316,.F.);
#16022=ORIENTED_EDGE('',*,*,#11262,.F.);
#16023=ORIENTED_EDGE('',*,*,#11269,.F.);
#16024=ORIENTED_EDGE('',*,*,#11272,.F.);
#16025=ORIENTED_EDGE('',*,*,#11275,.F.);
#16026=ORIENTED_EDGE('',*,*,#11278,.F.);
#16027=ORIENTED_EDGE('',*,*,#11281,.F.);
#16028=ORIENTED_EDGE('',*,*,#11284,.F.);
#16029=ORIENTED_EDGE('',*,*,#11322,.F.);
#16030=ORIENTED_EDGE('',*,*,#11289,.F.);
#16031=ORIENTED_EDGE('',*,*,#11323,.F.);
#16032=ORIENTED_EDGE('',*,*,#11313,.T.);
#16033=ORIENTED_EDGE('',*,*,#11319,.T.);
#16034=ORIENTED_EDGE('',*,*,#11311,.T.);
#16035=ORIENTED_EDGE('',*,*,#11308,.T.);
#16036=ORIENTED_EDGE('',*,*,#11305,.T.);
#16037=ORIENTED_EDGE('',*,*,#11302,.T.);
#16038=ORIENTED_EDGE('',*,*,#11299,.T.);
#16039=ORIENTED_EDGE('',*,*,#11296,.T.);
#16040=ORIENTED_EDGE('',*,*,#11293,.T.);
#16041=ORIENTED_EDGE('',*,*,#11286,.T.);
#16042=ORIENTED_EDGE('',*,*,#11322,.T.);
#16043=ORIENTED_EDGE('',*,*,#11283,.F.);
#16044=ORIENTED_EDGE('',*,*,#11321,.T.);
#16045=ORIENTED_EDGE('',*,*,#11208,.F.);
#16046=ORIENTED_EDGE('',*,*,#11324,.T.);
#16047=ORIENTED_EDGE('',*,*,#11237,.T.);
#16048=ORIENTED_EDGE('',*,*,#11325,.T.);
#16049=ORIENTED_EDGE('',*,*,#11211,.F.);
#16050=ORIENTED_EDGE('',*,*,#11257,.T.);
#16051=ORIENTED_EDGE('',*,*,#11326,.T.);
#16052=ORIENTED_EDGE('',*,*,#11254,.F.);
#16053=ORIENTED_EDGE('',*,*,#11327,.F.);
#16054=ORIENTED_EDGE('',*,*,#11325,.F.);
#16055=ORIENTED_EDGE('',*,*,#11236,.F.);
#16056=ORIENTED_EDGE('',*,*,#11240,.F.);
#16057=ORIENTED_EDGE('',*,*,#11243,.F.);
#16058=ORIENTED_EDGE('',*,*,#11246,.F.);
#16059=ORIENTED_EDGE('',*,*,#11249,.F.);
#16060=ORIENTED_EDGE('',*,*,#11252,.F.);
#16061=ORIENTED_EDGE('',*,*,#11255,.F.);
#16062=ORIENTED_EDGE('',*,*,#11326,.F.);
#16063=ORIENTED_EDGE('',*,*,#11260,.F.);
#16064=ORIENTED_EDGE('',*,*,#11328,.F.);
#16065=ORIENTED_EDGE('',*,*,#11232,.F.);
#16066=ORIENTED_EDGE('',*,*,#11329,.F.);
#16067=ORIENTED_EDGE('',*,*,#11230,.F.);
#16068=ORIENTED_EDGE('',*,*,#11227,.F.);
#16069=ORIENTED_EDGE('',*,*,#11224,.F.);
#16070=ORIENTED_EDGE('',*,*,#11221,.F.);
#16071=ORIENTED_EDGE('',*,*,#11218,.F.);
#16072=ORIENTED_EDGE('',*,*,#11215,.F.);
#16073=ORIENTED_EDGE('',*,*,#11212,.F.);
#16074=ORIENTED_EDGE('',*,*,#11324,.F.);
#16075=ORIENTED_EDGE('',*,*,#11207,.F.);
#16076=ORIENTED_EDGE('',*,*,#11214,.F.);
#16077=ORIENTED_EDGE('',*,*,#11217,.F.);
#16078=ORIENTED_EDGE('',*,*,#11220,.F.);
#16079=ORIENTED_EDGE('',*,*,#11223,.F.);
#16080=ORIENTED_EDGE('',*,*,#11226,.F.);
#16081=ORIENTED_EDGE('',*,*,#11229,.F.);
#16082=ORIENTED_EDGE('',*,*,#11330,.F.);
#16083=ORIENTED_EDGE('',*,*,#11234,.F.);
#16084=ORIENTED_EDGE('',*,*,#11331,.F.);
#16085=ORIENTED_EDGE('',*,*,#11258,.T.);
#16086=ORIENTED_EDGE('',*,*,#11327,.T.);
#16087=ORIENTED_EDGE('',*,*,#11256,.T.);
#16088=ORIENTED_EDGE('',*,*,#11253,.T.);
#16089=ORIENTED_EDGE('',*,*,#11250,.T.);
#16090=ORIENTED_EDGE('',*,*,#11247,.T.);
#16091=ORIENTED_EDGE('',*,*,#11244,.T.);
#16092=ORIENTED_EDGE('',*,*,#11241,.T.);
#16093=ORIENTED_EDGE('',*,*,#11238,.T.);
#16094=ORIENTED_EDGE('',*,*,#11231,.T.);
#16095=ORIENTED_EDGE('',*,*,#11330,.T.);
#16096=ORIENTED_EDGE('',*,*,#11228,.F.);
#16097=ORIENTED_EDGE('',*,*,#11329,.T.);
#16098=ORIENTED_EDGE('',*,*,#11153,.F.);
#16099=ORIENTED_EDGE('',*,*,#11332,.T.);
#16100=ORIENTED_EDGE('',*,*,#11182,.T.);
#16101=ORIENTED_EDGE('',*,*,#11333,.T.);
#16102=ORIENTED_EDGE('',*,*,#11156,.F.);
#16103=ORIENTED_EDGE('',*,*,#11202,.T.);
#16104=ORIENTED_EDGE('',*,*,#11334,.T.);
#16105=ORIENTED_EDGE('',*,*,#11199,.F.);
#16106=ORIENTED_EDGE('',*,*,#11335,.F.);
#16107=ORIENTED_EDGE('',*,*,#11333,.F.);
#16108=ORIENTED_EDGE('',*,*,#11181,.F.);
#16109=ORIENTED_EDGE('',*,*,#11185,.F.);
#16110=ORIENTED_EDGE('',*,*,#11188,.F.);
#16111=ORIENTED_EDGE('',*,*,#11191,.F.);
#16112=ORIENTED_EDGE('',*,*,#11194,.F.);
#16113=ORIENTED_EDGE('',*,*,#11197,.F.);
#16114=ORIENTED_EDGE('',*,*,#11200,.F.);
#16115=ORIENTED_EDGE('',*,*,#11334,.F.);
#16116=ORIENTED_EDGE('',*,*,#11205,.F.);
#16117=ORIENTED_EDGE('',*,*,#11336,.F.);
#16118=ORIENTED_EDGE('',*,*,#11177,.F.);
#16119=ORIENTED_EDGE('',*,*,#11337,.F.);
#16120=ORIENTED_EDGE('',*,*,#11175,.F.);
#16121=ORIENTED_EDGE('',*,*,#11172,.F.);
#16122=ORIENTED_EDGE('',*,*,#11169,.F.);
#16123=ORIENTED_EDGE('',*,*,#11166,.F.);
#16124=ORIENTED_EDGE('',*,*,#11163,.F.);
#16125=ORIENTED_EDGE('',*,*,#11160,.F.);
#16126=ORIENTED_EDGE('',*,*,#11157,.F.);
#16127=ORIENTED_EDGE('',*,*,#11332,.F.);
#16128=ORIENTED_EDGE('',*,*,#11152,.F.);
#16129=ORIENTED_EDGE('',*,*,#11159,.F.);
#16130=ORIENTED_EDGE('',*,*,#11162,.F.);
#16131=ORIENTED_EDGE('',*,*,#11165,.F.);
#16132=ORIENTED_EDGE('',*,*,#11168,.F.);
#16133=ORIENTED_EDGE('',*,*,#11171,.F.);
#16134=ORIENTED_EDGE('',*,*,#11174,.F.);
#16135=ORIENTED_EDGE('',*,*,#11338,.F.);
#16136=ORIENTED_EDGE('',*,*,#11179,.F.);
#16137=ORIENTED_EDGE('',*,*,#11339,.F.);
#16138=ORIENTED_EDGE('',*,*,#11203,.T.);
#16139=ORIENTED_EDGE('',*,*,#11335,.T.);
#16140=ORIENTED_EDGE('',*,*,#11201,.T.);
#16141=ORIENTED_EDGE('',*,*,#11198,.T.);
#16142=ORIENTED_EDGE('',*,*,#11195,.T.);
#16143=ORIENTED_EDGE('',*,*,#11192,.T.);
#16144=ORIENTED_EDGE('',*,*,#11189,.T.);
#16145=ORIENTED_EDGE('',*,*,#11186,.T.);
#16146=ORIENTED_EDGE('',*,*,#11183,.T.);
#16147=ORIENTED_EDGE('',*,*,#11176,.T.);
#16148=ORIENTED_EDGE('',*,*,#11338,.T.);
#16149=ORIENTED_EDGE('',*,*,#11173,.F.);
#16150=ORIENTED_EDGE('',*,*,#11337,.T.);
#16151=ORIENTED_EDGE('',*,*,#11210,.F.);
#16152=ORIENTED_EDGE('',*,*,#11155,.F.);
#16153=ORIENTED_EDGE('',*,*,#11265,.F.);
#16154=ORIENTED_EDGE('',*,*,#11340,.F.);
#16155=ORIENTED_EDGE('',*,*,#11341,.F.);
#16156=ORIENTED_EDGE('',*,*,#11341,.T.);
#16157=ORIENTED_EDGE('',*,*,#11342,.F.);
#16158=ORIENTED_EDGE('',*,*,#11343,.T.);
#16159=ORIENTED_EDGE('',*,*,#11344,.T.);
#16160=ORIENTED_EDGE('',*,*,#11343,.F.);
#16161=ORIENTED_EDGE('',*,*,#11342,.T.);
#16162=ORIENTED_EDGE('',*,*,#11323,.T.);
#16163=ORIENTED_EDGE('',*,*,#11288,.T.);
#16164=ORIENTED_EDGE('',*,*,#11320,.T.);
#16165=ORIENTED_EDGE('',*,*,#11314,.T.);
#16166=ORIENTED_EDGE('',*,*,#11331,.T.);
#16167=ORIENTED_EDGE('',*,*,#11233,.T.);
#16168=ORIENTED_EDGE('',*,*,#11328,.T.);
#16169=ORIENTED_EDGE('',*,*,#11259,.T.);
#16170=ORIENTED_EDGE('',*,*,#11339,.T.);
#16171=ORIENTED_EDGE('',*,*,#11178,.T.);
#16172=ORIENTED_EDGE('',*,*,#11336,.T.);
#16173=ORIENTED_EDGE('',*,*,#11204,.T.);
#16174=ORIENTED_EDGE('',*,*,#11340,.T.);
#16175=ORIENTED_EDGE('',*,*,#11344,.F.);
#20064=CYLINDRICAL_SURFACE('',#22702,2.5175);
#20065=CYLINDRICAL_SURFACE('',#22706,2.5175);
#20066=CYLINDRICAL_SURFACE('',#22707,2.5175);
#20067=CYLINDRICAL_SURFACE('',#22708,2.5175);
#20068=CYLINDRICAL_SURFACE('',#22709,2.5175);
#20069=CYLINDRICAL_SURFACE('',#22710,2.5175);
#20070=CYLINDRICAL_SURFACE('',#22711,2.5175);
#20071=CYLINDRICAL_SURFACE('',#22712,2.5175);
#20072=CYLINDRICAL_SURFACE('',#22714,3.0735);
#20073=CYLINDRICAL_SURFACE('',#22716,3.0735);
#20074=CYLINDRICAL_SURFACE('',#22717,3.0735);
#20075=CYLINDRICAL_SURFACE('',#22718,3.0735);
#20076=CYLINDRICAL_SURFACE('',#22719,3.0735);
#20077=CYLINDRICAL_SURFACE('',#22720,3.0735);
#20078=CYLINDRICAL_SURFACE('',#22721,3.0735);
#20079=CYLINDRICAL_SURFACE('',#22722,3.0735);
#20080=CYLINDRICAL_SURFACE('',#22724,2.5175);
#20081=CYLINDRICAL_SURFACE('',#22728,2.5175);
#20082=CYLINDRICAL_SURFACE('',#22729,2.5175);
#20083=CYLINDRICAL_SURFACE('',#22730,2.5175);
#20084=CYLINDRICAL_SURFACE('',#22731,2.5175);
#20085=CYLINDRICAL_SURFACE('',#22732,2.5175);
#20086=CYLINDRICAL_SURFACE('',#22733,2.5175);
#20087=CYLINDRICAL_SURFACE('',#22734,2.5175);
#20088=CYLINDRICAL_SURFACE('',#22736,3.0735);
#20089=CYLINDRICAL_SURFACE('',#22738,3.0735);
#20090=CYLINDRICAL_SURFACE('',#22739,3.0735);
#20091=CYLINDRICAL_SURFACE('',#22740,3.0735);
#20092=CYLINDRICAL_SURFACE('',#22741,3.0735);
#20093=CYLINDRICAL_SURFACE('',#22742,3.0735);
#20094=CYLINDRICAL_SURFACE('',#22743,3.0735);
#20095=CYLINDRICAL_SURFACE('',#22744,3.0735);
#20096=CYLINDRICAL_SURFACE('',#22746,2.5175);
#20097=CYLINDRICAL_SURFACE('',#22750,2.5175);
#20098=CYLINDRICAL_SURFACE('',#22751,2.5175);
#20099=CYLINDRICAL_SURFACE('',#22752,2.5175);
#20100=CYLINDRICAL_SURFACE('',#22753,2.5175);
#20101=CYLINDRICAL_SURFACE('',#22754,2.5175);
#20102=CYLINDRICAL_SURFACE('',#22755,2.5175);
#20103=CYLINDRICAL_SURFACE('',#22756,2.5175);
#20104=CYLINDRICAL_SURFACE('',#22758,3.0735);
#20105=CYLINDRICAL_SURFACE('',#22760,3.0735);
#20106=CYLINDRICAL_SURFACE('',#22761,3.0735);
#20107=CYLINDRICAL_SURFACE('',#22762,3.0735);
#20108=CYLINDRICAL_SURFACE('',#22763,3.0735);
#20109=CYLINDRICAL_SURFACE('',#22764,3.0735);
#20110=CYLINDRICAL_SURFACE('',#22765,3.0735);
#20111=CYLINDRICAL_SURFACE('',#22766,3.0735);
#20112=CYLINDRICAL_SURFACE('',#22769,3.0735);
#20113=CYLINDRICAL_SURFACE('',#22770,2.5175);
#20114=CYLINDRICAL_SURFACE('',#22772,3.0735);
#20115=CYLINDRICAL_SURFACE('',#22773,2.5175);
#20116=CYLINDRICAL_SURFACE('',#22775,3.0735);
#20117=CYLINDRICAL_SURFACE('',#22776,2.5175);
#20118=CYLINDRICAL_SURFACE('',#22783,30.);
#21128=ADVANCED_FACE('',(#3008),#20064,.F.);
#21129=ADVANCED_FACE('',(#3009),#20065,.F.);
#21130=ADVANCED_FACE('',(#3010),#20066,.F.);
#21131=ADVANCED_FACE('',(#3011),#20067,.F.);
#21132=ADVANCED_FACE('',(#3012),#20068,.F.);
#21133=ADVANCED_FACE('',(#3013),#20069,.F.);
#21134=ADVANCED_FACE('',(#3014),#20070,.F.);
#21135=ADVANCED_FACE('',(#3015),#20071,.F.);
#21136=ADVANCED_FACE('',(#3016),#20072,.F.);
#21137=ADVANCED_FACE('',(#3017),#20073,.F.);
#21138=ADVANCED_FACE('',(#3018),#20074,.F.);
#21139=ADVANCED_FACE('',(#3019),#20075,.F.);
#21140=ADVANCED_FACE('',(#3020),#20076,.F.);
#21141=ADVANCED_FACE('',(#3021),#20077,.F.);
#21142=ADVANCED_FACE('',(#3022),#20078,.F.);
#21143=ADVANCED_FACE('',(#3023),#20079,.F.);
#21144=ADVANCED_FACE('',(#3024),#20080,.F.);
#21145=ADVANCED_FACE('',(#3025),#20081,.F.);
#21146=ADVANCED_FACE('',(#3026),#20082,.F.);
#21147=ADVANCED_FACE('',(#3027),#20083,.F.);
#21148=ADVANCED_FACE('',(#3028),#20084,.F.);
#21149=ADVANCED_FACE('',(#3029),#20085,.F.);
#21150=ADVANCED_FACE('',(#3030),#20086,.F.);
#21151=ADVANCED_FACE('',(#3031),#20087,.F.);
#21152=ADVANCED_FACE('',(#3032),#20088,.F.);
#21153=ADVANCED_FACE('',(#3033),#20089,.F.);
#21154=ADVANCED_FACE('',(#3034),#20090,.F.);
#21155=ADVANCED_FACE('',(#3035),#20091,.F.);
#21156=ADVANCED_FACE('',(#3036),#20092,.F.);
#21157=ADVANCED_FACE('',(#3037),#20093,.F.);
#21158=ADVANCED_FACE('',(#3038),#20094,.F.);
#21159=ADVANCED_FACE('',(#3039),#20095,.F.);
#21160=ADVANCED_FACE('',(#3040),#20096,.F.);
#21161=ADVANCED_FACE('',(#3041),#20097,.F.);
#21162=ADVANCED_FACE('',(#3042),#20098,.F.);
#21163=ADVANCED_FACE('',(#3043),#20099,.F.);
#21164=ADVANCED_FACE('',(#3044),#20100,.F.);
#21165=ADVANCED_FACE('',(#3045),#20101,.F.);
#21166=ADVANCED_FACE('',(#3046),#20102,.F.);
#21167=ADVANCED_FACE('',(#3047),#20103,.F.);
#21168=ADVANCED_FACE('',(#3048),#20104,.F.);
#21169=ADVANCED_FACE('',(#3049),#20105,.F.);
#21170=ADVANCED_FACE('',(#3050),#20106,.F.);
#21171=ADVANCED_FACE('',(#3051),#20107,.F.);
#21172=ADVANCED_FACE('',(#3052),#20108,.F.);
#21173=ADVANCED_FACE('',(#3053),#20109,.F.);
#21174=ADVANCED_FACE('',(#3054),#20110,.F.);
#21175=ADVANCED_FACE('',(#3055),#20111,.F.);
#21176=ADVANCED_FACE('',(#3056),#2478,.T.);
#21177=ADVANCED_FACE('',(#3057),#20112,.F.);
#21178=ADVANCED_FACE('',(#3058),#350,.F.);
#21179=ADVANCED_FACE('',(#3059),#351,.F.);
#21180=ADVANCED_FACE('',(#3060),#20113,.F.);
#21181=ADVANCED_FACE('',(#3061),#2479,.T.);
#21182=ADVANCED_FACE('',(#3062),#20114,.F.);
#21183=ADVANCED_FACE('',(#3063),#352,.F.);
#21184=ADVANCED_FACE('',(#3064),#353,.F.);
#21185=ADVANCED_FACE('',(#3065),#20115,.F.);
#21186=ADVANCED_FACE('',(#3066),#2480,.T.);
#21187=ADVANCED_FACE('',(#3067),#20116,.F.);
#21188=ADVANCED_FACE('',(#3068),#354,.F.);
#21189=ADVANCED_FACE('',(#3069),#355,.F.);
#21190=ADVANCED_FACE('',(#3070),#20117,.F.);
#21191=ADVANCED_FACE('',(#3071),#2481,.F.);
#21192=ADVANCED_FACE('',(#3072),#2482,.F.);
#21193=ADVANCED_FACE('',(#3073),#2483,.F.);
#21194=ADVANCED_FACE('',(#3074),#11,.F.);
#21195=ADVANCED_FACE('',(#3075),#20118,.T.);
#21196=ADVANCED_FACE('',(#3076,#2341,#2342,#2343,#2344),#2484,.T.);
#21197=ADVANCED_FACE('',(#3077),#2485,.F.);
#21820=CLOSED_SHELL('',(#21128,#21129,#21130,#21131,#21132,#21133,#21134,
#21135,#21136,#21137,#21138,#21139,#21140,#21141,#21142,#21143,#21144,#21145,
#21146,#21147,#21148,#21149,#21150,#21151,#21152,#21153,#21154,#21155,#21156,
#21157,#21158,#21159,#21160,#21161,#21162,#21163,#21164,#21165,#21166,#21167,
#21168,#21169,#21170,#21171,#21172,#21173,#21174,#21175,#21176,#21177,#21178,
#21179,#21180,#21181,#21182,#21183,#21184,#21185,#21186,#21187,#21188,#21189,
#21190,#21191,#21192,#21193,#21194,#21195,#21196,#21197));
#22701=AXIS2_PLACEMENT_3D('',#56452,#25382,#25383);
#22702=AXIS2_PLACEMENT_3D('',#56453,#25384,#25385);
#22703=AXIS2_PLACEMENT_3D('',#56463,#25387,#25388);
#22704=AXIS2_PLACEMENT_3D('',#56466,#25390,#25391);
#22705=AXIS2_PLACEMENT_3D('',#56468,#25392,#25393);
#22706=AXIS2_PLACEMENT_3D('',#56479,#25394,#25395);
#22707=AXIS2_PLACEMENT_3D('',#56530,#25397,#25398);
#22708=AXIS2_PLACEMENT_3D('',#56581,#25400,#25401);
#22709=AXIS2_PLACEMENT_3D('',#56629,#25403,#25404);
#22710=AXIS2_PLACEMENT_3D('',#56680,#25406,#25407);
#22711=AXIS2_PLACEMENT_3D('',#56731,#25409,#25410);
#22712=AXIS2_PLACEMENT_3D('',#56779,#25412,#25413);
#22713=AXIS2_PLACEMENT_3D('',#56798,#25415,#25416);
#22714=AXIS2_PLACEMENT_3D('',#56818,#25417,#25418);
#22715=AXIS2_PLACEMENT_3D('',#56832,#25420,#25421);
#22716=AXIS2_PLACEMENT_3D('',#56842,#25422,#25423);
#22717=AXIS2_PLACEMENT_3D('',#56866,#25425,#25426);
#22718=AXIS2_PLACEMENT_3D('',#56891,#25428,#25429);
#22719=AXIS2_PLACEMENT_3D('',#56916,#25431,#25432);
#22720=AXIS2_PLACEMENT_3D('',#56940,#25434,#25435);
#22721=AXIS2_PLACEMENT_3D('',#56965,#25437,#25438);
#22722=AXIS2_PLACEMENT_3D('',#56990,#25440,#25441);
#22723=AXIS2_PLACEMENT_3D('',#57001,#25443,#25444);
#22724=AXIS2_PLACEMENT_3D('',#57007,#25445,#25446);
#22725=AXIS2_PLACEMENT_3D('',#57017,#25448,#25449);
#22726=AXIS2_PLACEMENT_3D('',#57020,#25451,#25452);
#22727=AXIS2_PLACEMENT_3D('',#57022,#25453,#25454);
#22728=AXIS2_PLACEMENT_3D('',#57033,#25455,#25456);
#22729=AXIS2_PLACEMENT_3D('',#57084,#25458,#25459);
#22730=AXIS2_PLACEMENT_3D('',#57135,#25461,#25462);
#22731=AXIS2_PLACEMENT_3D('',#57183,#25464,#25465);
#22732=AXIS2_PLACEMENT_3D('',#57234,#25467,#25468);
#22733=AXIS2_PLACEMENT_3D('',#57285,#25470,#25471);
#22734=AXIS2_PLACEMENT_3D('',#57333,#25473,#25474);
#22735=AXIS2_PLACEMENT_3D('',#57352,#25476,#25477);
#22736=AXIS2_PLACEMENT_3D('',#57372,#25478,#25479);
#22737=AXIS2_PLACEMENT_3D('',#57386,#25481,#25482);
#22738=AXIS2_PLACEMENT_3D('',#57396,#25483,#25484);
#22739=AXIS2_PLACEMENT_3D('',#57420,#25486,#25487);
#22740=AXIS2_PLACEMENT_3D('',#57445,#25489,#25490);
#22741=AXIS2_PLACEMENT_3D('',#57470,#25492,#25493);
#22742=AXIS2_PLACEMENT_3D('',#57494,#25495,#25496);
#22743=AXIS2_PLACEMENT_3D('',#57519,#25498,#25499);
#22744=AXIS2_PLACEMENT_3D('',#57544,#25501,#25502);
#22745=AXIS2_PLACEMENT_3D('',#57555,#25504,#25505);
#22746=AXIS2_PLACEMENT_3D('',#57561,#25506,#25507);
#22747=AXIS2_PLACEMENT_3D('',#57571,#25509,#25510);
#22748=AXIS2_PLACEMENT_3D('',#57574,#25512,#25513);
#22749=AXIS2_PLACEMENT_3D('',#57576,#25514,#25515);
#22750=AXIS2_PLACEMENT_3D('',#57587,#25516,#25517);
#22751=AXIS2_PLACEMENT_3D('',#57638,#25519,#25520);
#22752=AXIS2_PLACEMENT_3D('',#57689,#25522,#25523);
#22753=AXIS2_PLACEMENT_3D('',#57737,#25525,#25526);
#22754=AXIS2_PLACEMENT_3D('',#57788,#25528,#25529);
#22755=AXIS2_PLACEMENT_3D('',#57839,#25531,#25532);
#22756=AXIS2_PLACEMENT_3D('',#57887,#25534,#25535);
#22757=AXIS2_PLACEMENT_3D('',#57906,#25537,#25538);
#22758=AXIS2_PLACEMENT_3D('',#57926,#25539,#25540);
#22759=AXIS2_PLACEMENT_3D('',#57940,#25542,#25543);
#22760=AXIS2_PLACEMENT_3D('',#57950,#25544,#25545);
#22761=AXIS2_PLACEMENT_3D('',#57974,#25547,#25548);
#22762=AXIS2_PLACEMENT_3D('',#57999,#25550,#25551);
#22763=AXIS2_PLACEMENT_3D('',#58024,#25553,#25554);
#22764=AXIS2_PLACEMENT_3D('',#58048,#25556,#25557);
#22765=AXIS2_PLACEMENT_3D('',#58073,#25559,#25560);
#22766=AXIS2_PLACEMENT_3D('',#58098,#25562,#25563);
#22767=AXIS2_PLACEMENT_3D('',#58109,#25565,#25566);
#22768=AXIS2_PLACEMENT_3D('',#58115,#25567,#25568);
#22769=AXIS2_PLACEMENT_3D('',#58307,#25569,#25570);
#22770=AXIS2_PLACEMENT_3D('',#59006,#25571,#25572);
#22771=AXIS2_PLACEMENT_3D('',#59007,#25573,#25574);
#22772=AXIS2_PLACEMENT_3D('',#59199,#25575,#25576);
#22773=AXIS2_PLACEMENT_3D('',#59898,#25577,#25578);
#22774=AXIS2_PLACEMENT_3D('',#59899,#25579,#25580);
#22775=AXIS2_PLACEMENT_3D('',#60091,#25581,#25582);
#22776=AXIS2_PLACEMENT_3D('',#60790,#25583,#25584);
#22777=AXIS2_PLACEMENT_3D('',#60791,#25585,#25586);
#22778=AXIS2_PLACEMENT_3D('',#60792,#25587,#25588);
#22779=AXIS2_PLACEMENT_3D('',#60793,#25589,#25590);
#22780=AXIS2_PLACEMENT_3D('',#60794,#25591,#25592);
#22781=AXIS2_PLACEMENT_3D('',#60796,#25593,#25594);
#22782=AXIS2_PLACEMENT_3D('',#60798,#25595,#25596);
#22783=AXIS2_PLACEMENT_3D('',#60799,#25597,#25598);
#22784=AXIS2_PLACEMENT_3D('',#60801,#25599,#25600);
#22785=AXIS2_PLACEMENT_3D('',#60804,#25602,#25603);
#22786=AXIS2_PLACEMENT_3D('',#60805,#25604,#25605);
#22787=AXIS2_PLACEMENT_3D('',#60806,#25606,#25607);
#25382=DIRECTION('axis',(0.,0.,1.));
#25383=DIRECTION('refdir',(1.,0.,0.));
#25384=DIRECTION('center_axis',(0.,0.,-1.));
#25385=DIRECTION('ref_axis',(1.,0.,0.));
#25386=DIRECTION('',(0.,0.,-1.));
#25387=DIRECTION('center_axis',(0.,0.,1.));
#25388=DIRECTION('ref_axis',(1.,0.,0.));
#25389=DIRECTION('',(0.,0.,-1.));
#25390=DIRECTION('center_axis',(0.,0.,1.));
#25391=DIRECTION('ref_axis',(1.,0.,0.));
#25392=DIRECTION('center_axis',(0.,0.,1.));
#25393=DIRECTION('ref_axis',(1.,0.,0.));
#25394=DIRECTION('center_axis',(0.,0.,-1.));
#25395=DIRECTION('ref_axis',(1.,0.,0.));
#25396=DIRECTION('',(0.,0.,-1.));
#25397=DIRECTION('center_axis',(0.,0.,-1.));
#25398=DIRECTION('ref_axis',(1.,0.,0.));
#25399=DIRECTION('',(0.,0.,-1.));
#25400=DIRECTION('center_axis',(0.,0.,-1.));
#25401=DIRECTION('ref_axis',(1.,0.,0.));
#25402=DIRECTION('',(0.,0.,-1.));
#25403=DIRECTION('center_axis',(0.,0.,-1.));
#25404=DIRECTION('ref_axis',(1.,0.,0.));
#25405=DIRECTION('',(0.,0.,-1.));
#25406=DIRECTION('center_axis',(0.,0.,-1.));
#25407=DIRECTION('ref_axis',(1.,0.,0.));
#25408=DIRECTION('',(0.,0.,-1.));
#25409=DIRECTION('center_axis',(0.,0.,-1.));
#25410=DIRECTION('ref_axis',(1.,0.,0.));
#25411=DIRECTION('',(0.,0.,-1.));
#25412=DIRECTION('center_axis',(0.,0.,-1.));
#25413=DIRECTION('ref_axis',(0.937997876463511,-0.346641001253376,0.));
#25414=DIRECTION('',(0.,0.,-1.));
#25415=DIRECTION('center_axis',(0.,0.,-1.));
#25416=DIRECTION('ref_axis',(1.,0.,0.));
#25417=DIRECTION('center_axis',(0.,0.,-1.));
#25418=DIRECTION('ref_axis',(0.793233502010203,0.608917573476599,0.));
#25419=DIRECTION('',(1.22464679914735E-16,-2.67208401572961E-30,-1.));
#25420=DIRECTION('center_axis',(0.,0.,1.));
#25421=DIRECTION('ref_axis',(1.,-2.16967571364491E-14,0.));
#25422=DIRECTION('center_axis',(0.,0.,-1.));
#25423=DIRECTION('ref_axis',(1.,-2.16967571364491E-14,0.));
#25424=DIRECTION('',(1.22464679914735E-16,-2.67208401572961E-30,-1.));
#25425=DIRECTION('center_axis',(0.,0.,-1.));
#25426=DIRECTION('ref_axis',(1.,-2.16967571364491E-14,0.));
#25427=DIRECTION('',(1.22464679914735E-16,-2.67208401572961E-30,-1.));
#25428=DIRECTION('center_axis',(0.,0.,-1.));
#25429=DIRECTION('ref_axis',(1.,-2.16967571364491E-14,0.));
#25430=DIRECTION('',(1.22464679914735E-16,-2.67208401572961E-30,-1.));
#25431=DIRECTION('center_axis',(0.,0.,-1.));
#25432=DIRECTION('ref_axis',(1.,-2.16967571364491E-14,0.));
#25433=DIRECTION('',(1.22464679914735E-16,-2.67208401572961E-30,-1.));
#25434=DIRECTION('center_axis',(0.,0.,-1.));
#25435=DIRECTION('ref_axis',(1.,-2.16967571364491E-14,0.));
#25436=DIRECTION('',(1.22464679914735E-16,-2.67208401572961E-30,-1.));
#25437=DIRECTION('center_axis',(0.,0.,-1.));
#25438=DIRECTION('ref_axis',(1.,-2.16967571364491E-14,0.));
#25439=DIRECTION('',(1.22464679914735E-16,-2.67208401572961E-30,-1.));
#25440=DIRECTION('center_axis',(0.,0.,-1.));
#25441=DIRECTION('ref_axis',(-0.609100172155653,-0.793093298597305,0.));
#25442=DIRECTION('',(1.22464679914735E-16,-2.67208401572961E-30,-1.));
#25443=DIRECTION('center_axis',(0.,0.,-1.));
#25444=DIRECTION('ref_axis',(1.,-2.16967571364491E-14,0.));
#25445=DIRECTION('center_axis',(0.,0.,-1.));
#25446=DIRECTION('ref_axis',(1.,0.,0.));
#25447=DIRECTION('',(0.,0.,-1.));
#25448=DIRECTION('center_axis',(0.,0.,1.));
#25449=DIRECTION('ref_axis',(1.,0.,0.));
#25450=DIRECTION('',(0.,0.,-1.));
#25451=DIRECTION('center_axis',(0.,0.,1.));
#25452=DIRECTION('ref_axis',(1.,0.,0.));
#25453=DIRECTION('center_axis',(0.,0.,1.));
#25454=DIRECTION('ref_axis',(1.,0.,0.));
#25455=DIRECTION('center_axis',(0.,0.,-1.));
#25456=DIRECTION('ref_axis',(1.,0.,0.));
#25457=DIRECTION('',(0.,0.,-1.));
#25458=DIRECTION('center_axis',(0.,0.,-1.));
#25459=DIRECTION('ref_axis',(1.,0.,0.));
#25460=DIRECTION('',(0.,0.,-1.));
#25461=DIRECTION('center_axis',(0.,0.,-1.));
#25462=DIRECTION('ref_axis',(1.,0.,0.));
#25463=DIRECTION('',(0.,0.,-1.));
#25464=DIRECTION('center_axis',(0.,0.,-1.));
#25465=DIRECTION('ref_axis',(1.,0.,0.));
#25466=DIRECTION('',(0.,0.,-1.));
#25467=DIRECTION('center_axis',(0.,0.,-1.));
#25468=DIRECTION('ref_axis',(1.,0.,0.));
#25469=DIRECTION('',(0.,0.,-1.));
#25470=DIRECTION('center_axis',(0.,0.,-1.));
#25471=DIRECTION('ref_axis',(1.,0.,0.));
#25472=DIRECTION('',(0.,0.,-1.));
#25473=DIRECTION('center_axis',(0.,0.,-1.));
#25474=DIRECTION('ref_axis',(0.937998514609972,-0.346639274447495,0.));
#25475=DIRECTION('',(0.,0.,-1.));
#25476=DIRECTION('center_axis',(0.,0.,-1.));
#25477=DIRECTION('ref_axis',(1.,0.,0.));
#25478=DIRECTION('center_axis',(0.,0.,-1.));
#25479=DIRECTION('ref_axis',(0.793234421148473,0.608916376118468,0.));
#25480=DIRECTION('',(1.22464679914735E-16,-2.66923102573661E-30,-1.));
#25481=DIRECTION('center_axis',(0.,0.,1.));
#25482=DIRECTION('ref_axis',(1.,-2.16734607052251E-14,0.));
#25483=DIRECTION('center_axis',(0.,0.,-1.));
#25484=DIRECTION('ref_axis',(1.,-2.16734607052251E-14,0.));
#25485=DIRECTION('',(1.22464679914735E-16,-2.66923102573661E-30,-1.));
#25486=DIRECTION('center_axis',(0.,0.,-1.));
#25487=DIRECTION('ref_axis',(1.,-2.16734607052251E-14,0.));
#25488=DIRECTION('',(1.22464679914735E-16,-2.66923102573661E-30,-1.));
#25489=DIRECTION('center_axis',(0.,0.,-1.));
#25490=DIRECTION('ref_axis',(1.,-2.16734607052251E-14,0.));
#25491=DIRECTION('',(1.22464679914735E-16,-2.66923102573661E-30,-1.));
#25492=DIRECTION('center_axis',(0.,0.,-1.));
#25493=DIRECTION('ref_axis',(1.,-2.16734607052251E-14,0.));
#25494=DIRECTION('',(1.22464679914735E-16,-2.66923102573661E-30,-1.));
#25495=DIRECTION('center_axis',(0.,0.,-1.));
#25496=DIRECTION('ref_axis',(1.,-2.16734607052251E-14,0.));
#25497=DIRECTION('',(1.22464679914735E-16,-2.66923102573661E-30,-1.));
#25498=DIRECTION('center_axis',(0.,0.,-1.));
#25499=DIRECTION('ref_axis',(1.,-2.16734607052251E-14,0.));
#25500=DIRECTION('',(1.22464679914735E-16,-2.66923102573661E-30,-1.));
#25501=DIRECTION('center_axis',(0.,0.,-1.));
#25502=DIRECTION('ref_axis',(-0.609099316811134,-0.793093955506036,0.));
#25503=DIRECTION('',(1.22464679914735E-16,-2.66923102573661E-30,-1.));
#25504=DIRECTION('center_axis',(0.,0.,-1.));
#25505=DIRECTION('ref_axis',(1.,-2.16734607052251E-14,0.));
#25506=DIRECTION('center_axis',(0.,0.,-1.));
#25507=DIRECTION('ref_axis',(1.,0.,0.));
#25508=DIRECTION('',(0.,0.,-1.));
#25509=DIRECTION('center_axis',(0.,0.,1.));
#25510=DIRECTION('ref_axis',(1.,0.,0.));
#25511=DIRECTION('',(0.,0.,-1.));
#25512=DIRECTION('center_axis',(0.,0.,1.));
#25513=DIRECTION('ref_axis',(1.,0.,0.));
#25514=DIRECTION('center_axis',(0.,0.,1.));
#25515=DIRECTION('ref_axis',(1.,0.,0.));
#25516=DIRECTION('center_axis',(0.,0.,-1.));
#25517=DIRECTION('ref_axis',(1.,0.,0.));
#25518=DIRECTION('',(0.,0.,-1.));
#25519=DIRECTION('center_axis',(0.,0.,-1.));
#25520=DIRECTION('ref_axis',(1.,0.,0.));
#25521=DIRECTION('',(0.,0.,-1.));
#25522=DIRECTION('center_axis',(0.,0.,-1.));
#25523=DIRECTION('ref_axis',(1.,0.,0.));
#25524=DIRECTION('',(0.,0.,-1.));
#25525=DIRECTION('center_axis',(0.,0.,-1.));
#25526=DIRECTION('ref_axis',(1.,0.,0.));
#25527=DIRECTION('',(0.,0.,-1.));
#25528=DIRECTION('center_axis',(0.,0.,-1.));
#25529=DIRECTION('ref_axis',(1.,0.,0.));
#25530=DIRECTION('',(0.,0.,-1.));
#25531=DIRECTION('center_axis',(0.,0.,-1.));
#25532=DIRECTION('ref_axis',(1.,0.,0.));
#25533=DIRECTION('',(0.,0.,-1.));
#25534=DIRECTION('center_axis',(0.,0.,-1.));
#25535=DIRECTION('ref_axis',(0.937998542404131,-0.346639199237082,0.));
#25536=DIRECTION('',(0.,0.,-1.));
#25537=DIRECTION('center_axis',(0.,0.,-1.));
#25538=DIRECTION('ref_axis',(1.,0.,0.));
#25539=DIRECTION('center_axis',(0.,0.,-1.));
#25540=DIRECTION('ref_axis',(0.793234457633775,0.608916328589118,0.));
#25541=DIRECTION('',(1.22464679914735E-16,-2.66923102573661E-30,-1.));
#25542=DIRECTION('center_axis',(0.,0.,1.));
#25543=DIRECTION('ref_axis',(1.,-2.16734607052251E-14,0.));
#25544=DIRECTION('center_axis',(0.,0.,-1.));
#25545=DIRECTION('ref_axis',(1.,-2.16734607052251E-14,0.));
#25546=DIRECTION('',(1.22464679914735E-16,-2.66923102573661E-30,-1.));
#25547=DIRECTION('center_axis',(0.,0.,-1.));
#25548=DIRECTION('ref_axis',(1.,-2.16734607052251E-14,0.));
#25549=DIRECTION('',(1.22464679914735E-16,-2.66923102573661E-30,-1.));
#25550=DIRECTION('center_axis',(0.,0.,-1.));
#25551=DIRECTION('ref_axis',(1.,-2.16734607052251E-14,0.));
#25552=DIRECTION('',(1.22464679914735E-16,-2.66923102573661E-30,-1.));
#25553=DIRECTION('center_axis',(0.,0.,-1.));
#25554=DIRECTION('ref_axis',(1.,-2.16734607052251E-14,0.));
#25555=DIRECTION('',(1.22464679914735E-16,-2.66923102573661E-30,-1.));
#25556=DIRECTION('center_axis',(0.,0.,-1.));
#25557=DIRECTION('ref_axis',(1.,-2.16734607052251E-14,0.));
#25558=DIRECTION('',(1.22464679914735E-16,-2.66923102573661E-30,-1.));
#25559=DIRECTION('center_axis',(0.,0.,-1.));
#25560=DIRECTION('ref_axis',(1.,-2.16734607052251E-14,0.));
#25561=DIRECTION('',(1.22464679914735E-16,-2.66923102573661E-30,-1.));
#25562=DIRECTION('center_axis',(0.,0.,-1.));
#25563=DIRECTION('ref_axis',(-0.609099265708522,-0.793093994753042,0.));
#25564=DIRECTION('',(1.22464679914735E-16,-2.66923102573661E-30,-1.));
#25565=DIRECTION('center_axis',(0.,0.,-1.));
#25566=DIRECTION('ref_axis',(1.,-2.16734607052251E-14,0.));
#25567=DIRECTION('center_axis',(0.,0.,1.));
#25568=DIRECTION('ref_axis',(1.,0.,0.));
#25569=DIRECTION('center_axis',(0.,0.,-1.));
#25570=DIRECTION('ref_axis',(1.,-2.16734607052251E-14,0.));
#25571=DIRECTION('center_axis',(0.,0.,-1.));
#25572=DIRECTION('ref_axis',(1.,0.,0.));
#25573=DIRECTION('center_axis',(0.,0.,1.));
#25574=DIRECTION('ref_axis',(1.,0.,0.));
#25575=DIRECTION('center_axis',(0.,0.,-1.));
#25576=DIRECTION('ref_axis',(1.,-2.16734607052251E-14,0.));
#25577=DIRECTION('center_axis',(0.,0.,-1.));
#25578=DIRECTION('ref_axis',(1.,0.,0.));
#25579=DIRECTION('center_axis',(0.,0.,1.));
#25580=DIRECTION('ref_axis',(1.,0.,0.));
#25581=DIRECTION('center_axis',(0.,0.,-1.));
#25582=DIRECTION('ref_axis',(1.,-2.16967571364491E-14,0.));
#25583=DIRECTION('center_axis',(0.,0.,-1.));
#25584=DIRECTION('ref_axis',(1.,0.,0.));
#25585=DIRECTION('center_axis',(0.,0.,-1.));
#25586=DIRECTION('ref_axis',(1.,0.,0.));
#25587=DIRECTION('center_axis',(0.,0.,-1.));
#25588=DIRECTION('ref_axis',(1.,0.,0.));
#25589=DIRECTION('center_axis',(0.,0.,-1.));
#25590=DIRECTION('ref_axis',(1.,0.,0.));
#25591=DIRECTION('center_axis',(6.12323399573677E-17,0.,1.));
#25592=DIRECTION('ref_axis',(1.,0.,0.));
#25593=DIRECTION('center_axis',(0.,0.,-1.));
#25594=DIRECTION('ref_axis',(0.,1.,0.));
#25595=DIRECTION('center_axis',(-1.22464679914735E-16,1.,0.));
#25596=DIRECTION('ref_axis',(-1.,-1.22464679914735E-16,0.));
#25597=DIRECTION('center_axis',(0.,0.,1.));
#25598=DIRECTION('ref_axis',(1.,0.,0.));
#25599=DIRECTION('center_axis',(0.,0.,1.));
#25600=DIRECTION('ref_axis',(1.,0.,0.));
#25601=DIRECTION('',(0.,0.,-1.));
#25602=DIRECTION('center_axis',(0.,0.,1.));
#25603=DIRECTION('ref_axis',(1.,0.,0.));
#25604=DIRECTION('center_axis',(0.,0.,1.));
#25605=DIRECTION('ref_axis',(1.,0.,0.));
#25606=DIRECTION('center_axis',(0.,0.,1.));
#25607=DIRECTION('ref_axis',(1.,0.,0.));
#56452=CARTESIAN_POINT('',(0.,0.,0.));
#56453=CARTESIAN_POINT('Origin',(15.,0.,7.5));
#56454=CARTESIAN_POINT('',(12.4864520394788,-8.37379766882585E-5,4.38741669750802));
#56455=CARTESIAN_POINT('',(12.4839933051997,-0.00316412607611227,4.11258330249198));
#56456=CARTESIAN_POINT('',(12.4825,3.08304831685346E-16,7.5));
#56457=CARTESIAN_POINT('',(13.086534003335,1.63598720337497,4.));
#56458=CARTESIAN_POINT('Ctrl Pts',(12.4839933051997,-0.00316412607611227,
4.11258330249198));
#56459=CARTESIAN_POINT('Ctrl Pts',(12.4891843965477,0.589325119423629,4.07505553499466));
#56460=CARTESIAN_POINT('Ctrl Pts',(12.700778171916,1.18480356030443,4.03752776749733));
#56461=CARTESIAN_POINT('Ctrl Pts',(13.086534003335,1.63598720337497,4.));
#56462=CARTESIAN_POINT('',(12.4825,3.08304831685346E-16,4.));
#56463=CARTESIAN_POINT('Origin',(15.,0.,4.));
#56464=CARTESIAN_POINT('',(12.4825,-3.08304831685346E-16,3.));
#56465=CARTESIAN_POINT('',(12.4825,3.08304831685346E-16,7.5));
#56466=CARTESIAN_POINT('Origin',(15.,0.,3.));
#56467=CARTESIAN_POINT('',(16.9169900003259,1.63831767401966,4.));
#56468=CARTESIAN_POINT('Origin',(15.,0.,4.));
#56469=CARTESIAN_POINT('Ctrl Pts',(16.9170033607455,1.63832650944338,4.));
#56470=CARTESIAN_POINT('Ctrl Pts',(16.4032792982694,2.23546892087832,4.04999787746244));
#56471=CARTESIAN_POINT('Ctrl Pts',(15.5859097998096,2.57572249729409,4.09999575492489));
#56472=CARTESIAN_POINT('Ctrl Pts',(14.8008208232653,2.51338129467797,4.14999363238733));
#56473=CARTESIAN_POINT('Ctrl Pts',(13.9790588101819,2.44812801296032,4.20232700817141));
#56474=CARTESIAN_POINT('Ctrl Pts',(13.1926635275253,1.94178951401471,4.2546603839555));
#56475=CARTESIAN_POINT('Ctrl Pts',(12.7937453701095,1.22068434196769,4.30699375973958));
#56476=CARTESIAN_POINT('Ctrl Pts',(12.5894005030727,0.851299951304611,4.3338014056624));
#56477=CARTESIAN_POINT('Ctrl Pts',(12.4867287035022,0.425561301199251,4.36060905158521));
#56478=CARTESIAN_POINT('Ctrl Pts',(12.4864520394788,-8.37379766882585E-5,
4.38741669750802));
#56479=CARTESIAN_POINT('Origin',(15.,0.,7.5));
#56480=CARTESIAN_POINT('',(12.4798657694311,-0.00154038945686864,5.38741669750803));
#56481=CARTESIAN_POINT('',(12.4793021139561,0.00120904389216911,5.11258330249198));
#56482=CARTESIAN_POINT('',(12.4825,3.08304831685346E-16,7.5));
#56483=CARTESIAN_POINT('Ctrl Pts',(12.4793021139561,0.00120904389216911,
5.11258330249198));
#56484=CARTESIAN_POINT('Ctrl Pts',(12.478879906904,0.0725686704440801,5.10805583214991));
#56485=CARTESIAN_POINT('Ctrl Pts',(12.4816538040259,0.14389470397244,5.10352836180784));
#56486=CARTESIAN_POINT('Ctrl Pts',(12.4877315613661,0.214937734438189,5.09900089146578));
#56487=CARTESIAN_POINT('Ctrl Pts',(12.5579848230722,1.0361295544392,5.04666751568169));
#56488=CARTESIAN_POINT('Ctrl Pts',(13.0696742764471,1.81950869898314,4.99433413989761));
#56489=CARTESIAN_POINT('Ctrl Pts',(13.7933805800141,2.21395750784665,4.94200076411352));
#56490=CARTESIAN_POINT('Ctrl Pts',(14.5170868835811,2.60840631671017,4.88966738832944));
#56491=CARTESIAN_POINT('Ctrl Pts',(15.4528100373402,2.61392478989326,4.83733401254535));
#56492=CARTESIAN_POINT('Ctrl Pts',(16.1810158838377,2.22781637405164,4.78500063676127));
#56493=CARTESIAN_POINT('Ctrl Pts',(16.9092217303351,1.84170795821001,4.73266726097718));
#56494=CARTESIAN_POINT('Ctrl Pts',(17.4299102695709,1.06397265334366,4.6803338851931));
#56495=CARTESIAN_POINT('Ctrl Pts',(17.5096246317311,0.243745210316159,4.62800050940901));
#56496=CARTESIAN_POINT('Ctrl Pts',(17.5893389938914,-0.576482232711353,
4.57566713362493));
#56497=CARTESIAN_POINT('Ctrl Pts',(17.2280791789763,-1.43920181390003,4.52333375784085));
#56498=CARTESIAN_POINT('Ctrl Pts',(16.5878264117224,-1.95845762325597,4.47100038205676));
#56499=CARTESIAN_POINT('Ctrl Pts',(15.9475736444685,-2.47771343261192,4.41866700627268));
#56500=CARTESIAN_POINT('Ctrl Pts',(15.0283279248759,-2.65350547013512,4.36633363048859));
#56501=CARTESIAN_POINT('Ctrl Pts',(14.2422049662735,-2.40531717421469,4.3140002547045));
#56502=CARTESIAN_POINT('Ctrl Pts',(13.4560820076711,-2.15712887829427,4.26166687892042));
#56503=CARTESIAN_POINT('Ctrl Pts',(12.8030818100589,-1.48496024893023,4.20933350313634));
#56504=CARTESIAN_POINT('Ctrl Pts',(12.5762083591215,-0.69397784322712,4.15700012735226));
#56505=CARTESIAN_POINT('Ctrl Pts',(12.5120237084102,-0.470201419766977,
4.1421945190655));
#56506=CARTESIAN_POINT('Ctrl Pts',(12.4819452946144,-0.236915405941376,
4.12738891077874));
#56507=CARTESIAN_POINT('Ctrl Pts',(12.4839933051997,-0.00316412607611227,
4.11258330249198));
#56508=CARTESIAN_POINT('Ctrl Pts',(12.4864520394788,-8.37379766882585E-5,
4.38741669750802));
#56509=CARTESIAN_POINT('Ctrl Pts',(12.4861886052651,-0.405374837317443,
4.41294242736929));
#56510=CARTESIAN_POINT('Ctrl Pts',(12.5787615741259,-0.810581064443052,
4.43846815723057));
#56511=CARTESIAN_POINT('Ctrl Pts',(12.7647943027407,-1.16697133984538,4.46399388709184));
#56512=CARTESIAN_POINT('Ctrl Pts',(13.146202424963,-1.897650004463,4.51632726287592));
#56513=CARTESIAN_POINT('Ctrl Pts',(13.9204597015827,-2.42313548854983,4.56866063866001));
#56514=CARTESIAN_POINT('Ctrl Pts',(14.7402998673034,-2.50800691661078,4.62099401444409));
#56515=CARTESIAN_POINT('Ctrl Pts',(15.560140033024,-2.59287834467174,4.67332739022818));
#56516=CARTESIAN_POINT('Ctrl Pts',(16.4255630878457,-2.23713571670682,4.72566076601226));
#56517=CARTESIAN_POINT('Ctrl Pts',(16.9486162247073,-1.60018404184685,4.77799414179635));
#56518=CARTESIAN_POINT('Ctrl Pts',(17.471669361569,-0.963232366986897,4.83032751758043));
#56519=CARTESIAN_POINT('Ctrl Pts',(17.6523525804706,-0.0450716452319087,
4.88266089336451));
#56520=CARTESIAN_POINT('Ctrl Pts',(17.4096229743894,0.742588180844264,4.9349942691486));
#56521=CARTESIAN_POINT('Ctrl Pts',(17.1668933683082,1.53024800692044,4.98732764493268));
#56522=CARTESIAN_POINT('Ctrl Pts',(16.5007509372442,2.1874069373178,5.03966102071677));
#56523=CARTESIAN_POINT('Ctrl Pts',(15.7098806230762,2.41944933284425,5.09199439650085));
#56524=CARTESIAN_POINT('Ctrl Pts',(14.9190103089082,2.6514917283707,5.14432777228493));
#56525=CARTESIAN_POINT('Ctrl Pts',(14.0034121116361,2.45841758902623,5.19666114806902));
#56526=CARTESIAN_POINT('Ctrl Pts',(13.3735902615222,1.92677994818613,5.2489945238531));
#56527=CARTESIAN_POINT('Ctrl Pts',(12.8182957469354,1.45805142494902,5.29513524840474));
#56528=CARTESIAN_POINT('Ctrl Pts',(12.4851467735748,0.72614376520494,5.34127597295639));
#56529=CARTESIAN_POINT('Ctrl Pts',(12.4798657694311,-0.00154038945686864,
5.38741669750803));
#56530=CARTESIAN_POINT('Origin',(15.,0.,7.5));
#56531=CARTESIAN_POINT('',(12.482920633805,0.00216662177004473,6.38741669750803));
#56532=CARTESIAN_POINT('',(12.4862854318642,0.000566909999415368,6.11258330249198));
#56533=CARTESIAN_POINT('',(12.4825,3.08304831685346E-16,7.5));
#56534=CARTESIAN_POINT('Ctrl Pts',(12.4862854318642,0.000566909999415368,
6.11258330249198));
#56535=CARTESIAN_POINT('Ctrl Pts',(12.4855058897774,0.379333771915191,6.08872275352109));
#56536=CARTESIAN_POINT('Ctrl Pts',(12.5659381445238,0.757786273313489,6.06486220455019));
#56537=CARTESIAN_POINT('Ctrl Pts',(12.7293101493446,1.09619859491376,6.04100165557929));
#56538=CARTESIAN_POINT('Ctrl Pts',(13.08763419844,1.83843881821599,5.98866827979521));
#56539=CARTESIAN_POINT('Ctrl Pts',(13.8449458114837,2.38806291012985,5.93633490401113));
#56540=CARTESIAN_POINT('Ctrl Pts',(14.6617006772638,2.49864636478707,5.88400152822704));
#56541=CARTESIAN_POINT('Ctrl Pts',(15.4784555430439,2.60922981944428,5.83166815244296));
#56542=CARTESIAN_POINT('Ctrl Pts',(16.3546536615603,2.28077263684485,5.77933477665887));
#56543=CARTESIAN_POINT('Ctrl Pts',(16.8974474362482,1.66053609593171,5.72700140087479));
#56544=CARTESIAN_POINT('Ctrl Pts',(17.4402412109362,1.04029955501857,5.6746680250907));
#56545=CARTESIAN_POINT('Ctrl Pts',(17.6496306417956,0.128283655791723,5.62233464930662));
#56546=CARTESIAN_POINT('Ctrl Pts',(17.4317349092204,-0.66659696383412,5.57000127352254));
#56547=CARTESIAN_POINT('Ctrl Pts',(17.2138391766452,-1.46147758345996,5.51766789773845));
#56548=CARTESIAN_POINT('Ctrl Pts',(16.5686582806354,-2.13922292348481,5.46533452195437));
#56549=CARTESIAN_POINT('Ctrl Pts',(15.7854622951236,-2.39597806232545,5.41300114617028));
#56550=CARTESIAN_POINT('Ctrl Pts',(15.0022663096119,-2.65273320116609,5.3606677703862));
#56551=CARTESIAN_POINT('Ctrl Pts',(14.0810552345983,-2.48849813882253,5.30833439460211));
#56552=CARTESIAN_POINT('Ctrl Pts',(13.4348582321103,-1.9768783599217,5.25600101881803));
#56553=CARTESIAN_POINT('Ctrl Pts',(12.8445650905918,-1.50951988350108,5.20819511337601));
#56554=CARTESIAN_POINT('Ctrl Pts',(12.4837602304949,-0.752282707918894,
5.160389207934));
#56555=CARTESIAN_POINT('Ctrl Pts',(12.4793021139561,0.00120904389216911,
5.11258330249198));
#56556=CARTESIAN_POINT('Ctrl Pts',(12.4798657694311,-0.00154038945686864,
5.38741669750803));
#56557=CARTESIAN_POINT('Ctrl Pts',(12.4791569938941,-0.0992045293459824,
5.39360934874047));
#56558=CARTESIAN_POINT('Ctrl Pts',(12.4843540819724,-0.196792591522919,
5.39980199997291));
#56559=CARTESIAN_POINT('Ctrl Pts',(12.4957126236098,-0.293658114991017,
5.40599465120536));
#56560=CARTESIAN_POINT('Ctrl Pts',(12.5917023387672,-1.11225739499233,5.45832802698944));
#56561=CARTESIAN_POINT('Ctrl Pts',(13.1277272720379,-1.87925481265923,5.51066140277353));
#56562=CARTESIAN_POINT('Ctrl Pts',(13.8634558058795,-2.25076673554666,5.56299477855761));
#56563=CARTESIAN_POINT('Ctrl Pts',(14.5991843397211,-2.62227865843409,5.61532815434169));
#56564=CARTESIAN_POINT('Ctrl Pts',(15.5346164741336,-2.59830508654206,5.66766153012578));
#56565=CARTESIAN_POINT('Ctrl Pts',(16.2503478880118,-2.18959297269902,5.71999490590987));
#56566=CARTESIAN_POINT('Ctrl Pts',(16.96607930189,-1.78088085885597,5.77232828169395));
#56567=CARTESIAN_POINT('Ctrl Pts',(17.4621099952338,-0.98743020306191,5.82466165747803));
#56568=CARTESIAN_POINT('Ctrl Pts',(17.5160416303984,-0.16498929182795,5.87699503326212));
#56569=CARTESIAN_POINT('Ctrl Pts',(17.5699732655631,0.657451619406004,5.9293284090462));
#56570=CARTESIAN_POINT('Ctrl Pts',(17.1818058425485,1.50888278607985,5.98166178483029));
#56571=CARTESIAN_POINT('Ctrl Pts',(16.5255763936941,2.00756141147231,6.03399516061437));
#56572=CARTESIAN_POINT('Ctrl Pts',(15.8693469448397,2.50624003686478,6.08632853639846));
#56573=CARTESIAN_POINT('Ctrl Pts',(14.9450554701454,2.65216612097585,6.13866191218254));
#56574=CARTESIAN_POINT('Ctrl Pts',(14.1671123287709,2.37991277262463,6.19099528796662));
#56575=CARTESIAN_POINT('Ctrl Pts',(13.3891691873965,2.10765942427341,6.24332866375071));
#56576=CARTESIAN_POINT('Ctrl Pts',(12.7575743793418,1.41722664345988,6.2956620395348));
#56577=CARTESIAN_POINT('Ctrl Pts',(12.5555065470498,0.618173398042358,6.34799541531888));
#56578=CARTESIAN_POINT('Ctrl Pts',(12.5047691803197,0.417538506829285,6.36113584271526));
#56579=CARTESIAN_POINT('Ctrl Pts',(12.4811120172555,0.210055467607507,6.37427627011165));
#56580=CARTESIAN_POINT('Ctrl Pts',(12.482920633805,0.00216662177004473,
6.38741669750803));
#56581=CARTESIAN_POINT('Origin',(15.,0.,7.5));
#56582=CARTESIAN_POINT('',(12.4854953774899,-0.00143787083715985,7.38741669750803));
#56583=CARTESIAN_POINT('',(12.4810882026093,-0.00198272270578489,7.11258330249199));
#56584=CARTESIAN_POINT('',(12.4825,3.08304831685346E-16,7.5));
#56585=CARTESIAN_POINT('Ctrl Pts',(12.4810882026093,-0.00198272270578489,
7.11258330249199));
#56586=CARTESIAN_POINT('Ctrl Pts',(12.4869739395021,0.680084118616307,7.06938967489226));
#56587=CARTESIAN_POINT('Ctrl Pts',(12.7744552727444,1.36652561897882,7.02619604729254));
#56588=CARTESIAN_POINT('Ctrl Pts',(13.269118044078,1.83350231786092,6.98300241969281));
#56589=CARTESIAN_POINT('Ctrl Pts',(13.8684511896637,2.39929103307328,6.93066904390873));
#56590=CARTESIAN_POINT('Ctrl Pts',(14.7719211435091,2.64291129119537,6.87833566812465));
#56591=CARTESIAN_POINT('Ctrl Pts',(15.5744528177492,2.45513481925728,6.82600229234056));
#56592=CARTESIAN_POINT('Ctrl Pts',(16.3769844919893,2.26735834731918,6.77366891655648));
#56593=CARTESIAN_POINT('Ctrl Pts',(17.0785778866242,1.64818514532091,6.72133554077239));
#56594=CARTESIAN_POINT('Ctrl Pts',(17.3646702383797,0.875224413728682,6.66900216498831));
#56595=CARTESIAN_POINT('Ctrl Pts',(17.6507625901351,0.102263682136454,6.61666878920422));
#56596=CARTESIAN_POINT('Ctrl Pts',(17.5213538990113,-0.82448457904973,6.56433541342014));
#56597=CARTESIAN_POINT('Ctrl Pts',(17.0344651712476,-1.48950819606356,6.51200203763606));
#56598=CARTESIAN_POINT('Ctrl Pts',(16.547576443484,-2.15453181307739,6.45966866185197));
#56599=CARTESIAN_POINT('Ctrl Pts',(15.7032076790805,-2.55783078591888,6.40733528606789));
#56600=CARTESIAN_POINT('Ctrl Pts',(14.8799356660918,-2.51858436884117,6.3550019102838));
#56601=CARTESIAN_POINT('Ctrl Pts',(14.0566636531032,-2.47933795176346,6.30266853449972));
#56602=CARTESIAN_POINT('Ctrl Pts',(13.2544883915292,-1.99754614476656,6.25033515871564));
#56603=CARTESIAN_POINT('Ctrl Pts',(12.8330690033158,-1.28922206392281,6.19800178293155));
#56604=CARTESIAN_POINT('Ctrl Pts',(12.6037889105156,-0.903846792801687,
6.16952895611836));
#56605=CARTESIAN_POINT('Ctrl Pts',(12.4872156605381,-0.451416121701059,
6.14105612930517));
#56606=CARTESIAN_POINT('Ctrl Pts',(12.4862854318642,0.000566909999415368,
6.11258330249198));
#56607=CARTESIAN_POINT('Ctrl Pts',(12.482920633805,0.00216662177004473,
6.38741669750803));
#56608=CARTESIAN_POINT('Ctrl Pts',(12.488315056143,-0.617887548426095,6.42660964589573));
#56609=CARTESIAN_POINT('Ctrl Pts',(12.7202541571503,-1.24155179185567,6.46580259428343));
#56610=CARTESIAN_POINT('Ctrl Pts',(13.1359015380453,-1.69788793113621,6.50499554267113));
#56611=CARTESIAN_POINT('Ctrl Pts',(13.6909052178623,-2.30722230487577,6.55732891845522));
#56612=CARTESIAN_POINT('Ctrl Pts',(14.5734534340258,-2.61821734233337,6.6096622942393));
#56613=CARTESIAN_POINT('Ctrl Pts',(15.3878514816524,-2.49143689543374,6.66199567002338));
#56614=CARTESIAN_POINT('Ctrl Pts',(16.2022495292791,-2.36465644853411,6.71432904580747));
#56615=CARTESIAN_POINT('Ctrl Pts',(16.9484974083689,-1.80010051727723,6.76666242159155));
#56616=CARTESIAN_POINT('Ctrl Pts',(17.2920112918525,-1.05089047753226,6.81899579737564));
#56617=CARTESIAN_POINT('Ctrl Pts',(17.635525175336,-0.301680437787271,6.87132917315973));
#56618=CARTESIAN_POINT('Ctrl Pts',(17.5763050632133,0.632183710445827,6.92366254894381));
#56619=CARTESIAN_POINT('Ctrl Pts',(17.1409025824082,1.33199950499447,6.97599592472789));
#56620=CARTESIAN_POINT('Ctrl Pts',(16.7055001016032,2.03181529954311,7.02832930051198));
#56621=CARTESIAN_POINT('Ctrl Pts',(15.8939152521159,2.49758274040729,7.08066267629606));
#56622=CARTESIAN_POINT('Ctrl Pts',(15.0700259913432,2.52047275706227,7.13299605208015));
#56623=CARTESIAN_POINT('Ctrl Pts',(14.2461367305706,2.54336277371724,7.18532942786423));
#56624=CARTESIAN_POINT('Ctrl Pts',(13.4099430585124,2.12337536616301,7.23766280364831));
#56625=CARTESIAN_POINT('Ctrl Pts',(12.9363564205467,1.44881390534349,7.2899961794324));
#56626=CARTESIAN_POINT('Ctrl Pts',(12.6424900625863,1.03024018763275,7.32246968545761));
#56627=CARTESIAN_POINT('Ctrl Pts',(12.4882403133338,0.513646402355209,7.35494319148282));
#56628=CARTESIAN_POINT('Ctrl Pts',(12.4854953774899,-0.00143787083715985,
7.38741669750803));
#56629=CARTESIAN_POINT('Origin',(15.,0.,7.5));
#56630=CARTESIAN_POINT('',(12.4785663033905,-0.000147683907944251,8.38741669750803));
#56631=CARTESIAN_POINT('',(12.4815651121962,0.00207920831391662,8.11258330249198));
#56632=CARTESIAN_POINT('',(12.4825,3.08304831685346E-16,7.5));
#56633=CARTESIAN_POINT('Ctrl Pts',(12.4815651121962,0.00207920831391661,
8.11258330249198));
#56634=CARTESIAN_POINT('Ctrl Pts',(12.4801423769425,0.163120151964822,8.10238997204752));
#56635=CARTESIAN_POINT('Ctrl Pts',(12.4942993050251,0.323912101526709,8.09219664160305));
#56636=CARTESIAN_POINT('Ctrl Pts',(12.524955296352,0.48149432911561,8.08200331115859));
#56637=CARTESIAN_POINT('Ctrl Pts',(12.6823456137647,1.29053412020584,8.0296699353745));
#56638=CARTESIAN_POINT('Ctrl Pts',(13.27463109749,2.01496955827445,7.97733655959042));
#56639=CARTESIAN_POINT('Ctrl Pts',(14.036257709891,2.32999653926404,7.92500318380634));
#56640=CARTESIAN_POINT('Ctrl Pts',(14.797884322292,2.64502352025364,7.87266980802225));
#56641=CARTESIAN_POINT('Ctrl Pts',(15.7288520633688,2.55064204416424,7.82033643223817));
#56642=CARTESIAN_POINT('Ctrl Pts',(16.4117570807264,2.08916849927148,7.76800305645408));
#56643=CARTESIAN_POINT('Ctrl Pts',(17.0946620980841,1.62769495437873,7.71566968067));
#56644=CARTESIAN_POINT('Ctrl Pts',(17.5295043917226,0.799129340682624,7.66333630488591));
#56645=CARTESIAN_POINT('Ctrl Pts',(17.5213203334702,-0.0250369758568184,
7.61100292910183));
#56646=CARTESIAN_POINT('Ctrl Pts',(17.5131362752179,-0.849203292396252,
7.55866955331774));
#56647=CARTESIAN_POINT('Ctrl Pts',(17.0619258650746,-1.66897031177902,7.50633617753366));
#56648=CARTESIAN_POINT('Ctrl Pts',(16.3699914547578,-2.11679155594354,7.45400280174958));
#56649=CARTESIAN_POINT('Ctrl Pts',(15.678057044441,-2.56461280010805,7.4016694259655));
#56650=CARTESIAN_POINT('Ctrl Pts',(14.7453986339507,-2.6404882690543,7.34933605018141));
#56651=CARTESIAN_POINT('Ctrl Pts',(13.9901780954356,-2.31039883752012,7.29700267439732));
#56652=CARTESIAN_POINT('Ctrl Pts',(13.2349575569204,-1.98030940598595,7.24466929861324));
#56653=CARTESIAN_POINT('Ctrl Pts',(12.6571748903804,-1.24425507397135,7.19233592282916));
#56654=CARTESIAN_POINT('Ctrl Pts',(12.5158817257734,-0.43224932181273,7.14000254704507));
#56655=CARTESIAN_POINT('Ctrl Pts',(12.4912056194582,-0.29043679801142,7.13086279886071));
#56656=CARTESIAN_POINT('Ctrl Pts',(12.4798427838735,-0.146307696573625,
7.12172305067635));
#56657=CARTESIAN_POINT('Ctrl Pts',(12.4810882026093,-0.00198272270578489,
7.11258330249199));
#56658=CARTESIAN_POINT('Ctrl Pts',(12.4854953774899,-0.00143787083715985,
7.38741669750803));
#56659=CARTESIAN_POINT('Ctrl Pts',(12.4838166530455,-0.316448716062932,
7.4072765672669));
#56660=CARTESIAN_POINT('Ctrl Pts',(12.5388037075173,-0.630894974090679,
7.42713643702578));
#56661=CARTESIAN_POINT('Ctrl Pts',(12.6531758459131,-0.922010273445696,
7.44699630678465));
#56662=CARTESIAN_POINT('Ctrl Pts',(12.9545615131189,-1.68913747733048,7.49932968256874));
#56663=CARTESIAN_POINT('Ctrl Pts',(13.6683124514037,-2.29425637101525,7.55166305835282));
#56664=CARTESIAN_POINT('Ctrl Pts',(14.474415004267,-2.46605899527454,7.6039964341369));
#56665=CARTESIAN_POINT('Ctrl Pts',(15.2805175571303,-2.63786161953383,7.65632980992099));
#56666=CARTESIAN_POINT('Ctrl Pts',(16.1789717245721,-2.37634797436764,7.70866318570507));
#56667=CARTESIAN_POINT('Ctrl Pts',(16.766951270731,-1.79876895739606,7.76099656148916));
#56668=CARTESIAN_POINT('Ctrl Pts',(17.35493081689,-1.22118994042448,7.81332993727324));
#56669=CARTESIAN_POINT('Ctrl Pts',(17.6324357417662,-0.327545551647488,
7.86566331305733));
#56670=CARTESIAN_POINT('Ctrl Pts',(17.4750453812635,0.48149446094025,7.91799668884141));
#56671=CARTESIAN_POINT('Ctrl Pts',(17.3176550207607,1.290534473528,7.97033006462549));
#56672=CARTESIAN_POINT('Ctrl Pts',(16.7253693748791,2.01497010992651,8.02266344040958));
#56673=CARTESIAN_POINT('Ctrl Pts',(15.9637425539609,2.32999717716545,8.07499681619367));
#56674=CARTESIAN_POINT('Ctrl Pts',(15.2021157330427,2.64502424440439,8.12733019197775));
#56675=CARTESIAN_POINT('Ctrl Pts',(14.271147737088,2.55064274248376,8.17966356776183));
#56676=CARTESIAN_POINT('Ctrl Pts',(13.5882425327649,2.08916907124602,8.23199694354592));
#56677=CARTESIAN_POINT('Ctrl Pts',(12.9122114961964,1.63234062369425,8.28380352819995));
#56678=CARTESIAN_POINT('Ctrl Pts',(12.4792743543203,0.815773157793952,8.33561011285399));
#56679=CARTESIAN_POINT('Ctrl Pts',(12.4785663033905,-0.000147683907944251,
8.38741669750803));
#56680=CARTESIAN_POINT('Origin',(15.,0.,7.5));
#56681=CARTESIAN_POINT('',(12.4851788739807,0.00162480267774629,9.38741669750802));
#56682=CARTESIAN_POINT('',(12.486145438329,-0.000815058042068406,9.11258330249198));
#56683=CARTESIAN_POINT('',(12.4825,3.08304831685346E-16,7.5));
#56684=CARTESIAN_POINT('Ctrl Pts',(12.486145438329,-0.000815058042068406,
9.11258330249198));
#56685=CARTESIAN_POINT('Ctrl Pts',(12.4875376300823,0.467827170949961,9.08305689341869));
#56686=CARTESIAN_POINT('Ctrl Pts',(12.6134446697461,0.937164267550756,9.0535304843454));
#56687=CARTESIAN_POINT('Ctrl Pts',(12.8590980037376,1.33199914029708,9.02400407527211));
#56688=CARTESIAN_POINT('Ctrl Pts',(13.2945003653482,2.03181474323085,8.97167069948803));
#56689=CARTESIAN_POINT('Ctrl Pts',(14.1060849926179,2.49758205662421,8.91933732370394));
#56690=CARTESIAN_POINT('Ctrl Pts',(14.9299740278219,2.52047206702312,8.86700394791986));
#56691=CARTESIAN_POINT('Ctrl Pts',(15.753863063026,2.54336207742203,8.81467057213577));
#56692=CARTESIAN_POINT('Ctrl Pts',(16.5900565061644,2.12337478482649,8.76233719635169));
#56693=CARTESIAN_POINT('Ctrl Pts',(17.063643014475,1.44881350868189,8.7100038205676));
#56694=CARTESIAN_POINT('Ctrl Pts',(17.5372295227856,0.774252232537298,8.65767044478352));
#56695=CARTESIAN_POINT('Ctrl Pts',(17.6482090962684,-0.154883027156347,
8.60533706899943));
#56696=CARTESIAN_POINT('Ctrl Pts',(17.3468235115742,-0.922010021015011,
8.55300369321535));
#56697=CARTESIAN_POINT('Ctrl Pts',(17.0454379268799,-1.68913701487367,8.50067031743127));
#56698=CARTESIAN_POINT('Ctrl Pts',(16.3316871840086,-2.29425574289735,8.44833694164718));
#56699=CARTESIAN_POINT('Ctrl Pts',(15.5255848518399,-2.46605832012208,8.3960035658631));
#56700=CARTESIAN_POINT('Ctrl Pts',(14.7194825196712,-2.6378608973468,8.34367019007902));
#56701=CARTESIAN_POINT('Ctrl Pts',(13.8210285982051,-2.37634732377256,8.29133681429493));
#56702=CARTESIAN_POINT('Ctrl Pts',(13.2330492130222,-1.79876846492951,8.23900343851085));
#56703=CARTESIAN_POINT('Ctrl Pts',(12.7595946043877,-1.33368860080475,8.19686339317123));
#56704=CARTESIAN_POINT('Ctrl Pts',(12.4874468138073,-0.663676964701131,
8.1547233478316));
#56705=CARTESIAN_POINT('Ctrl Pts',(12.4815651121962,0.00207920831391661,
8.11258330249198));
#56706=CARTESIAN_POINT('Ctrl Pts',(12.4785663033905,-0.000147683907944251,
8.38741669750803));
#56707=CARTESIAN_POINT('Ctrl Pts',(12.478559103631,-0.0084443100048087,
8.38794348863808));
#56708=CARTESIAN_POINT('Ctrl Pts',(12.4785965949646,-0.016740869242818,
8.38847027976812));
#56709=CARTESIAN_POINT('Ctrl Pts',(12.4786789762444,-0.0250369827190495,
8.38899707089817));
#56710=CARTESIAN_POINT('Ctrl Pts',(12.4868630367383,-0.84920352489154,8.44133044668226));
#56711=CARTESIAN_POINT('Ctrl Pts',(12.9380735704173,-1.66897076868167,8.49366382246634));
#56712=CARTESIAN_POINT('Ctrl Pts',(13.6300081701693,-2.11679213546203,8.54599719825043));
#56713=CARTESIAN_POINT('Ctrl Pts',(14.3219427699214,-2.5646135022424,8.59833057403451));
#56714=CARTESIAN_POINT('Ctrl Pts',(15.2546014357464,-2.64048899201301,8.65066394981859));
#56715=CARTESIAN_POINT('Ctrl Pts',(16.0098221810285,-2.31039947008532,8.70299732560268));
#56716=CARTESIAN_POINT('Ctrl Pts',(16.7650429263106,-1.98030994815763,8.75533070138676));
#56717=CARTESIAN_POINT('Ctrl Pts',(17.3428257510498,-1.24425541453165,8.80766407717086));
#56718=CARTESIAN_POINT('Ctrl Pts',(17.4841189543331,-0.432249440103775,
8.85999745295494));
#56719=CARTESIAN_POINT('Ctrl Pts',(17.6254121576165,0.379756534324098,8.91233082873902));
#56720=CARTESIAN_POINT('Ctrl Pts',(17.3302157394439,1.26771394955386,8.9646642045231));
#56721=CARTESIAN_POINT('Ctrl Pts',(16.7308824297867,1.83350281974262,9.01699758030718));
#56722=CARTESIAN_POINT('Ctrl Pts',(16.1315491201295,2.39929168993138,9.06933095609127));
#56723=CARTESIAN_POINT('Ctrl Pts',(15.2280789189876,2.64291201507916,9.12166433187536));
#56724=CARTESIAN_POINT('Ctrl Pts',(14.4255470250055,2.45513549159302,9.17399770765945));
#56725=CARTESIAN_POINT('Ctrl Pts',(13.6230151310234,2.26735896810689,9.22633108344353));
#56726=CARTESIAN_POINT('Ctrl Pts',(12.9214215442012,1.64818559598687,9.2786644592276));
#56727=CARTESIAN_POINT('Ctrl Pts',(12.6353291141696,0.875224653029136,9.33099783501169));
#56728=CARTESIAN_POINT('Ctrl Pts',(12.5325202200407,0.597456870981902,9.34980412251047));
#56729=CARTESIAN_POINT('Ctrl Pts',(12.4833676454127,0.29982951718309,9.36861041000924));
#56730=CARTESIAN_POINT('Ctrl Pts',(12.4851788739807,0.00162480267774629,
9.38741669750802));
#56731=CARTESIAN_POINT('Origin',(15.,0.,7.5));
#56732=CARTESIAN_POINT('',(12.4833920687165,-0.00213593309729046,10.387416697508));
#56733=CARTESIAN_POINT('',(12.4790122776664,-0.000936909191352325,10.112583302492));
#56734=CARTESIAN_POINT('',(12.4825,3.08304831685346E-16,7.5));
#56735=CARTESIAN_POINT('Ctrl Pts',(12.4790122776664,-0.000936909191352325,
10.112583302492));
#56736=CARTESIAN_POINT('Ctrl Pts',(12.4827416706421,0.768933033990792,10.0637238147899));
#56737=CARTESIAN_POINT('Ctrl Pts',(12.8617552362247,1.54198463745441,10.0148643270877));
#56738=CARTESIAN_POINT('Ctrl Pts',(13.4744240244193,2.00756086084053,9.96600483938563));
#56739=CARTESIAN_POINT('Ctrl Pts',(14.1306532939369,2.50623934889895,9.91367146360154));
#56740=CARTESIAN_POINT('Ctrl Pts',(15.0549445147503,2.65216539497217,9.86133808781746));
#56741=CARTESIAN_POINT('Ctrl Pts',(15.8328874429565,2.37991212159725,9.80900471203338));
#56742=CARTESIAN_POINT('Ctrl Pts',(16.6108303711627,2.10765884822232,9.75667133624929));
#56743=CARTESIAN_POINT('Ctrl Pts',(17.2424250067619,1.41722625539925,9.70433796046521));
#56744=CARTESIAN_POINT('Ctrl Pts',(17.4444927838351,0.618173228507267,9.65200458468112));
#56745=CARTESIAN_POINT('Ctrl Pts',(17.6465605609084,-0.18087979838472,9.59967120889704));
#56746=CARTESIAN_POINT('Ctrl Pts',(17.4191014794558,-1.08855325934562,9.54733783311295));
#56747=CARTESIAN_POINT('Ctrl Pts',(16.8640979515296,-1.69788746613335,9.49500445732887));
#56748=CARTESIAN_POINT('Ctrl Pts',(16.3090944236034,-2.30722167292107,9.44267108154478));
#56749=CARTESIAN_POINT('Ctrl Pts',(15.4265464492036,-2.61821662553562,9.3903377057607));
#56750=CARTESIAN_POINT('Ctrl Pts',(14.6121486245737,-2.49143621341537,9.33800432997662));
#56751=CARTESIAN_POINT('Ctrl Pts',(13.7977507999438,-2.36465580129513,9.28567095419253));
#56752=CARTESIAN_POINT('Ctrl Pts',(13.0515031250838,-1.80010002444009,9.23333757840845));
#56753=CARTESIAN_POINT('Ctrl Pts',(12.7079893356296,-1.05089018977548,9.18100420262436));
#56754=CARTESIAN_POINT('Ctrl Pts',(12.5582854909339,-0.724383376435316,
9.15819723591357));
#56755=CARTESIAN_POINT('Ctrl Pts',(12.4850700731909,-0.362806510824638,
9.13539026920278));
#56756=CARTESIAN_POINT('Ctrl Pts',(12.486145438329,-0.000815058042068406,
9.11258330249198));
#56757=CARTESIAN_POINT('Ctrl Pts',(12.4851788739807,0.00162480267774629,
9.38741669750802));
#56758=CARTESIAN_POINT('Ctrl Pts',(12.4884078589736,-0.530002494361348,
9.42094378579333));
#56759=CARTESIAN_POINT('Ctrl Pts',(12.6536116109961,-1.06346477741145,9.45447087407864));
#56760=CARTESIAN_POINT('Ctrl Pts',(12.9655342718635,-1.48950860327335,9.48799796236395));
#56761=CARTESIAN_POINT('Ctrl Pts',(13.4524231328298,-2.15453240282264,9.54033133814804));
#56762=CARTESIAN_POINT('Ctrl Pts',(14.2967921280032,-2.55783148812579,9.59266471393212));
#56763=CARTESIAN_POINT('Ctrl Pts',(15.1200643665754,-2.51858505945467,9.6449980897162));
#56764=CARTESIAN_POINT('Ctrl Pts',(15.9433366051476,-2.47933863078355,9.69733146550028));
#56765=CARTESIAN_POINT('Ctrl Pts',(16.7455120871185,-1.99754668813814,9.74966484128436));
#56766=CARTESIAN_POINT('Ctrl Pts',(17.1669315903404,-1.28922241490791,9.80199821706845));
#56767=CARTESIAN_POINT('Ctrl Pts',(17.5883510935622,-0.580898141677671,
9.85433159285254));
#56768=CARTESIAN_POINT('Ctrl Pts',(17.6290146180349,0.353958462137397,9.90666496863663));
#56769=CARTESIAN_POINT('Ctrl Pts',(17.2706904715522,1.09619889141998,9.95899834442071));
#56770=CARTESIAN_POINT('Ctrl Pts',(16.9123663250695,1.83843932070257,10.0113317202048));
#56771=CARTESIAN_POINT('Ctrl Pts',(16.1550545076315,2.38806357545267,10.0636650959889));
#56772=CARTESIAN_POINT('Ctrl Pts',(15.3382994168527,2.49864705542611,10.115998471773));
#56773=CARTESIAN_POINT('Ctrl Pts',(14.5215443260739,2.60923053539955,10.168331847557));
#56774=CARTESIAN_POINT('Ctrl Pts',(13.6453459619542,2.28077324059635,10.2206652233411));
#56775=CARTESIAN_POINT('Ctrl Pts',(13.1025520413601,1.66053653868267,10.2729985991252));
#56776=CARTESIAN_POINT('Ctrl Pts',(12.7069762589991,1.20852223030592,10.3111379652528));
#56777=CARTESIAN_POINT('Ctrl Pts',(12.4884769342622,0.601539190041919,10.3492773313804));
#56778=CARTESIAN_POINT('Ctrl Pts',(12.4833920687165,-0.00213593309729046,
10.387416697508));
#56779=CARTESIAN_POINT('Origin',(15.,0.,7.5));
#56780=CARTESIAN_POINT('',(12.4794948718273,0.00124609658704006,11.387416697508));
#56781=CARTESIAN_POINT('',(12.4841021658346,0.00201143405015815,11.112583302492));
#56782=CARTESIAN_POINT('',(12.4825,3.08304831685346E-16,7.5));
#56783=CARTESIAN_POINT('',(16.9134659966651,1.63598720337492,12.));
#56784=CARTESIAN_POINT('Ctrl Pts',(12.4794948718273,0.00124609658704006,
11.387416697508));
#56785=CARTESIAN_POINT('Ctrl Pts',(12.4843009282632,-0.742606326482963,
11.4346110043198));
#56786=CARTESIAN_POINT('Ctrl Pts',(12.8347911135691,-1.49019380442116,11.4818053111315));
#56787=CARTESIAN_POINT('Ctrl Pts',(13.4121725655462,-1.95845906653105,11.5289996179432));
#56788=CARTESIAN_POINT('Ctrl Pts',(14.0524260736147,-2.47771453576351,11.5813329937273));
#56789=CARTESIAN_POINT('Ctrl Pts',(14.971674348053,-2.65350400257885,11.6336663695114));
#56790=CARTESIAN_POINT('Ctrl Pts',(15.7577964008607,-2.4053165320775,11.6859997452955));
#56791=CARTESIAN_POINT('Ctrl Pts',(16.5439184536685,-2.15712906157615,11.7383331210796));
#56792=CARTESIAN_POINT('Ctrl Pts',(17.1969142848456,-1.4849646537581,11.7906664968637));
#56793=CARTESIAN_POINT('Ctrl Pts',(17.4237876204482,-0.693982202234524,
11.8429998726477));
#56794=CARTESIAN_POINT('Ctrl Pts',(17.6506609560507,0.0970002492890512,
11.8953332484318));
#56795=CARTESIAN_POINT('Ctrl Pts',(17.4514117960785,1.00680074451815,11.9476666242159));
#56796=CARTESIAN_POINT('Ctrl Pts',(16.9134659966651,1.63598720337493,12.));
#56797=CARTESIAN_POINT('',(13.0830107080184,1.63831915944298,12.));
#56798=CARTESIAN_POINT('Origin',(15.,0.,12.));
#56799=CARTESIAN_POINT('Ctrl Pts',(13.0829974340784,1.63832794503776,12.));
#56800=CARTESIAN_POINT('Ctrl Pts',(13.5967216860793,2.23547110522819,11.9500021225376));
#56801=CARTESIAN_POINT('Ctrl Pts',(14.4140905740858,2.57572139725963,11.9000042450751));
#56802=CARTESIAN_POINT('Ctrl Pts',(15.1991791514308,2.51337952595466,11.8500063676127));
#56803=CARTESIAN_POINT('Ctrl Pts',(16.0209407466675,2.44812554431239,11.7976729918286));
#56804=CARTESIAN_POINT('Ctrl Pts',(16.8073358429282,1.94178921121356,11.7453396160445));
#56805=CARTESIAN_POINT('Ctrl Pts',(17.2062539503585,1.22068465472099,11.6930062402604));
#56806=CARTESIAN_POINT('Ctrl Pts',(17.6051720577887,0.499580098228415,11.6406728644763));
#56807=CARTESIAN_POINT('Ctrl Pts',(17.6166131763885,-0.436292681657898,
11.5883394886922));
#56808=CARTESIAN_POINT('Ctrl Pts',(17.2352051529428,-1.16697139580525,11.5360061129082));
#56809=CARTESIAN_POINT('Ctrl Pts',(16.853797129497,-1.8976501099526,11.4836727371241));
#56810=CARTESIAN_POINT('Ctrl Pts',(16.0795399640059,-2.42313475836099,11.43133936134));
#56811=CARTESIAN_POINT('Ctrl Pts',(15.259700012361,-2.508006015706,11.3790059855559));
#56812=CARTESIAN_POINT('Ctrl Pts',(14.439860060716,-2.59287727305101,11.3266726097718));
#56813=CARTESIAN_POINT('Ctrl Pts',(13.5744373229174,-2.23713513933264,11.2743392339877));
#56814=CARTESIAN_POINT('Ctrl Pts',(13.0513843414681,-1.60018372469102,11.2220058582037));
#56815=CARTESIAN_POINT('Ctrl Pts',(12.6868381785572,-1.15625509336019,11.1855316729664));
#56816=CARTESIAN_POINT('Ctrl Pts',(12.488598465426,-0.575728774038117,11.1490574877292));
#56817=CARTESIAN_POINT('Ctrl Pts',(12.4841021658346,0.00201143405015815,
11.112583302492));
#56818=CARTESIAN_POINT('Origin',(15.,0.,14.2084234471775));
#56819=CARTESIAN_POINT('',(11.9225958479619,0.00147606609843115,4.79157655282255));
#56820=CARTESIAN_POINT('',(11.9313248632922,-0.000102231845577353,4.70842344717745));
#56821=CARTESIAN_POINT('',(11.9265,6.70613782525944E-14,14.2084234471775));
#56822=CARTESIAN_POINT('',(15.7937992825329,-2.9692229537457,4.));
#56823=CARTESIAN_POINT('Ctrl Pts',(11.9313248632922,-0.000102231845577234,
4.70842344717745));
#56824=CARTESIAN_POINT('Ctrl Pts',(11.9316626296779,0.519548226111607,4.68161580125464));
#56825=CARTESIAN_POINT('Ctrl Pts',(12.3017104806267,2.0539878015009,4.60247477954774));
#56826=CARTESIAN_POINT('Ctrl Pts',(14.713653685934,3.60697232347283,4.47100038205677));
#56827=CARTESIAN_POINT('Ctrl Pts',(17.8529409071999,2.23046453345384,4.3140002547045));
#56828=CARTESIAN_POINT('Ctrl Pts',(18.4294036968932,-1.15306868324745,4.15700012735226));
#56829=CARTESIAN_POINT('Ctrl Pts',(16.7701400584231,-2.7082056372685,4.05233337578409));
#56830=CARTESIAN_POINT('Ctrl Pts',(15.7937992825329,-2.9692229537457,4.));
#56831=CARTESIAN_POINT('',(14.2042685477155,-2.9740056618826,4.));
#56832=CARTESIAN_POINT('Origin',(15.,0.,4.));
#56833=CARTESIAN_POINT('Ctrl Pts',(11.9225958479619,0.00147606609843164,
4.79157655282255));
#56834=CARTESIAN_POINT('Ctrl Pts',(11.9220803947843,0.0885957531718082,
4.78704908248048));
#56835=CARTESIAN_POINT('Ctrl Pts',(11.9646120017673,1.18222348786824,4.73018823635433));
#56836=CARTESIAN_POINT('Ctrl Pts',(13.2680522040149,3.17774609218688,4.62099401444409));
#56837=CARTESIAN_POINT('Ctrl Pts',(16.6951963308219,3.19795784272698,4.46399388709183));
#56838=CARTESIAN_POINT('Ctrl Pts',(18.6022504225887,0.349454018091392,4.30699375973959));
#56839=CARTESIAN_POINT('Ctrl Pts',(17.2987966073653,-2.76330605967289,4.15232913070897));
#56840=CARTESIAN_POINT('Ctrl Pts',(15.1340732479013,-3.21955219912907,4.04999787746244));
#56841=CARTESIAN_POINT('Ctrl Pts',(14.2042612683071,-2.97402368063355,4.));
#56842=CARTESIAN_POINT('Origin',(15.,0.,14.2084234471775));
#56843=CARTESIAN_POINT('',(11.9311214597158,0.000692114352876805,5.79157655282255));
#56844=CARTESIAN_POINT('',(11.9232839890155,-0.001880590663607,5.70842344717745));
#56845=CARTESIAN_POINT('',(11.9265,6.70613782525944E-14,14.2084234471775));
#56846=CARTESIAN_POINT('Ctrl Pts',(11.9232839890155,-0.00188059066360697,
5.70842344717745));
#56847=CARTESIAN_POINT('Ctrl Pts',(11.9297313241637,0.88651553618964,5.66228272262581));
#56848=CARTESIAN_POINT('Ctrl Pts',(12.7977715060129,2.79354605065376,5.56380862229009));
#56849=CARTESIAN_POINT('Ctrl Pts',(16.0189351514379,3.47279968000896,5.41300114617029));
#56850=CARTESIAN_POINT('Ctrl Pts',(18.4587231497003,1.06591431050395,5.25600101881802));
#56851=CARTESIAN_POINT('Ctrl Pts',(17.7969596462713,-2.29690631906584,5.09900089146578));
#56852=CARTESIAN_POINT('Ctrl Pts',(14.6272939950368,-3.59983577334609,4.94200076411352));
#56853=CARTESIAN_POINT('Ctrl Pts',(12.2757333222409,-2.00384044231271,4.81180828268409));
#56854=CARTESIAN_POINT('Ctrl Pts',(11.9310032485729,-0.494903500494573,
4.73394917703873));
#56855=CARTESIAN_POINT('Ctrl Pts',(11.9313248632922,-0.000102231845577234,
4.70842344717745));
#56856=CARTESIAN_POINT('Ctrl Pts',(11.9311214597158,0.000692114352877186,
5.79157655282255));
#56857=CARTESIAN_POINT('Ctrl Pts',(11.930169752624,0.463111161065124,5.76771600385165));
#56858=CARTESIAN_POINT('Ctrl Pts',(12.2437393113606,1.9385290048203,5.69152207909668));
#56859=CARTESIAN_POINT('Ctrl Pts',(14.5144143770745,3.58648699137295,5.56299477855761));
#56860=CARTESIAN_POINT('Ctrl Pts',(17.7235443678513,2.3834921742297,5.40599465120536));
#56861=CARTESIAN_POINT('Ctrl Pts',(18.4904461542425,-0.956822661448993,
5.2489945238531));
#56862=CARTESIAN_POINT('Ctrl Pts',(16.1274310791049,-3.43910703392132,5.09199439650085));
#56863=CARTESIAN_POINT('Ctrl Pts',(12.8507354093227,-2.85493220992714,4.93952173949066));
#56864=CARTESIAN_POINT('Ctrl Pts',(11.9280385574681,-0.918427369528735,
4.83938245826456));
#56865=CARTESIAN_POINT('Ctrl Pts',(11.9225958479619,0.00147606609843164,
4.79157655282255));
#56866=CARTESIAN_POINT('Origin',(15.,0.,14.2084234471775));
#56867=CARTESIAN_POINT('',(11.9247764014775,-0.00242061498952145,6.79157655282255));
#56868=CARTESIAN_POINT('',(11.9270135324726,0.00264512890178066,6.70842344717746));
#56869=CARTESIAN_POINT('',(11.9265,6.70613782525944E-14,14.2084234471775));
#56870=CARTESIAN_POINT('Ctrl Pts',(11.9270135324726,0.00264512890178106,
6.70842344717746));
#56871=CARTESIAN_POINT('Ctrl Pts',(11.9248054756842,0.256447062439599,6.69528301978107));
#56872=CARTESIAN_POINT('Ctrl Pts',(12.0687133238052,1.518578012587,6.62980921660061));
#56873=CARTESIAN_POINT('Ctrl Pts',(13.8044957855091,3.41606212207931,6.51200203763605));
#56874=CARTESIAN_POINT('Ctrl Pts',(17.1897706782275,2.88159878204111,6.35500191028381));
#56875=CARTESIAN_POINT('Ctrl Pts',(18.6114579568395,-0.236820710438023,
6.19800178293155));
#56876=CARTESIAN_POINT('Ctrl Pts',(16.7947147560542,-3.14288298322814,6.04100165557929));
#56877=CARTESIAN_POINT('Ctrl Pts',(13.3686365056666,-3.23068767821543,5.88400152822705));
#56878=CARTESIAN_POINT('Ctrl Pts',(11.9823834565481,-1.24709989542488,5.77314212542643));
#56879=CARTESIAN_POINT('Ctrl Pts',(11.9224186775506,-0.121114248637474,
5.7146160984099));
#56880=CARTESIAN_POINT('Ctrl Pts',(11.9232839890155,-0.00188059066360697,
5.70842344717745));
#56881=CARTESIAN_POINT('Ctrl Pts',(11.9247764014775,-0.00242061498952133,
6.79157655282255));
#56882=CARTESIAN_POINT('Ctrl Pts',(11.9319620270346,0.830283431407061,6.74838292522283));
#56883=CARTESIAN_POINT('Ctrl Pts',(12.7081731527432,2.68370300380156,6.65285592183902));
#56884=CARTESIAN_POINT('Ctrl Pts',(15.824553937525,3.52403365117268,6.50499554267113));
#56885=CARTESIAN_POINT('Ctrl Pts',(18.3941832901488,1.25627336953411,6.34799541531888));
#56886=CARTESIAN_POINT('Ctrl Pts',(17.9202159270872,-2.13799965619268,6.19099528796662));
#56887=CARTESIAN_POINT('Ctrl Pts',(14.8276629212552,-3.61510717519363,6.03399516061437));
#56888=CARTESIAN_POINT('Ctrl Pts',(12.3361598311427,-2.11869381838128,5.90085558223301));
#56889=CARTESIAN_POINT('Ctrl Pts',(11.9322571331336,-0.551113187705301,
5.82004937963574));
#56890=CARTESIAN_POINT('Ctrl Pts',(11.9311214597158,0.000692114352877186,
5.79157655282255));
#56891=CARTESIAN_POINT('Origin',(15.,0.,14.2084234471775));
#56892=CARTESIAN_POINT('',(11.9253586384648,0.00253840983232584,7.79157655282255));
#56893=CARTESIAN_POINT('',(11.9301569186554,-0.00175543039446494,7.70842344717746));
#56894=CARTESIAN_POINT('',(11.9265,6.70613782525944E-14,14.2084234471775));
#56895=CARTESIAN_POINT('Ctrl Pts',(11.9301569186554,-0.00175543039446478,
7.70842344717746));
#56896=CARTESIAN_POINT('Ctrl Pts',(11.9335080846202,0.627087276122613,7.67594994115225));
#56897=CARTESIAN_POINT('Ctrl Pts',(12.425309891706,2.27416779560488,7.59114305934296));
#56898=CARTESIAN_POINT('Ctrl Pts',(15.1005134031695,3.61781798694653,7.45400280174957));
#56899=CARTESIAN_POINT('Ctrl Pts',(18.0729932858696,1.91191582667314,7.29700267439733));
#56900=CARTESIAN_POINT('Ctrl Pts',(18.2898906220475,-1.50841957701434,7.14000254704506));
#56901=CARTESIAN_POINT('Ctrl Pts',(15.5567114486024,-3.57614071471203,6.98300241969282));
#56902=CARTESIAN_POINT('Ctrl Pts',(12.5948647250275,-2.532436114927,6.83914271973694));
#56903=CARTESIAN_POINT('Ctrl Pts',(11.9335993346794,-0.754350498545223,
6.74761639556516));
#56904=CARTESIAN_POINT('Ctrl Pts',(11.9270135324726,0.00264512890178106,
6.70842344717746));
#56905=CARTESIAN_POINT('Ctrl Pts',(11.9253586384648,0.00253840983232619,
7.79157655282255));
#56906=CARTESIAN_POINT('Ctrl Pts',(11.9236216864083,0.199145893570575,7.78138322237808));
#56907=CARTESIAN_POINT('Ctrl Pts',(12.0296403223963,1.40328729141077,7.71885651614953));
#56908=CARTESIAN_POINT('Ctrl Pts',(13.6166705510885,3.34441360725337,7.60399643413689));
#56909=CARTESIAN_POINT('Ctrl Pts',(17.0263976837988,2.99873559323853,7.44699630678466));
#56910=CARTESIAN_POINT('Ctrl Pts',(18.6190345729722,-0.0359373922966709,
7.2899961794324));
#56911=CARTESIAN_POINT('Ctrl Pts',(16.9664484412042,-3.03838498006983,7.13299605208014));
#56912=CARTESIAN_POINT('Ctrl Pts',(13.5505291268344,-3.3162835943375,6.97599592472789));
#56913=CARTESIAN_POINT('Ctrl Pts',(12.0165601959407,-1.36211545786235,6.86218942497536));
#56914=CARTESIAN_POINT('Ctrl Pts',(11.923255927005,-0.178620339789062,6.80071630100691));
#56915=CARTESIAN_POINT('Ctrl Pts',(11.9247764014775,-0.00242061498952133,
6.79157655282255));
#56916=CARTESIAN_POINT('Origin',(15.,0.,14.2084234471775));
#56917=CARTESIAN_POINT('',(11.9309505480454,-0.000995066888654084,8.79157655282255));
#56918=CARTESIAN_POINT('',(11.9216975306736,-0.000180300492997754,8.70842344717746));
#56919=CARTESIAN_POINT('',(11.9265,6.70613782525944E-14,14.2084234471775));
#56920=CARTESIAN_POINT('Ctrl Pts',(11.9216975306736,-0.000180300492997622,
8.70842344717746));
#56921=CARTESIAN_POINT('Ctrl Pts',(11.9225619574989,0.995939940607609,8.65661686252342));
#56922=CARTESIAN_POINT('Ctrl Pts',(12.9850426088341,2.99989628694768,8.5524769020853));
#56923=CARTESIAN_POINT('Ctrl Pts',(16.383329827636,3.34441452287188,8.39600356586309));
#56924=CARTESIAN_POINT('Ctrl Pts',(18.5526127662067,0.691124042072478,8.23900343851084));
#56925=CARTESIAN_POINT('Ctrl Pts',(17.5362337553543,-2.58190399634584,8.08200331115859));
#56926=CARTESIAN_POINT('Ctrl Pts',(14.2455896040548,-3.53971395275292,7.92500318380633));
#56927=CARTESIAN_POINT('Ctrl Pts',(12.1721380845128,-1.78183929043833,7.8004765624793));
#56928=CARTESIAN_POINT('Ctrl Pts',(11.928107441166,-0.386337687713779,7.72828331693634));
#56929=CARTESIAN_POINT('Ctrl Pts',(11.9301569186554,-0.00175543039446478,
7.70842344717746));
#56930=CARTESIAN_POINT('Ctrl Pts',(11.9309505480454,-0.000995066888653875,
8.79157655282255));
#56931=CARTESIAN_POINT('Ctrl Pts',(11.9326502109465,0.571148683183627,8.76205014374926));
#56932=CARTESIAN_POINT('Ctrl Pts',(12.3588112254404,2.15972684180816,8.68019035889189));
#56933=CARTESIAN_POINT('Ctrl Pts',(14.8994866243195,3.61781699652394,8.54599719825042));
#56934=CARTESIAN_POINT('Ctrl Pts',(17.9620970086125,2.07958747065415,8.38899707089818));
#56935=CARTESIAN_POINT('Ctrl Pts',(18.3685665845007,-1.32342808525659,8.23199694354591));
#56936=CARTESIAN_POINT('Ctrl Pts',(15.7544101894084,-3.53971298366467,8.07499681619367));
#56937=CARTESIAN_POINT('Ctrl Pts',(12.6774139888043,-2.64408967670503,7.92819001928588));
#56938=CARTESIAN_POINT('Ctrl Pts',(11.932539337532,-0.810252691562618,7.83371659816217));
#56939=CARTESIAN_POINT('Ctrl Pts',(11.9253586384648,0.00253840983232619,
7.79157655282255));
#56940=CARTESIAN_POINT('Origin',(15.,0.,14.2084234471775));
#56941=CARTESIAN_POINT('',(11.9222420001619,-0.00114382935434674,9.79157655282255));
#56942=CARTESIAN_POINT('',(11.9297705140734,0.00198364688382296,9.70842344717746));
#56943=CARTESIAN_POINT('',(11.9265,6.70613782525944E-14,14.2084234471775));
#56944=CARTESIAN_POINT('Ctrl Pts',(11.9297705140734,0.00198364688382347,
9.70842344717746));
#56945=CARTESIAN_POINT('Ctrl Pts',(11.9275592683916,0.36604807192143,9.68961715967868));
#56946=CARTESIAN_POINT('Ctrl Pts',(12.1545555502906,1.7405498801195,9.61847749639582));
#56947=CARTESIAN_POINT('Ctrl Pts',(14.1754458368614,3.52403461675767,9.49500445732887));
#56948=CARTESIAN_POINT('Ctrl Pts',(17.4844615229107,2.63176005547664,9.33800432997661));
#56949=CARTESIAN_POINT('Ctrl Pts',(18.565636725993,-0.620439089359897,9.18100420262437));
#56950=CARTESIAN_POINT('Ctrl Pts',(16.4494712699821,-3.31628450238807,9.0240040752721));
#56951=CARTESIAN_POINT('Ctrl Pts',(13.033551020433,-3.03838581184986,8.86700394791986));
#56952=CARTESIAN_POINT('Ctrl Pts',(11.9262816166307,-1.02667925906391,8.76181040522164));
#56953=CARTESIAN_POINT('Ctrl Pts',(11.9216887408183,-0.0103092698311159,
8.70895023830751));
#56954=CARTESIAN_POINT('Ctrl Pts',(11.9216975306736,-0.000180300492997622,
8.70842344717746));
#56955=CARTESIAN_POINT('Ctrl Pts',(11.9222420001619,-0.00114382935434687,
9.79157655282255));
#56956=CARTESIAN_POINT('Ctrl Pts',(11.9267950445754,0.938754987078744,9.74271706512043));
#56957=CARTESIAN_POINT('Ctrl Pts',(12.8851347215443,2.89342387288723,9.64152420163423));
#56958=CARTESIAN_POINT('Ctrl Pts',(16.1955038860992,3.41606118929613,9.48799796236394));
#56959=CARTESIAN_POINT('Ctrl Pts',(18.5087584392439,0.887308966009096,9.3309978350117));
#56960=CARTESIAN_POINT('Ctrl Pts',(17.6756754360527,-2.43710142000481,9.17399770765943));
#56961=CARTESIAN_POINT('Ctrl Pts',(14.4432887039958,-3.57613973602564,9.0169975803072));
#56962=CARTESIAN_POINT('Ctrl Pts',(12.2241286148511,-1.89728740549368,8.88952386202822));
#56963=CARTESIAN_POINT('Ctrl Pts',(11.9296376841916,-0.442933787892533,
8.81438351953334));
#56964=CARTESIAN_POINT('Ctrl Pts',(11.9309505480454,-0.000995066888653875,
8.79157655282255));
#56965=CARTESIAN_POINT('Origin',(15.,0.,14.2084234471775));
#56966=CARTESIAN_POINT('',(11.9284560106028,0.00245566734982605,10.7915765528225));
#56967=CARTESIAN_POINT('',(11.9275890856804,-0.00260766251225693,10.7084234471775));
#56968=CARTESIAN_POINT('',(11.9265,6.70613782525944E-14,14.2084234471775));
#56969=CARTESIAN_POINT('Ctrl Pts',(11.9275890856804,-0.00260766251225678,
10.7084234471775));
#56970=CARTESIAN_POINT('Ctrl Pts',(11.9337969642323,0.734391539461283,10.6702840810499));
#56971=CARTESIAN_POINT('Ctrl Pts',(12.5665847955819,2.49225272359552,10.5798113391382));
#56972=CARTESIAN_POINT('Ctrl Pts',(15.4855857629831,3.58648800243424,10.4370052214424));
#56973=CARTESIAN_POINT('Ctrl Pts',(18.2592872973176,1.57345505668517,10.2800050940901));
#56974=CARTESIAN_POINT('Ctrl Pts',(18.1103546151327,-1.85051527716861,10.1230049667379));
#56975=CARTESIAN_POINT('Ctrl Pts',(15.1723371249586,-3.61510816978504,9.96600483938563));
#56976=CARTESIAN_POINT('Ctrl Pts',(12.4502253736084,-2.31493586870828,9.82781099953215));
#56977=CARTESIAN_POINT('Ctrl Pts',(11.9337126333884,-0.647055676830039,
9.74195053546276));
#56978=CARTESIAN_POINT('Ctrl Pts',(11.9297705140734,0.00198364688382347,
9.70842344717746));
#56979=CARTESIAN_POINT('Ctrl Pts',(11.9284560106028,0.0024556673498264,
10.7915765528226));
#56980=CARTESIAN_POINT('Ctrl Pts',(11.9260692195737,0.309140112596412,10.7757173622757));
#56981=CARTESIAN_POINT('Ctrl Pts',(12.1080878285752,1.62508037117336,10.7075247959448));
#56982=CARTESIAN_POINT('Ctrl Pts',(13.9810651784412,3.47279856287599,10.5869988538297));
#56983=CARTESIAN_POINT('Ctrl Pts',(17.3344994031312,2.76565299665532,10.4299987264775));
#56984=CARTESIAN_POINT('Ctrl Pts',(18.5945871152999,-0.421511967551375,
10.2729985991252));
#56985=CARTESIAN_POINT('Ctrl Pts',(16.6313630370479,-3.23068676566348,10.115998471773));
#56986=CARTESIAN_POINT('Ctrl Pts',(13.205285741413,-3.14288213812672,9.9589983444207));
#56987=CARTESIAN_POINT('Ctrl Pts',(11.9539254885605,-1.14120637601563,9.85085770477057));
#56988=CARTESIAN_POINT('Ctrl Pts',(11.921918280707,-0.0679702217342443,
9.79505044090452));
#56989=CARTESIAN_POINT('Ctrl Pts',(11.9222420001619,-0.00114382935434687,
9.79157655282255));
#56990=CARTESIAN_POINT('Origin',(15.,0.,14.2084234471775));
#56991=CARTESIAN_POINT('',(11.9297760945785,-0.00333806817183438,11.7915765528226));
#56992=CARTESIAN_POINT('',(11.9228311771842,0.00152130202986591,11.7084234471775));
#56993=CARTESIAN_POINT('',(11.9265,6.70613782525944E-14,14.2084234471775));
#56994=CARTESIAN_POINT('',(14.2062007174671,-2.96922295374568,12.));
#56995=CARTESIAN_POINT('Ctrl Pts',(14.2062007174671,-2.96922295374568,12.));
#56996=CARTESIAN_POINT('Ctrl Pts',(13.2298599415769,-2.70820563726846,11.9476666242159));
#56997=CARTESIAN_POINT('Ctrl Pts',(12.1284916041782,-1.6759644246982,11.8781921418234));
#56998=CARTESIAN_POINT('Ctrl Pts',(11.9274999800733,-0.33505537898738,11.8087176594309));
#56999=CARTESIAN_POINT('Ctrl Pts',(11.9297760945785,-0.00333806817183434,
11.7915765528225));
#57000=CARTESIAN_POINT('',(15.7957331921886,-2.97400465723624,12.));
#57001=CARTESIAN_POINT('Origin',(15.,0.,12.));
#57002=CARTESIAN_POINT('Ctrl Pts',(15.7957405241459,-2.97402278592475,12.));
#57003=CARTESIAN_POINT('Ctrl Pts',(14.8659292530302,-3.21955068215558,11.9500021225376));
#57004=CARTESIAN_POINT('Ctrl Pts',(12.809912552641,-2.78622279751186,11.8528099382634));
#57005=CARTESIAN_POINT('Ctrl Pts',(11.9286986705132,-0.906613920335824,
11.7556177539892));
#57006=CARTESIAN_POINT('Ctrl Pts',(11.9228311771842,0.00152130202986659,
11.7084234471775));
#57007=CARTESIAN_POINT('Origin',(-7.5,12.9903810567666,7.5));
#57008=CARTESIAN_POINT('',(-10.0135512354019,12.9902955808623,4.38741669750803));
#57009=CARTESIAN_POINT('',(-10.0159871075715,12.98719611739,4.11258330249198));
#57010=CARTESIAN_POINT('',(-10.0175,12.9903810567666,7.5));
#57011=CARTESIAN_POINT('',(-9.41346599666504,14.6263682601415,4.));
#57012=CARTESIAN_POINT('Ctrl Pts',(-10.0159871075715,12.98719611739,4.11258330249198));
#57013=CARTESIAN_POINT('Ctrl Pts',(-10.0108029441705,13.5796929638899,4.07505553499465));
#57014=CARTESIAN_POINT('Ctrl Pts',(-9.79922182808404,14.175184617071,4.03752776749733));
#57015=CARTESIAN_POINT('Ctrl Pts',(-9.41346599666504,14.6263682601416,4.));
#57016=CARTESIAN_POINT('',(-10.0175,12.9903810567666,4.));
#57017=CARTESIAN_POINT('Origin',(-7.5,12.9903810567666,4.));
#57018=CARTESIAN_POINT('',(-10.0175,12.9903810567666,3.));
#57019=CARTESIAN_POINT('',(-10.0175,12.9903810567666,7.5));
#57020=CARTESIAN_POINT('Origin',(-7.5,12.9903810567666,3.));
#57021=CARTESIAN_POINT('',(-5.58300657818904,14.6286918237334,4.));
#57022=CARTESIAN_POINT('Origin',(-7.5,12.9903810567666,4.));
#57023=CARTESIAN_POINT('Ctrl Pts',(-5.58299280741585,14.6287008947316,4.));
#57024=CARTESIAN_POINT('Ctrl Pts',(-6.09671594976083,15.225839628633,4.04999787746244));
#57025=CARTESIAN_POINT('Ctrl Pts',(-6.91408837638834,15.566108849254,4.09999575492489));
#57026=CARTESIAN_POINT('Ctrl Pts',(-7.69917928811933,15.5037708430362,4.14999363238733));
#57027=CARTESIAN_POINT('Ctrl Pts',(-8.52094332678579,15.4385209070269,4.20232700817142));
#57028=CARTESIAN_POINT('Ctrl Pts',(-9.30733954710939,14.9321721158988,4.2546603839555));
#57029=CARTESIAN_POINT('Ctrl Pts',(-9.7062579619942,14.2110639837978,4.30699375973958));
#57030=CARTESIAN_POINT('Ctrl Pts',(-9.91060296091885,13.8416780768541,4.3338014056624));
#57031=CARTESIAN_POINT('Ctrl Pts',(-10.0132747138948,13.4159398344011,4.36060905158521));
#57032=CARTESIAN_POINT('Ctrl Pts',(-10.0135512354019,12.9902955808623,4.38741669750803));
#57033=CARTESIAN_POINT('Origin',(-7.5,12.9903810567666,7.5));
#57034=CARTESIAN_POINT('',(-10.0201376030965,12.9888406983805,5.38741669750803));
#57035=CARTESIAN_POINT('',(-10.0207017684327,12.9915893349038,5.11258330249198));
#57036=CARTESIAN_POINT('',(-10.0175,12.9903810567666,7.5));
#57037=CARTESIAN_POINT('Ctrl Pts',(-10.0207017684327,12.9915893349038,5.11258330249198));
#57038=CARTESIAN_POINT('Ctrl Pts',(-10.021123985829,13.062949094674,5.10805583214991));
#57039=CARTESIAN_POINT('Ctrl Pts',(-10.0183500982852,13.1342752724561,5.10352836180784));
#57040=CARTESIAN_POINT('Ctrl Pts',(-10.0122723502588,13.2053184595532,5.09900089146578));
#57041=CARTESIAN_POINT('Ctrl Pts',(-9.94201919621031,14.0265120900682,5.04666751568169));
#57042=CARTESIAN_POINT('Ctrl Pts',(-9.43032981516091,14.8098946989374,4.99433413989761));
#57043=CARTESIAN_POINT('Ctrl Pts',(-8.7066218792309,15.204343412931,4.94200076411352));
#57044=CARTESIAN_POINT('Ctrl Pts',(-7.98291394330089,15.5987921269246,4.88966738832944));
#57045=CARTESIAN_POINT('Ctrl Pts',(-7.04718745249026,15.6043069460425,4.83733401254535));
#57046=CARTESIAN_POINT('Ctrl Pts',(-6.31898125676283,15.2181990815764,4.78500063676127));
#57047=CARTESIAN_POINT('Ctrl Pts',(-5.59077506103539,14.8320912171102,4.73266726097718));
#57048=CARTESIAN_POINT('Ctrl Pts',(-5.07008916039116,14.0543606690598,4.6803338851931));
#57049=CARTESIAN_POINT('Ctrl Pts',(-4.99037298951262,13.2341300396427,4.62800050940902));
#57050=CARTESIAN_POINT('Ctrl Pts',(-4.91065681863409,12.4138994102257,4.57566713362493));
#57051=CARTESIAN_POINT('Ctrl Pts',(-5.27191037752124,11.5511686994419,4.52333375784085));
#57052=CARTESIAN_POINT('Ctrl Pts',(-5.91216754016691,11.0319148801645,4.47100038205676));
#57053=CARTESIAN_POINT('Ctrl Pts',(-6.55242470281257,10.5126610608871,4.41866700627268));
#57054=CARTESIAN_POINT('Ctrl Pts',(-7.47168546921673,10.336884133116,4.36633363048859));
#57055=CARTESIAN_POINT('Ctrl Pts',(-8.25780300491658,10.5850674765643,4.31400025470451));
#57056=CARTESIAN_POINT('Ctrl Pts',(-9.04392054061644,10.8332508200125,4.26166687892042));
#57057=CARTESIAN_POINT('Ctrl Pts',(-9.696894845612,11.50539443468,4.20933350313634));
#57058=CARTESIAN_POINT('Ctrl Pts',(-9.92376765947752,12.2963771799981,4.15700012735225));
#57059=CARTESIAN_POINT('Ctrl Pts',(-9.98795212995513,12.5201536995385,4.1421945190655));
#57060=CARTESIAN_POINT('Ctrl Pts',(-10.0180323849149,12.7534418387471,4.12738891077874));
#57061=CARTESIAN_POINT('Ctrl Pts',(-10.0159871075715,12.98719611739,4.11258330249198));
#57062=CARTESIAN_POINT('Ctrl Pts',(-10.0135512354019,12.9902955808623,4.38741669750803));
#57063=CARTESIAN_POINT('Ctrl Pts',(-10.0138145339143,12.5850052295903,4.4129424273693));
#57064=CARTESIAN_POINT('Ctrl Pts',(-9.92124134238478,12.1798000932329,4.43846815723057));
#57065=CARTESIAN_POINT('Ctrl Pts',(-9.73520837540778,11.8234099166911,4.46399388709184));
#57066=CARTESIAN_POINT('Ctrl Pts',(-9.35379976449056,11.0927314547595,4.51632726287592));
#57067=CARTESIAN_POINT('Ctrl Pts',(-8.57954193321014,10.5672420039701,4.56866063866001));
#57068=CARTESIAN_POINT('Ctrl Pts',(-7.75970071708304,10.482369764132,4.62099401444409));
#57069=CARTESIAN_POINT('Ctrl Pts',(-6.93985950095593,10.3974975242939,4.67332739022817));
#57070=CARTESIAN_POINT('Ctrl Pts',(-6.07443489998217,10.7532424954071,4.72566076601226));
#57071=CARTESIAN_POINT('Ctrl Pts',(-5.55138100127894,11.3901954309976,4.77799414179634));
#57072=CARTESIAN_POINT('Ctrl Pts',(-5.02832710257572,12.0271483665881,4.83032751758043));
#57073=CARTESIAN_POINT('Ctrl Pts',(-4.84764390614303,12.945309266656,4.88266089336452));
#57074=CARTESIAN_POINT('Ctrl Pts',(-5.09037388542358,13.7329699193423,4.9349942691486));
#57075=CARTESIAN_POINT('Ctrl Pts',(-5.33310386470412,14.5206305720287,4.98732764493268));
#57076=CARTESIAN_POINT('Ctrl Pts',(-5.9992470196979,15.1777909773334,5.03966102071676));
#57077=CARTESIAN_POINT('Ctrl Pts',(-6.79011836385736,15.4098338158843,5.09199439650085));
#57078=CARTESIAN_POINT('Ctrl Pts',(-7.58098970801682,15.6418766544352,5.14432777228493));
#57079=CARTESIAN_POINT('Ctrl Pts',(-8.49658924134195,15.4488019262325,5.19666114806902));
#57080=CARTESIAN_POINT('Ctrl Pts',(-9.12641195891838,14.9171634974037,5.24899452385311));
#57081=CARTESIAN_POINT('Ctrl Pts',(-9.68170723832013,14.4484342794212,5.29513524840475));
#57082=CARTESIAN_POINT('Ctrl Pts',(-10.0148566122412,13.7165257701398,5.34127597295639));
#57083=CARTESIAN_POINT('Ctrl Pts',(-10.0201376030965,12.9888406983805,5.38741669750803));
#57084=CARTESIAN_POINT('Origin',(-7.5,12.9903810567666,7.5));
#57085=CARTESIAN_POINT('',(-10.0170827477036,12.9925476830062,6.38741669750803));
#57086=CARTESIAN_POINT('',(-10.0137187170915,12.9909479514162,6.11258330249198));
#57087=CARTESIAN_POINT('',(-10.0175,12.9903810567666,7.5));
#57088=CARTESIAN_POINT('Ctrl Pts',(-10.0137187170915,12.9909479514162,6.11258330249198));
#57089=CARTESIAN_POINT('Ctrl Pts',(-10.0144982588899,13.3697154315319,6.08872275352109));
#57090=CARTESIAN_POINT('Ctrl Pts',(-9.93406587049998,13.7481685539756,6.06486220455019));
#57091=CARTESIAN_POINT('Ctrl Pts',(-9.77069359762705,14.0865814419388,6.0410016555793));
#57092=CARTESIAN_POINT('Ctrl Pts',(-9.41236896061271,14.8288229074456,5.98866827979521));
#57093=CARTESIAN_POINT('Ctrl Pts',(-8.65505611306826,15.3784479785104,5.93633490401113));
#57094=CARTESIAN_POINT('Ctrl Pts',(-7.83829989006264,15.4890315871854,5.88400152822704));
#57095=CARTESIAN_POINT('Ctrl Pts',(-7.02154366705702,15.5996151958603,5.83166815244296));
#57096=CARTESIAN_POINT('Ctrl Pts',(-6.14534406859022,15.2711573421455,5.77933477665887));
#57097=CARTESIAN_POINT('Ctrl Pts',(-5.60254941260429,14.6509198275943,5.72700140087479));
#57098=CARTESIAN_POINT('Ctrl Pts',(-5.05975475661836,14.0306823130431,5.6746680250907));
#57099=CARTESIAN_POINT('Ctrl Pts',(-4.8503650431133,13.1186651376555,5.62233464930662));
#57100=CARTESIAN_POINT('Ctrl Pts',(-5.06826110556232,12.3237831148942,5.57000127352254));
#57101=CARTESIAN_POINT('Ctrl Pts',(-5.28615716801134,11.5289010921329,5.51766789773845));
#57102=CARTESIAN_POINT('Ctrl Pts',(-5.93133900641445,10.8511542219977,5.46533452195436));
#57103=CARTESIAN_POINT('Ctrl Pts',(-6.71453634454677,10.5943988157391,5.41300114617028));
#57104=CARTESIAN_POINT('Ctrl Pts',(-7.49773368267909,10.3376434094805,5.3606677703862));
#57105=CARTESIAN_POINT('Ctrl Pts',(-8.41894652054063,10.5018794670985,5.30833439460211));
#57106=CARTESIAN_POINT('Ctrl Pts',(-9.06514447594766,11.0134998219879,5.25600101881803));
#57107=CARTESIAN_POINT('Ctrl Pts',(-9.65543848794614,11.4808588245671,5.20819511337601));
#57108=CARTESIAN_POINT('Ctrl Pts',(-10.0162435426697,12.2380961764306,5.160389207934));
#57109=CARTESIAN_POINT('Ctrl Pts',(-10.0207017684327,12.9915893349038,5.11258330249198));
#57110=CARTESIAN_POINT('Ctrl Pts',(-10.0201376030965,12.9888406983805,5.38741669750803));
#57111=CARTESIAN_POINT('Ctrl Pts',(-10.02084637685,12.8911764354056,5.39360934874047));
#57112=CARTESIAN_POINT('Ctrl Pts',(-10.0156492795336,12.793588248926,5.39980199997291));
#57113=CARTESIAN_POINT('Ctrl Pts',(-10.0042907210835,12.6967226001492,5.40599465120536));
#57114=CARTESIAN_POINT('Ctrl Pts',(-9.90830086384453,11.8781222611782,5.45832802698944));
#57115=CARTESIAN_POINT('Ctrl Pts',(-9.37227524753879,11.1111237126909,5.51066140277353));
#57116=CARTESIAN_POINT('Ctrl Pts',(-8.63654573295752,10.739611267924,5.56299477855761));
#57117=CARTESIAN_POINT('Ctrl Pts',(-7.90081621837627,10.368098823157,5.6153281543417));
#57118=CARTESIAN_POINT('Ctrl Pts',(-6.96538280551948,10.3920724821103,5.66766153012578));
#57119=CARTESIAN_POINT('Ctrl Pts',(-6.24965042528476,10.8007851576184,5.71999490590986));
#57120=CARTESIAN_POINT('Ctrl Pts',(-5.53391804505003,11.2094978331266,5.77232828169395));
#57121=CARTESIAN_POINT('Ctrl Pts',(-5.03788669743737,12.0029495251895,5.82466165747803));
#57122=CARTESIAN_POINT('Ctrl Pts',(-4.98395499247446,12.8253915347154,5.87699503326212));
#57123=CARTESIAN_POINT('Ctrl Pts',(-4.93002328751154,13.6478335442413,5.9293284090462));
#57124=CARTESIAN_POINT('Ctrl Pts',(-5.31819122519835,14.4992658712303,5.98166178483029));
#57125=CARTESIAN_POINT('Ctrl Pts',(-5.97442155431181,14.997945170426,6.03399516061437));
#57126=CARTESIAN_POINT('Ctrl Pts',(-6.63065188342527,15.4966244696218,6.08632853639846));
#57127=CARTESIAN_POINT('Ctrl Pts',(-7.55494460396538,15.6425507410243,6.13866191218253));
#57128=CARTESIAN_POINT('Ctrl Pts',(-8.33288879152928,15.3702970248207,6.19099528796662));
#57129=CARTESIAN_POINT('Ctrl Pts',(-9.11083297909318,15.0980433086171,6.2433286637507));
#57130=CARTESIAN_POINT('Ctrl Pts',(-9.74242863368087,14.4076096048073,6.2956620395348));
#57131=CARTESIAN_POINT('Ctrl Pts',(-9.94449673701248,13.6085552867894,6.34799541531888));
#57132=CARTESIAN_POINT('Ctrl Pts',(-9.99523417179805,13.4079201262562,6.36113584271526));
#57133=CARTESIAN_POINT('Ctrl Pts',(-10.0188913666349,13.2004368082823,6.37427627011165));
#57134=CARTESIAN_POINT('Ctrl Pts',(-10.0170827477036,12.9925476830062,6.38741669750803));
#57135=CARTESIAN_POINT('Origin',(-7.5,12.9903810567666,7.5));
#57136=CARTESIAN_POINT('',(-10.0145080012689,12.9889431840086,7.38741669750803));
#57137=CARTESIAN_POINT('',(-10.0189159587739,12.9883983308864,7.11258330249199));
#57138=CARTESIAN_POINT('',(-10.0175,12.9903810567666,7.5));
#57139=CARTESIAN_POINT('Ctrl Pts',(-10.0189159587739,12.9883983308864,7.11258330249199));
#57140=CARTESIAN_POINT('Ctrl Pts',(-10.0130302121016,13.6704662986594,7.06938967489226));
#57141=CARTESIAN_POINT('Ctrl Pts',(-9.72554840383075,14.3569089324365,7.02619604729254));
#57142=CARTESIAN_POINT('Ctrl Pts',(-9.2308848153494,14.8238864031427,6.98300241969281));
#57143=CARTESIAN_POINT('Ctrl Pts',(-8.63155067970796,15.3896760534967,6.93066904390873));
#57144=CARTESIAN_POINT('Ctrl Pts',(-7.72807923358486,15.6332967159553,6.87833566812465));
#57145=CARTESIAN_POINT('Ctrl Pts',(-6.9255462333781,15.4455199330078,6.82600229234057));
#57146=CARTESIAN_POINT('Ctrl Pts',(-6.12301323317133,15.2577431500604,6.77366891655648));
#57147=CARTESIAN_POINT('Ctrl Pts',(-5.4214186788809,14.638568921707,6.72133554077239));
#57148=CARTESIAN_POINT('Ctrl Pts',(-5.13532585476554,13.8656069146025,6.66900216498831));
#57149=CARTESIAN_POINT('Ctrl Pts',(-4.84923303065017,13.092644907498,6.61666878920422));
#57150=CARTESIAN_POINT('Ctrl Pts',(-4.97864193670987,12.1658951216425,6.56433541342014));
#57151=CARTESIAN_POINT('Ctrl Pts',(-5.46553146829354,11.5008704033029,6.51200203763605));
#57152=CARTESIAN_POINT('Ctrl Pts',(-5.95242099987721,10.8358456849633,6.45966866185197));
#57153=CARTESIAN_POINT('Ctrl Pts',(-6.79679115698486,10.4325460341398,6.40733528606789));
#57154=CARTESIAN_POINT('Ctrl Pts',(-7.62006453112491,10.471792520931,6.35500191028381));
#57155=CARTESIAN_POINT('Ctrl Pts',(-8.44333790526497,10.5110390077222,6.30266853449972));
#57156=CARTESIAN_POINT('Ctrl Pts',(-9.24551449643742,10.9928316321281,6.25033515871563));
#57157=CARTESIAN_POINT('Ctrl Pts',(-9.66693457878153,11.7011568743055,6.19800178293155));
#57158=CARTESIAN_POINT('Ctrl Pts',(-9.89621504923482,12.0865327772692,6.16952895611836));
#57159=CARTESIAN_POINT('Ctrl Pts',(-10.0127884887617,12.5389641820168,6.14105612930517));
#57160=CARTESIAN_POINT('Ctrl Pts',(-10.0137187170915,12.9909479514162,6.11258330249198));
#57161=CARTESIAN_POINT('Ctrl Pts',(-10.0170827477036,12.9925476830062,6.38741669750803));
#57162=CARTESIAN_POINT('Ctrl Pts',(-10.0116883182615,12.3724926793498,6.42660964589573));
#57163=CARTESIAN_POINT('Ctrl Pts',(-9.77974890631033,11.7488275963524,6.46580259428343));
#57164=CARTESIAN_POINT('Ctrl Pts',(-9.36410096710587,11.2924908434457,6.50499554267113));
#57165=CARTESIAN_POINT('Ctrl Pts',(-8.80909654179214,10.6831556503463,6.55732891845521));
#57166=CARTESIAN_POINT('Ctrl Pts',(-7.92654713908917,10.3721601963736,6.6096622942393));
#57167=CARTESIAN_POINT('Ctrl Pts',(-7.11214799700031,10.4989408139477,6.66199567002338));
#57168=CARTESIAN_POINT('Ctrl Pts',(-6.29774885491145,10.6257214315218,6.71432904580747));
#57169=CARTESIAN_POINT('Ctrl Pts',(-5.55149997343671,11.1902781206427,6.76666242159156));
#57170=CARTESIAN_POINT('Ctrl Pts',(-5.20798562845119,11.9394891669376,6.81899579737564));
#57171=CARTESIAN_POINT('Ctrl Pts',(-4.86447128346568,12.6887002132326,6.87132917315972));
#57172=CARTESIAN_POINT('Ctrl Pts',(-4.92369147496937,13.6225656167016,6.92366254894381));
#57173=CARTESIAN_POINT('Ctrl Pts',(-5.35909454078469,14.3223823516912,6.97599592472789));
#57174=CARTESIAN_POINT('Ctrl Pts',(-5.79449760660002,15.0221990866808,7.02832930051197));
#57175=CARTESIAN_POINT('Ctrl Pts',(-6.60608354672698,15.4879671531909,7.08066267629606));
#57176=CARTESIAN_POINT('Ctrl Pts',(-7.42997391459192,15.5108572005546,7.13299605208014));
#57177=CARTESIAN_POINT('Ctrl Pts',(-8.25386428245684,15.5337472479183,7.18532942786423));
#57178=CARTESIAN_POINT('Ctrl Pts',(-9.09005907805975,15.1137592761355,7.23766280364831));
#57179=CARTESIAN_POINT('Ctrl Pts',(-9.56364635237551,14.4391969089269,7.2899961794324));
#57180=CARTESIAN_POINT('Ctrl Pts',(-9.85751310519891,14.0206226287906,7.32246968545761));
#57181=CARTESIAN_POINT('Ctrl Pts',(-10.0117630617271,13.5040281493434,7.35494319148282));
#57182=CARTESIAN_POINT('Ctrl Pts',(-10.0145080012689,12.9889431840086,7.38741669750803));
#57183=CARTESIAN_POINT('Origin',(-7.5,12.9903810567666,7.5));
#57184=CARTESIAN_POINT('',(-10.0214370846894,12.9902333726245,8.38741669750803));
#57185=CARTESIAN_POINT('',(-10.0184390483887,12.992460268524,8.11258330249199));
#57186=CARTESIAN_POINT('',(-10.0175,12.9903810567666,7.5));
#57187=CARTESIAN_POINT('Ctrl Pts',(-10.0184390483887,12.992460268524,8.11258330249199));
#57188=CARTESIAN_POINT('Ctrl Pts',(-10.0198617859934,13.1535014782239,8.10238997204752));
#57189=CARTESIAN_POINT('Ctrl Pts',(-10.0057048345233,13.3142936934228,8.09219664160306));
#57190=CARTESIAN_POINT('Ctrl Pts',(-9.9750487925512,13.4718761813451,8.08200331115859));
#57191=CARTESIAN_POINT('Ctrl Pts',(-9.8176582151223,14.2809173090076,8.02966993537451));
#57192=CARTESIAN_POINT('Ctrl Pts',(-9.22537175290504,15.0053539438514,7.97733655959042));
#57193=CARTESIAN_POINT('Ctrl Pts',(-8.46374388225838,15.3203814452906,7.92500318380634));
#57194=CARTESIAN_POINT('Ctrl Pts',(-7.70211601161172,15.6354089467299,7.87266980802225));
#57195=CARTESIAN_POINT('Ctrl Pts',(-6.77114673253565,15.5410273147647,7.82033643223817));
#57196=CARTESIAN_POINT('Ctrl Pts',(-6.08824058698168,15.0795530074754,7.76800305645409));
#57197=CARTESIAN_POINT('Ctrl Pts',(-5.40533444142772,14.6180787001861,7.71566968067));
#57198=CARTESIAN_POINT('Ctrl Pts',(-4.97049142939586,13.7895117175727,7.66333630488591));
#57199=CARTESIAN_POINT('Ctrl Pts',(-4.97867550117357,12.9653440395039,7.61100292910182));
#57200=CARTESIAN_POINT('Ctrl Pts',(-4.98685957295128,12.1411763614351,7.55866955331774));
#57201=CARTESIAN_POINT('Ctrl Pts',(-5.43807072853852,11.3214079879109,7.50633617753367));
#57202=CARTESIAN_POINT('Ctrl Pts',(-6.13000628195668,10.8735860038557,7.45400280174958));
#57203=CARTESIAN_POINT('Ctrl Pts',(-6.82194183537485,10.4257640198005,7.4016694259655));
#57204=CARTESIAN_POINT('Ctrl Pts',(-7.75460178662392,10.3498884252143,7.3493360501814));
#57205=CARTESIAN_POINT('Ctrl Pts',(-8.50982357282137,10.6799784021981,7.29700267439732));
#57206=CARTESIAN_POINT('Ctrl Pts',(-9.2650453590188,11.0100683791819,7.24466929861323));
#57207=CARTESIAN_POINT('Ctrl Pts',(-9.84282898016461,11.7461239277358,7.19233592282916));
#57208=CARTESIAN_POINT('Ctrl Pts',(-9.98412237815762,12.5581310211375,7.14000254704507));
#57209=CARTESIAN_POINT('Ctrl Pts',(-10.0087985252324,12.6999437791798,7.13086279886071));
#57210=CARTESIAN_POINT('Ctrl Pts',(-10.020161379579,12.8440731186622,7.12172305067635));
#57211=CARTESIAN_POINT('Ctrl Pts',(-10.0189159587739,12.9883983308864,7.11258330249199));
#57212=CARTESIAN_POINT('Ctrl Pts',(-10.0145080012689,12.9889431840086,7.38741669750803));
#57213=CARTESIAN_POINT('Ctrl Pts',(-10.0161867279748,12.6739319154882,7.4072765672669));
#57214=CARTESIAN_POINT('Ctrl Pts',(-9.96119959962244,12.359485234924,7.42713643702578));
#57215=CARTESIAN_POINT('Ctrl Pts',(-9.84682730754632,12.0683695443894,7.44699630678465));
#57216=CARTESIAN_POINT('Ctrl Pts',(-9.54544123537271,11.3012413096949,7.49932968256874));
#57217=CARTESIAN_POINT('Ctrl Pts',(-8.83168933799688,10.6961216029404,7.55166305835282));
#57218=CARTESIAN_POINT('Ctrl Pts',(-8.02558570196195,10.5243187478344,7.60399643413691));
#57219=CARTESIAN_POINT('Ctrl Pts',(-7.21948206592701,10.3525158927284,7.65632980992099));
#57220=CARTESIAN_POINT('Ctrl Pts',(-6.32102669123297,10.6140298892709,7.70866318570508));
#57221=CARTESIAN_POINT('Ctrl Pts',(-5.73304635500187,11.1916096823396,7.76099656148916));
#57222=CARTESIAN_POINT('Ctrl Pts',(-5.14506601877077,11.7691894754082,7.81332993727325));
#57223=CARTESIAN_POINT('Ctrl Pts',(-4.8675607210026,12.6628350650029,7.86566331305733));
#57224=CARTESIAN_POINT('Ctrl Pts',(-5.02495129299175,13.4718761647033,7.91799668884141));
#57225=CARTESIAN_POINT('Ctrl Pts',(-5.18234186498089,14.2809172644038,7.9703300646255));
#57226=CARTESIAN_POINT('Ctrl Pts',(-5.77462830672734,15.0053538742101,8.02266344040958));
#57227=CARTESIAN_POINT('Ctrl Pts',(-6.53625615105054,15.3203813647611,8.07499681619367));
#57228=CARTESIAN_POINT('Ctrl Pts',(-7.29788399537374,15.6354088553122,8.12733019197775));
#57229=CARTESIAN_POINT('Ctrl Pts',(-8.22885324227368,15.5410272266082,8.17966356776184));
#57230=CARTESIAN_POINT('Ctrl Pts',(-8.91175936422494,15.0795529352688,8.23199694354592));
#57231=CARTESIAN_POINT('Ctrl Pts',(-9.58779130918474,14.6227238738573,8.28380352819996));
#57232=CARTESIAN_POINT('Ctrl Pts',(-10.0207290328118,13.8061553106607,8.33561011285399));
#57233=CARTESIAN_POINT('Ctrl Pts',(-10.0214370846894,12.9902333726245,8.38741669750803));
#57234=CARTESIAN_POINT('Origin',(-7.5,12.9903810567666,7.5));
#57235=CARTESIAN_POINT('',(-10.0148245050326,12.9920058624485,9.38741669750802));
#57236=CARTESIAN_POINT('',(-10.0138587145805,12.9895659971561,9.11258330249198));
#57237=CARTESIAN_POINT('',(-10.0175,12.9903810567666,7.5));
#57238=CARTESIAN_POINT('Ctrl Pts',(-10.0138587145805,12.9895659971561,9.11258330249198));
#57239=CARTESIAN_POINT('Ctrl Pts',(-10.0124665205819,13.458209000479,9.08305689341869));
#57240=CARTESIAN_POINT('Ctrl Pts',(-9.88655927300326,13.9275468726326,9.0535304843454));
#57241=CARTESIAN_POINT('Ctrl Pts',(-9.64090553321082,14.3223823977307,9.02400407527211));
#57242=CARTESIAN_POINT('Ctrl Pts',(-9.20550245234811,15.0221991569096,8.97167069948803));
#57243=CARTESIAN_POINT('Ctrl Pts',(-8.39391648416845,15.4879672395126,8.91933732370394));
#57244=CARTESIAN_POINT('Ctrl Pts',(-7.57002608782754,15.5108572876662,8.86700394791986));
#57245=CARTESIAN_POINT('Ctrl Pts',(-6.74613569148664,15.5337473358198,8.81467057213577));
#57246=CARTESIAN_POINT('Ctrl Pts',(-5.90994086698447,15.113759349524,8.76233719635169));
#57247=CARTESIAN_POINT('Ctrl Pts',(-5.43635357630086,14.4391969590017,8.71000382056761));
#57248=CARTESIAN_POINT('Ctrl Pts',(-4.96276628561725,13.7646345684795,8.65767044478352));
#57249=CARTESIAN_POINT('Ctrl Pts',(-4.85178652875219,12.8354977737306,8.60533706899943));
#57250=CARTESIAN_POINT('Ctrl Pts',(-5.15317261134217,12.0683695125223,8.55300369321535));
#57251=CARTESIAN_POINT('Ctrl Pts',(-5.45455869393216,11.3012412513139,8.50067031743126));
#57252=CARTESIAN_POINT('Ctrl Pts',(-6.16831061597719,10.696121523646,8.44833694164718));
#57253=CARTESIAN_POINT('Ctrl Pts',(-6.97441427987286,10.5243186626023,8.3960035658631));
#57254=CARTESIAN_POINT('Ctrl Pts',(-7.78051794376854,10.3525158015586,8.34367019007901));
#57255=CARTESIAN_POINT('Ctrl Pts',(-8.67897334951486,10.6140298071391,8.29133681429493));
#57256=CARTESIAN_POINT('Ctrl Pts',(-9.26695370606775,11.1916096201701,8.23900343851084));
#57257=CARTESIAN_POINT('Ctrl Pts',(-9.74040909687172,11.656690252629,8.19686339317122));
#57258=CARTESIAN_POINT('Ctrl Pts',(-10.0125573370586,12.3267029956413,8.15472334783161));
#57259=CARTESIAN_POINT('Ctrl Pts',(-10.0184390483887,12.992460268524,8.11258330249199));
#57260=CARTESIAN_POINT('Ctrl Pts',(-10.0214370846894,12.9902333726245,8.38741669750803));
#57261=CARTESIAN_POINT('Ctrl Pts',(-10.0214442844586,12.9819367353796,8.38794348863807));
#57262=CARTESIAN_POINT('Ctrl Pts',(-10.0214067930746,12.9736401649937,8.38847027976812));
#57263=CARTESIAN_POINT('Ctrl Pts',(-10.021324411684,12.9653440403702,8.38899707089817));
#57264=CARTESIAN_POINT('Ctrl Pts',(-10.0131403401893,12.1411763907856,8.44133044668226));
#57265=CARTESIAN_POINT('Ctrl Pts',(-9.56192920019726,11.3214080455913,8.49366382246634));
#57266=CARTESIAN_POINT('Ctrl Pts',(-8.86999367069368,10.873586077015,8.54599719825042));
#57267=CARTESIAN_POINT('Ctrl Pts',(-8.1780581411901,10.4257641084388,8.59833057403451));
#57268=CARTESIAN_POINT('Ctrl Pts',(-7.24539822217496,10.3498885164806,8.65066394981859));
#57269=CARTESIAN_POINT('Ctrl Pts',(-6.49017646207993,10.6799784820534,8.70299732560268));
#57270=CARTESIAN_POINT('Ctrl Pts',(-5.7349547019849,11.0100684476262,8.75533070138676));
#57271=CARTESIAN_POINT('Ctrl Pts',(-5.15717110080998,11.7461239707299,8.80766407717085));
#57272=CARTESIAN_POINT('Ctrl Pts',(-5.01587770769964,12.5581310360714,8.85999745295494));
#57273=CARTESIAN_POINT('Ctrl Pts',(-4.8745843145893,13.3701381014129,8.91233082873902));
#57274=CARTESIAN_POINT('Ctrl Pts',(-5.16978112954355,14.2580967089923,8.96466420452309));
#57275=CARTESIAN_POINT('Ctrl Pts',(-5.76911524447212,14.823886339783,9.01699758030718));
#57276=CARTESIAN_POINT('Ctrl Pts',(-6.36844935940068,15.3896759705738,9.06933095609126));
#57277=CARTESIAN_POINT('Ctrl Pts',(-7.27192077430355,15.633296624576,9.12166433187536));
#57278=CARTESIAN_POINT('Ctrl Pts',(-8.07445374677037,15.4455198481341,9.17399770765944));
#57279=CARTESIAN_POINT('Ctrl Pts',(-8.87698671923719,15.2577430716922,9.22633108344353));
#57280=CARTESIAN_POINT('Ctrl Pts',(-9.57858124926796,14.6385688648061,9.2786644592276));
#57281=CARTESIAN_POINT('Ctrl Pts',(-9.8646740635007,13.8656068843882,9.33099783501169));
#57282=CARTESIAN_POINT('Ctrl Pts',(-9.96748309569448,13.5878387295239,9.34980412251046));
#57283=CARTESIAN_POINT('Ctrl Pts',(-10.0166357361991,13.2902109767329,9.36861041000924));
#57284=CARTESIAN_POINT('Ctrl Pts',(-10.0148245050326,12.9920058624485,9.38741669750802));
#57285=CARTESIAN_POINT('Origin',(-7.5,12.9903810567666,7.5));
#57286=CARTESIAN_POINT('',(-10.0166112816083,12.988245230306,10.387416697508));
#57287=CARTESIAN_POINT('',(-10.0209918820407,12.9894441341194,10.112583302492));
#57288=CARTESIAN_POINT('',(-10.0175,12.9903810567666,7.5));
#57289=CARTESIAN_POINT('Ctrl Pts',(-10.0209918820407,12.9894441341194,10.112583302492));
#57290=CARTESIAN_POINT('Ctrl Pts',(-10.0172624812131,13.7593153446234,10.0637238147899));
#57291=CARTESIAN_POINT('Ctrl Pts',(-9.63824829706051,14.5323682430672,10.0148643270877));
#57292=CARTESIAN_POINT('Ctrl Pts',(-9.02557849846605,14.9979452399236,9.96600483938563));
#57293=CARTESIAN_POINT('Ctrl Pts',(-8.36934814670953,15.4966245564456,9.91367146360154));
#57294=CARTESIAN_POINT('Ctrl Pts',(-7.44505539412875,15.642550832678,9.86133808781746));
#57295=CARTESIAN_POINT('Ctrl Pts',(-6.66711117965626,15.3702971070154,9.80900471203338));
#57296=CARTESIAN_POINT('Ctrl Pts',(-5.88916696518377,15.0980433813528,9.75667133624929));
#57297=CARTESIAN_POINT('Ctrl Pts',(-5.25757128881956,14.4076096537953,9.70433796046521));
#57298=CARTESIAN_POINT('Ctrl Pts',(-5.05550317851592,13.608555308187,9.65200458468112));
#57299=CARTESIAN_POINT('Ctrl Pts',(-4.85343506821227,12.8095009625786,9.59967120889704));
#57300=CARTESIAN_POINT('Ctrl Pts',(-5.08089452396919,11.9018259989194,9.54733783311296));
#57301=CARTESIAN_POINT('Ctrl Pts',(-5.6358989684585,11.2924907847457,9.49500445732887));
#57302=CARTESIAN_POINT('Ctrl Pts',(-6.19090341294781,10.683155570572,9.44267108154479));
#57303=CARTESIAN_POINT('Ctrl Pts',(-7.0734528461695,10.3721601058839,9.3903377057607));
#57304=CARTESIAN_POINT('Ctrl Pts',(-7.88785201640932,10.4989407278476,9.33800432997662));
#57305=CARTESIAN_POINT('Ctrl Pts',(-8.70225118664915,10.6257213498112,9.28567095419253));
#57306=CARTESIAN_POINT('Ctrl Pts',(-9.44850009390711,11.1902780584266,9.23333757840845));
#57307=CARTESIAN_POINT('Ctrl Pts',(-9.79201445076321,11.9394891306117,9.18100420262436));
#57308=CARTESIAN_POINT('Ctrl Pts',(-9.9417185427335,12.2659964832652,9.15819723591357));
#57309=CARTESIAN_POINT('Ctrl Pts',(-10.014934081453,12.6275739462602,9.13539026920278));
#57310=CARTESIAN_POINT('Ctrl Pts',(-10.0138587145805,12.9895659971561,9.11258330249198));
#57311=CARTESIAN_POINT('Ctrl Pts',(-10.0148245050326,12.9920058624485,9.38741669750802));
#57312=CARTESIAN_POINT('Ctrl Pts',(-10.0115955154073,12.4603778526996,9.42094378579333));
#57313=CARTESIAN_POINT('Ctrl Pts',(-9.84639154112273,11.9269148544392,9.45447087407864));
#57314=CARTESIAN_POINT('Ctrl Pts',(-9.53446846140197,11.5008704547181,9.48799796236395));
#57315=CARTESIAN_POINT('Ctrl Pts',(-9.0475789466358,10.8358457594159,9.54033133814803));
#57316=CARTESIAN_POINT('Ctrl Pts',(-8.20320881866876,10.4325461227612,9.59266471393211));
#57317=CARTESIAN_POINT('Ctrl Pts',(-7.37993547300324,10.4717926080996,9.64499808971619));
#57318=CARTESIAN_POINT('Ctrl Pts',(-6.55666212733773,10.5110390934381,9.69733146550028));
#57319=CARTESIAN_POINT('Ctrl Pts',(-5.75448556397372,10.9928317007697,9.74966484128437));
#57320=CARTESIAN_POINT('Ctrl Pts',(-5.33306549615464,11.7011569186411,9.80199821706845));
#57321=CARTESIAN_POINT('Ctrl Pts',(-4.91164542833556,12.4094821365125,9.85433159285254));
#57322=CARTESIAN_POINT('Ctrl Pts',(-4.87098185606138,13.3443399649238,9.90666496863662));
#57323=CARTESIAN_POINT('Ctrl Pts',(-5.22930648076992,14.0865814044601,9.9589983444207));
#57324=CARTESIAN_POINT('Ctrl Pts',(-5.58763110547847,14.8288228439964,10.0113317202048));
#57325=CARTESIAN_POINT('Ctrl Pts',(-6.34494392716974,15.3784478946578,10.0636650959889));
#57326=CARTESIAN_POINT('Ctrl Pts',(-7.1617001217923,15.489031500081,10.115998471773));
#57327=CARTESIAN_POINT('Ctrl Pts',(-7.97845631641486,15.5996151055041,10.168331847557));
#57328=CARTESIAN_POINT('Ctrl Pts',(-8.8546558839687,15.2711572656891,10.2206652233411));
#57329=CARTESIAN_POINT('Ctrl Pts',(-9.39745052149691,14.6509197715574,10.2729985991252));
#57330=CARTESIAN_POINT('Ctrl Pts',(-9.79302682634298,14.1989048858303,10.3111379652528));
#57331=CARTESIAN_POINT('Ctrl Pts',(-10.0115264151771,13.5919211369207,10.3492773313804));
#57332=CARTESIAN_POINT('Ctrl Pts',(-10.0166112816083,12.988245230306,10.387416697508));
#57333=CARTESIAN_POINT('Origin',(-7.5,12.9903810567666,7.5));
#57334=CARTESIAN_POINT('',(-10.020507596494,12.9916292754481,11.387416697508));
#57335=CARTESIAN_POINT('',(-10.0159019782719,12.9923925656114,11.112583302492));
#57336=CARTESIAN_POINT('',(-10.0175,12.9903810567666,7.5));
#57337=CARTESIAN_POINT('',(-5.58653400333491,14.6263682601415,12.));
#57338=CARTESIAN_POINT('Ctrl Pts',(-10.020507596494,12.9916292754481,11.387416697508));
#57339=CARTESIAN_POINT('Ctrl Pts',(-10.0157033908479,12.2477735308672,11.4346110043198));
#57340=CARTESIAN_POINT('Ctrl Pts',(-9.66521700262529,11.5001788657538,11.4818053111315));
#57341=CARTESIAN_POINT('Ctrl Pts',(-9.08783233623607,11.0319150553912,11.5289996179432));
#57342=CARTESIAN_POINT('Ctrl Pts',(-8.44757526373259,10.5126611959891,11.5813329937273));
#57343=CARTESIAN_POINT('Ctrl Pts',(-7.52831480323821,10.3368839617759,11.6336663695114));
#57344=CARTESIAN_POINT('Ctrl Pts',(-6.74219715513642,10.5850674081367,11.6859997452955));
#57345=CARTESIAN_POINT('Ctrl Pts',(-5.95607950703463,10.8332508544976,11.7383331210796));
#57346=CARTESIAN_POINT('Ctrl Pts',(-5.30310467132541,11.5053949814325,11.7906664968637));
#57347=CARTESIAN_POINT('Ctrl Pts',(-5.07623184554712,12.2963777181293,11.8429998726477));
#57348=CARTESIAN_POINT('Ctrl Pts',(-4.84935901976883,13.0873604548261,11.8953332484318));
#57349=CARTESIAN_POINT('Ctrl Pts',(-5.04858820392146,13.9971818012847,11.9476666242159));
#57350=CARTESIAN_POINT('Ctrl Pts',(-5.58653400333491,14.6263682601415,12.));
#57351=CARTESIAN_POINT('',(-9.41699350863879,14.6286916542883,12.));
#57352=CARTESIAN_POINT('Origin',(-7.5,12.9903810567666,12.));
#57353=CARTESIAN_POINT('Ctrl Pts',(-9.41700728965905,14.6287007311509,12.));
#57354=CARTESIAN_POINT('Ctrl Pts',(-8.90328417076102,15.2258393704274,11.9500021225376));
#57355=CARTESIAN_POINT('Ctrl Pts',(-8.08591167026785,15.5661089832965,11.9000042450751));
#57356=CARTESIAN_POINT('Ctrl Pts',(-7.30082070927967,15.5037710574514,11.8500063676127));
#57357=CARTESIAN_POINT('Ctrl Pts',(-6.47905661905513,15.438521205569,11.7976729918286));
#57358=CARTESIAN_POINT('Ctrl Pts',(-5.6926603741346,14.9321721568753,11.7453396160445));
#57359=CARTESIAN_POINT('Ctrl Pts',(-5.29374195236929,14.2110639499398,11.6930062402604));
#57360=CARTESIAN_POINT('Ctrl Pts',(-4.89482353060398,13.4899557430043,11.6406728644763));
#57361=CARTESIAN_POINT('Ctrl Pts',(-4.88338293199389,12.554088377827,11.5883394886922));
#57362=CARTESIAN_POINT('Ctrl Pts',(-5.26479155556264,11.8234099202509,11.5360061129082));
#57363=CARTESIAN_POINT('Ctrl Pts',(-5.64620017913138,11.0927314626748,11.4836727371241));
#57364=CARTESIAN_POINT('Ctrl Pts',(-6.42045802487898,10.5672419126997,11.43133936134));
#57365=CARTESIAN_POINT('Ctrl Pts',(-7.24029926801916,10.482369652534,11.3790059855559));
#57366=CARTESIAN_POINT('Ctrl Pts',(-8.06014051115934,10.3974973923684,11.3266726097718));
#57367=CARTESIAN_POINT('Ctrl Pts',(-8.92556515169212,10.753242422012,11.2743392339877));
#57368=CARTESIAN_POINT('Ctrl Pts',(-9.44861906997071,11.3901953896836,11.2220058582037));
#57369=CARTESIAN_POINT('Ctrl Pts',(-9.81316588581269,11.8341251034117,11.1855316729664));
#57370=CARTESIAN_POINT('Ctrl Pts',(-10.0114057826858,12.4146518528183,11.1490574877292));
#57371=CARTESIAN_POINT('Ctrl Pts',(-10.0159019782719,12.9923925656114,11.112583302492));
#57372=CARTESIAN_POINT('Origin',(-7.5,12.9903810567666,14.2084234471775));
#57373=CARTESIAN_POINT('',(-10.5774088918681,12.99185618799,4.79157655282255));
#57374=CARTESIAN_POINT('',(-10.5686791348591,12.9902767031652,4.70842344717746));
#57375=CARTESIAN_POINT('',(-10.5735,12.9903810567666,14.2084234471775));
#57376=CARTESIAN_POINT('',(-6.70620071746715,10.0211581030209,4.));
#57377=CARTESIAN_POINT('Ctrl Pts',(-10.5686791348591,12.9902767031652,4.70842344717746));
#57378=CARTESIAN_POINT('Ctrl Pts',(-10.568341542465,13.509926201974,4.68161580125464));
#57379=CARTESIAN_POINT('Ctrl Pts',(-10.1982938594512,15.0443643081101,4.60247477954774));
#57380=CARTESIAN_POINT('Ctrl Pts',(-7.78634777823694,16.5973803971072,4.47100038205676));
#57381=CARTESIAN_POINT('Ctrl Pts',(-4.64704915358778,15.2208104036021,4.31400025470451));
#57382=CARTESIAN_POINT('Ctrl Pts',(-4.07060765975928,11.8373819589561,4.15700012735225));
#57383=CARTESIAN_POINT('Ctrl Pts',(-5.72985994157694,10.2821754194981,4.05233337578409));
#57384=CARTESIAN_POINT('Ctrl Pts',(-6.70620071746715,10.0211581030209,4.));
#57385=CARTESIAN_POINT('',(-8.29574161562937,10.0163810931058,4.00000000000001));
#57386=CARTESIAN_POINT('Origin',(-7.5,12.9903810567666,4.));
#57387=CARTESIAN_POINT('Ctrl Pts',(-10.5774088918681,12.99185618799,4.79157655282254));
#57388=CARTESIAN_POINT('Ctrl Pts',(-10.5779243576744,13.0789760377035,4.78704908248048));
#57389=CARTESIAN_POINT('Ctrl Pts',(-10.535392897551,14.1726059842126,4.73018823635432));
#57390=CARTESIAN_POINT('Ctrl Pts',(-9.2319528795399,16.1681374132995,4.62099401444409));
#57391=CARTESIAN_POINT('Ctrl Pts',(-5.80479653057489,16.1883357805992,4.46399388709183));
#57392=CARTESIAN_POINT('Ctrl Pts',(-3.89775210281319,13.3398493780975,4.30699375973959));
#57393=CARTESIAN_POINT('Ctrl Pts',(-5.2011833457958,10.227049143879,4.15232913070897));
#57394=CARTESIAN_POINT('Ctrl Pts',(-7.36594149062469,9.77083767708475,4.04999787746245));
#57395=CARTESIAN_POINT('Ctrl Pts',(-8.29574920379123,10.0163624306404,4.00000000000001));
#57396=CARTESIAN_POINT('Origin',(-7.5,12.9903810567666,14.2084234471775));
#57397=CARTESIAN_POINT('',(-10.5688836055535,12.9910731523796,5.79157655282255));
#57398=CARTESIAN_POINT('',(-10.5767201283484,12.9885005040359,5.70842344717746));
#57399=CARTESIAN_POINT('',(-10.5735,12.9903810567666,14.2084234471775));
#57400=CARTESIAN_POINT('Ctrl Pts',(-10.5767201283484,12.9885005040358,5.70842344717746));
#57401=CARTESIAN_POINT('Ctrl Pts',(-10.5702728094234,13.8768977505312,5.66228272262582));
#57402=CARTESIAN_POINT('Ctrl Pts',(-9.70223158388916,15.7839304785174,5.56380862229009));
#57403=CARTESIAN_POINT('Ctrl Pts',(-6.48106323809927,16.4631861795336,5.41300114617029));
#57404=CARTESIAN_POINT('Ctrl Pts',(-4.04127258839909,14.0562954080889,5.25600101881802));
#57405=CARTESIAN_POINT('Ctrl Pts',(-4.70303600953422,10.693474125437,5.09900089146578));
#57406=CARTESIAN_POINT('Ctrl Pts',(-7.87270732364685,9.390536089231,4.94200076411351));
#57407=CARTESIAN_POINT('Ctrl Pts',(-10.2242696810485,10.9865434678639,4.81180828268408));
#57408=CARTESIAN_POINT('Ctrl Pts',(-10.5690005839068,12.4954763477989,4.73394917703873));
#57409=CARTESIAN_POINT('Ctrl Pts',(-10.5686791348591,12.9902767031652,4.70842344717746));
#57410=CARTESIAN_POINT('Ctrl Pts',(-10.5688836055535,12.9910731523796,5.79157655282255));
#57411=CARTESIAN_POINT('Ctrl Pts',(-10.5698353122932,13.4534929538237,5.76771600385165));
#57412=CARTESIAN_POINT('Ctrl Pts',(-10.2562652325398,14.9289132187583,5.69152207909668));
#57413=CARTESIAN_POINT('Ctrl Pts',(-7.98558646537732,16.576874141135,5.56299477855761));
#57414=CARTESIAN_POINT('Ctrl Pts',(-4.77645105419042,15.3738768659897,5.40599465120536));
#57415=CARTESIAN_POINT('Ctrl Pts',(-4.00954823259222,12.0335573562934,5.24899452385311));
#57416=CARTESIAN_POINT('Ctrl Pts',(-6.37256675930357,9.55126737969704,5.09199439650085));
#57417=CARTESIAN_POINT('Ctrl Pts',(-9.64926869943611,10.135445743826,4.93952173949067));
#57418=CARTESIAN_POINT('Ctrl Pts',(-10.571966049015,12.0719510350338,4.83938245826456));
#57419=CARTESIAN_POINT('Ctrl Pts',(-10.5774088918681,12.99185618799,4.79157655282254));
#57420=CARTESIAN_POINT('Origin',(-7.5,12.9903810567666,14.2084234471775));
#57421=CARTESIAN_POINT('',(-10.5752286789639,12.9879604379016,6.79157655282255));
#57422=CARTESIAN_POINT('',(-10.5729905958558,12.9930261911251,6.70842344717746));
#57423=CARTESIAN_POINT('',(-10.5735,12.9903810567666,14.2084234471775));
#57424=CARTESIAN_POINT('Ctrl Pts',(-10.5729905958558,12.9930261911251,6.70842344717746));
#57425=CARTESIAN_POINT('Ctrl Pts',(-10.5751986555521,13.2468284658167,6.69528301978108));
#57426=CARTESIAN_POINT('Ctrl Pts',(-10.4312906141563,14.5089611116288,6.62980921660061));
#57427=CARTESIAN_POINT('Ctrl Pts',(-8.69550582596531,16.4064477577484,6.51200203763606));
#57428=CARTESIAN_POINT('Ctrl Pts',(-5.31022637025923,15.8719837317436,6.3550019102838));
#57429=CARTESIAN_POINT('Ctrl Pts',(-3.88853720662811,12.7535599895385,6.19800178293155));
#57430=CARTESIAN_POINT('Ctrl Pts',(-5.70528280371351,9.84749392134933,6.04100165557929));
#57431=CARTESIAN_POINT('Ctrl Pts',(-9.13136573648253,9.75968890749465,5.88400152822705));
#57432=CARTESIAN_POINT('Ctrl Pts',(-10.5176205520478,11.7432796147819,5.77314212542643));
#57433=CARTESIAN_POINT('Ctrl Pts',(-10.5775854376359,12.8692666957923,5.7146160984099));
#57434=CARTESIAN_POINT('Ctrl Pts',(-10.5767201283484,12.9885005040358,5.70842344717746));
#57435=CARTESIAN_POINT('Ctrl Pts',(-10.5752286789639,12.9879604379016,6.79157655282255));
#57436=CARTESIAN_POINT('Ctrl Pts',(-10.5680430414674,13.8206658595303,6.74838292522283));
#57437=CARTESIAN_POINT('Ctrl Pts',(-9.79183063316292,15.6740884921896,6.65285592183902));
#57438=CARTESIAN_POINT('Ctrl Pts',(-6.67544470099851,16.5144205342573,6.50499554267113));
#57439=CARTESIAN_POINT('Ctrl Pts',(-4.10581110106408,14.2466564935293,6.34799541531888));
#57440=CARTESIAN_POINT('Ctrl Pts',(-4.57977925134152,10.8523778836063,6.19099528796662));
#57441=CARTESIAN_POINT('Ctrl Pts',(-7.67233735803906,9.3752678814539,6.03399516061438));
#57442=CARTESIAN_POINT('Ctrl Pts',(-10.1638445777963,10.8716837770844,5.90085558223301));
#57443=CARTESIAN_POINT('Ctrl Pts',(-10.5677479325558,12.4392669496988,5.82004937963574));
#57444=CARTESIAN_POINT('Ctrl Pts',(-10.5688836055535,12.9910731523796,5.79157655282255));
#57445=CARTESIAN_POINT('Origin',(-7.5,12.9903810567666,14.2084234471775));
#57446=CARTESIAN_POINT('',(-10.5746464410021,12.992919470803,7.79157655282256));
#57447=CARTESIAN_POINT('',(-10.5698472063158,12.988625624027,7.70842344717746));
#57448=CARTESIAN_POINT('',(-10.5735,12.9903810567666,14.2084234471775));
#57449=CARTESIAN_POINT('Ctrl Pts',(-10.5698472063158,12.988625624027,7.70842344717746));
#57450=CARTESIAN_POINT('Ctrl Pts',(-10.5664960358364,13.6174691755491,7.67594994115225));
#57451=CARTESIAN_POINT('Ctrl Pts',(-10.0746935678837,15.2645519082853,7.59114305934296));
#57452=CARTESIAN_POINT('Ctrl Pts',(-7.39948646190492,16.6082039047423,7.45400280174958));
#57453=CARTESIAN_POINT('Ctrl Pts',(-4.42700258466931,14.902299453002,7.29700267439732));
#57454=CARTESIAN_POINT('Ctrl Pts',(-4.21010495775379,11.4819594519348,7.14000254704507));
#57455=CARTESIAN_POINT('Ctrl Pts',(-6.94328780249567,9.41423553851335,6.98300241969282));
#57456=CARTESIAN_POINT('Ctrl Pts',(-9.90513850811741,10.4579415361298,6.83914271973694));
#57457=CARTESIAN_POINT('Ctrl Pts',(-10.5664047849758,12.2360295461447,6.74761639556516));
#57458=CARTESIAN_POINT('Ctrl Pts',(-10.5729905958558,12.9930261911251,6.70842344717746));
#57459=CARTESIAN_POINT('Ctrl Pts',(-10.5746464410021,12.992919470803,7.79157655282255));
#57460=CARTESIAN_POINT('Ctrl Pts',(-10.5763833959288,13.1895272793482,7.78138322237809));
#57461=CARTESIAN_POINT('Ctrl Pts',(-10.4703645847954,14.393670666495,7.71885651614954));
#57462=CARTESIAN_POINT('Ctrl Pts',(-8.88333173423194,16.3348001890992,7.6039964341369));
#57463=CARTESIAN_POINT('Ctrl Pts',(-5.47359896850368,15.9891216041795,7.44699630678466));
#57464=CARTESIAN_POINT('Ctrl Pts',(-3.88095944817013,12.9544436048999,7.28999617943239));
#57465=CARTESIAN_POINT('Ctrl Pts',(-5.53354831017302,9.95199105749957,7.13299605208015));
#57466=CARTESIAN_POINT('Ctrl Pts',(-8.9494732676674,9.67409198306777,6.97599592472789));
#57467=CARTESIAN_POINT('Ctrl Pts',(-10.4834447329667,11.6282633493619,6.86218942497536));
#57468=CARTESIAN_POINT('Ctrl Pts',(-10.5767491559627,12.8117604221037,6.80071630100691));
#57469=CARTESIAN_POINT('Ctrl Pts',(-10.5752286789639,12.9879604379016,6.79157655282255));
#57470=CARTESIAN_POINT('Origin',(-7.5,12.9903810567666,14.2084234471775));
#57471=CARTESIAN_POINT('',(-10.5690545220509,12.9893859879631,8.79157655282255));
#57472=CARTESIAN_POINT('',(-10.5783066056774,12.9902007559877,8.70842344717746));
#57473=CARTESIAN_POINT('',(-10.5735,12.9903810567666,14.2084234471775));
#57474=CARTESIAN_POINT('Ctrl Pts',(-10.5783066056774,12.9902007559877,8.70842344717746));
#57475=CARTESIAN_POINT('Ctrl Pts',(-10.5774421776949,13.9863223355525,8.65661686252342));
#57476=CARTESIAN_POINT('Ctrl Pts',(-9.51496009867182,15.9902813747918,8.5524769020853));
#57477=CARTESIAN_POINT('Ctrl Pts',(-6.11666831357863,16.3348000735102,8.3960035658631));
#57478=CARTESIAN_POINT('Ctrl Pts',(-3.9473824601037,13.6815060275445,8.23900343851085));
#57479=CARTESIAN_POINT('Ctrl Pts',(-4.9637628366961,10.4084735910568,8.08200331115859));
#57480=CARTESIAN_POINT('Ctrl Pts',(-8.25441140963209,9.45066234771208,7.92500318380633));
#57481=CARTESIAN_POINT('Ctrl Pts',(-10.3278657153401,11.208539372,7.80047656247929));
#57482=CARTESIAN_POINT('Ctrl Pts',(-10.5718966865663,12.6040428499268,7.72828331693633));
#57483=CARTESIAN_POINT('Ctrl Pts',(-10.5698472063158,12.988625624027,7.70842344717746));
#57484=CARTESIAN_POINT('Ctrl Pts',(-10.5690545220509,12.9893859879631,8.79157655282255));
#57485=CARTESIAN_POINT('Ctrl Pts',(-10.5673548564085,13.5615306833804,8.76205014374926));
#57486=CARTESIAN_POINT('Ctrl Pts',(-10.1411931381796,15.1501114670399,8.6801903588919));
#57487=CARTESIAN_POINT('Ctrl Pts',(-7.60051354156566,16.6082040297755,8.54599719825042));
#57488=CARTESIAN_POINT('Ctrl Pts',(-4.53789809794217,15.0699719631857,8.38899707089818));
#57489=CARTESIAN_POINT('Ctrl Pts',(-4.1314278504052,11.6669507850401,8.23199694354592));
#57490=CARTESIAN_POINT('Ctrl Pts',(-6.74558856429446,9.45066222537301,8.07499681619367));
#57491=CARTESIAN_POINT('Ctrl Pts',(-9.82258984821385,10.3462870118539,7.92819001928587));
#57492=CARTESIAN_POINT('Ctrl Pts',(-10.5674657300694,12.1801270266301,7.83371659816217));
#57493=CARTESIAN_POINT('Ctrl Pts',(-10.5746464410021,12.992919470803,7.79157655282255));
#57494=CARTESIAN_POINT('Origin',(-7.5,12.9903810567666,14.2084234471775));
#57495=CARTESIAN_POINT('',(-10.5777630782332,12.9892372109846,9.79157655282255));
#57496=CARTESIAN_POINT('',(-10.5702336112086,12.9923647073181,9.70842344717745));
#57497=CARTESIAN_POINT('',(-10.5735,12.9903810567666,14.2084234471775));
#57498=CARTESIAN_POINT('Ctrl Pts',(-10.5702336112086,12.9923647073181,9.70842344717746));
#57499=CARTESIAN_POINT('Ctrl Pts',(-10.5724448600627,13.3564296204275,9.68961715967868));
#57500=CARTESIAN_POINT('Ctrl Pts',(-10.3454482739325,14.7309332712505,9.61847749639582));
#57501=CARTESIAN_POINT('Ctrl Pts',(-8.32455527051676,16.5144204123725,9.49500445732887));
#57502=CARTESIAN_POINT('Ctrl Pts',(-5.01553513899265,15.6221446466417,9.33800432997661));
#57503=CARTESIAN_POINT('Ctrl Pts',(-3.93435848267263,12.3699411347509,9.18100420262437));
#57504=CARTESIAN_POINT('Ctrl Pts',(-6.0505267824277,9.67409209769908,9.02400407527211));
#57505=CARTESIAN_POINT('Ctrl Pts',(-9.46645162186327,9.95199116250562,8.86700394791985));
#57506=CARTESIAN_POINT('Ctrl Pts',(-10.573722513556,11.9637004181345,8.76181040522164));
#57507=CARTESIAN_POINT('Ctrl Pts',(-10.5783153955445,12.9800717730395,8.70895023830751));
#57508=CARTESIAN_POINT('Ctrl Pts',(-10.5783066056774,12.9902007559877,8.70842344717746));
#57509=CARTESIAN_POINT('Ctrl Pts',(-10.5777630782332,12.9892372109846,9.79157655282255));
#57510=CARTESIAN_POINT('Ctrl Pts',(-10.5732100242337,13.9291375746327,9.74271706512043));
#57511=CARTESIAN_POINT('Ctrl Pts',(-9.61486878320428,15.8838097348119,9.64152420163422));
#57512=CARTESIAN_POINT('Ctrl Pts',(-6.30449413259093,16.4064478755407,9.48799796236394));
#57513=CARTESIAN_POINT('Ctrl Pts',(-3.99123576757957,13.8776914962184,9.3309978350117));
#57514=CARTESIAN_POINT('Ctrl Pts',(-4.82432014168349,10.5532756064786,9.17399770765943));
#57515=CARTESIAN_POINT('Ctrl Pts',(-8.05671221676616,9.41423541495656,9.0169975803072));
#57516=CARTESIAN_POINT('Ctrl Pts',(-10.2758759707643,11.0930905163184,8.88952386202821));
#57517=CARTESIAN_POINT('Ctrl Pts',(-10.5703673880222,12.5474465367502,8.81438351953334));
#57518=CARTESIAN_POINT('Ctrl Pts',(-10.5690545220509,12.9893859879631,8.79157655282255));
#57519=CARTESIAN_POINT('Origin',(-7.5,12.9903810567666,14.2084234471775));
#57520=CARTESIAN_POINT('',(-10.5715490487462,12.9928368154298,10.7915765528225));
#57521=CARTESIAN_POINT('',(-10.5724150045772,12.9877735244422,10.7084234471775));
#57522=CARTESIAN_POINT('',(-10.5735,12.9903810567666,14.2084234471775));
#57523=CARTESIAN_POINT('Ctrl Pts',(-10.5724150045772,12.9877735244422,10.7084234471775));
#57524=CARTESIAN_POINT('Ctrl Pts',(-10.5662071249442,13.7247736829249,10.6702840810499));
#57525=CARTESIAN_POINT('Ctrl Pts',(-9.93341852875246,15.4826369193415,10.5798113391382));
#57526=CARTESIAN_POINT('Ctrl Pts',(-7.01441355218445,16.5768740138536,10.4370052214424));
#57527=CARTESIAN_POINT('Ctrl Pts',(-4.24070833971001,14.56383815303,10.2800050940901));
#57528=CARTESIAN_POINT('Ctrl Pts',(-4.38964119697082,11.1398633340167,10.1230049667379));
#57529=CARTESIAN_POINT('Ctrl Pts',(-7.32766264781398,9.3752680069458,9.96600483938563));
#57530=CARTESIAN_POINT('Ctrl Pts',(-10.0497780511113,10.6754420854925,9.82781099953215));
#57531=CARTESIAN_POINT('Ctrl Pts',(-10.5662914862381,12.3433245134896,9.74195053546276));
#57532=CARTESIAN_POINT('Ctrl Pts',(-10.5702336112086,12.9923647073181,9.70842344717746));
#57533=CARTESIAN_POINT('Ctrl Pts',(-10.5715490487462,12.9928368154298,10.7915765528225));
#57534=CARTESIAN_POINT('Ctrl Pts',(-10.5739357845658,13.2995215285911,10.7757173622757));
#57535=CARTESIAN_POINT('Ctrl Pts',(-10.391916652594,14.6154630132259,10.7075247959447));
#57536=CARTESIAN_POINT('Ctrl Pts',(-8.5189368031419,16.4631863186891,10.5869988538297));
#57537=CARTESIAN_POINT('Ctrl Pts',(-5.16549655959477,15.7560380892136,10.4299987264775));
#57538=CARTESIAN_POINT('Ctrl Pts',(-3.90540705298465,12.5688686867556,10.2729985991252));
#57539=CARTESIAN_POINT('Ctrl Pts',(-5.86863420589283,9.75968879265402,10.115998471773));
#57540=CARTESIAN_POINT('Ctrl Pts',(-9.29471725902464,9.84749381445728,9.9589983444207));
#57541=CARTESIAN_POINT('Ctrl Pts',(-10.5460795409153,11.8491727898316,9.85085770477057));
#57542=CARTESIAN_POINT('Ctrl Pts',(-10.5780867983696,12.9224107085984,9.79505044090452));
#57543=CARTESIAN_POINT('Ctrl Pts',(-10.5777630782332,12.9892372109846,9.79157655282255));
#57544=CARTESIAN_POINT('Origin',(-7.5,12.9903810567666,14.2084234471775));
#57545=CARTESIAN_POINT('',(-10.5702206634037,12.9870745539208,11.7915765528226));
#57546=CARTESIAN_POINT('',(-10.5771718362758,12.9919049495641,11.7084234471775));
#57547=CARTESIAN_POINT('',(-10.5735,12.9903810567666,14.2084234471775));
#57548=CARTESIAN_POINT('',(-8.29379928253292,10.0211581030209,12.));
#57549=CARTESIAN_POINT('Ctrl Pts',(-8.29379928253292,10.0211581030209,12.));
#57550=CARTESIAN_POINT('Ctrl Pts',(-9.27014005842312,10.2821754194981,11.9476666242159));
#57551=CARTESIAN_POINT('Ctrl Pts',(-10.3714991025232,11.3144735509882,11.8781921418234));
#57552=CARTESIAN_POINT('Ctrl Pts',(-10.5724953140326,12.655363779409,11.808717659431));
#57553=CARTESIAN_POINT('Ctrl Pts',(-10.5702206634037,12.9870745539208,11.7915765528226));
#57554=CARTESIAN_POINT('',(-6.70425858890745,10.0163809826708,12.));
#57555=CARTESIAN_POINT('Origin',(-7.5,12.9903810567666,12.));
#57556=CARTESIAN_POINT('Ctrl Pts',(-6.70425100699972,10.0163623331919,12.));
#57557=CARTESIAN_POINT('Ctrl Pts',(-7.63405880919358,9.77083750064795,11.9500021225376));
#57558=CARTESIAN_POINT('Ctrl Pts',(-9.69010226711413,10.2041387247117,11.8528099382634));
#57559=CARTESIAN_POINT('Ctrl Pts',(-10.5713066024909,12.0837656721183,11.7556177539892));
#57560=CARTESIAN_POINT('Ctrl Pts',(-10.5771718362758,12.9919049495641,11.7084234471775));
#57561=CARTESIAN_POINT('Origin',(-7.50000000000001,-12.9903810567666,7.5));
#57562=CARTESIAN_POINT('',(-10.0135514395051,-12.9904666377399,4.38741669750803));
#57563=CARTESIAN_POINT('',(-10.0159862278212,-12.9935669321582,4.11258330249198));
#57564=CARTESIAN_POINT('',(-10.0175,-12.9903810567666,7.5));
#57565=CARTESIAN_POINT('',(-9.41346599666503,-11.3543938533916,4.));
#57566=CARTESIAN_POINT('Ctrl Pts',(-10.0159862278212,-12.9935669321582,
4.11258330249198));
#57567=CARTESIAN_POINT('Ctrl Pts',(-10.0108023762528,-12.4010697429433,
4.07505553499466));
#57568=CARTESIAN_POINT('Ctrl Pts',(-9.79922182808404,-11.8055774964621,
4.03752776749733));
#57569=CARTESIAN_POINT('Ctrl Pts',(-9.41346599666503,-11.3543938533916,
4.));
#57570=CARTESIAN_POINT('',(-10.0175,-12.9903810567666,4.));
#57571=CARTESIAN_POINT('Origin',(-7.50000000000001,-12.9903810567666,4.));
#57572=CARTESIAN_POINT('',(-10.0175,-12.9903810567666,3.));
#57573=CARTESIAN_POINT('',(-10.0175,-12.9903810567666,7.5));
#57574=CARTESIAN_POINT('Origin',(-7.50000000000001,-12.9903810567666,3.));
#57575=CARTESIAN_POINT('',(-5.58300636833058,-11.3520706988407,4.));
#57576=CARTESIAN_POINT('Origin',(-7.50000000000001,-12.9903810567666,4.));
#57577=CARTESIAN_POINT('Ctrl Pts',(-5.58299257280548,-11.3520616136783,
4.));
#57578=CARTESIAN_POINT('Ctrl Pts',(-6.09671565847252,-10.7549231085896,
4.04999787746244));
#57579=CARTESIAN_POINT('Ctrl Pts',(-6.91408826359173,-10.4146529403296,
4.09999575492489));
#57580=CARTESIAN_POINT('Ctrl Pts',(-7.6991792943871,-10.4769907523554,4.14999363238733));
#57581=CARTESIAN_POINT('Ctrl Pts',(-8.52094345767964,-10.5422404851016,
4.20232700817142));
#57582=CARTESIAN_POINT('Ctrl Pts',(-9.30733973752043,-11.0485898984475,
4.2546603839555));
#57583=CARTESIAN_POINT('Ctrl Pts',(-9.70625816906456,-11.7696982113955,
4.30699375973958));
#57584=CARTESIAN_POINT('Ctrl Pts',(-9.91060317652291,-12.1390842109776,
4.3338014056624));
#57585=CARTESIAN_POINT('Ctrl Pts',(-10.0132749267868,-12.5648224302545,
4.36060905158521));
#57586=CARTESIAN_POINT('Ctrl Pts',(-10.0135514395051,-12.9904666377399,
4.38741669750803));
#57587=CARTESIAN_POINT('Origin',(-7.50000000000001,-12.9903810567666,7.5));
#57588=CARTESIAN_POINT('',(-10.0201378128903,-12.991921413328,5.38741669750803));
#57589=CARTESIAN_POINT('',(-10.020701946345,-12.9891728119784,5.11258330249198));
#57590=CARTESIAN_POINT('',(-10.0175,-12.9903810567666,7.5));
#57591=CARTESIAN_POINT('Ctrl Pts',(-10.020701946345,-12.9891728119784,5.11258330249198));
#57592=CARTESIAN_POINT('Ctrl Pts',(-10.0211241641948,-12.9178130461518,
5.10805583214991));
#57593=CARTESIAN_POINT('Ctrl Pts',(-10.0183502770585,-12.846486861832,5.10352836180784));
#57594=CARTESIAN_POINT('Ctrl Pts',(-10.0122725294143,-12.775443667658,5.09900089146577));
#57595=CARTESIAN_POINT('Ctrl Pts',(-9.94201937978509,-11.9542499553417,
5.04666751568169));
#57596=CARTESIAN_POINT('Ctrl Pts',(-9.43032999980707,-11.170867192649,4.99433413989761));
#57597=CARTESIAN_POINT('Ctrl Pts',(-8.70662199025935,-10.7764184817432,
4.94200076411352));
#57598=CARTESIAN_POINT('Ctrl Pts',(-7.98291398071162,-10.3819697708373,
4.88966738832944));
#57599=CARTESIAN_POINT('Ctrl Pts',(-7.04718734159418,-10.3764551117184,
4.83733401254535));
#57600=CARTESIAN_POINT('Ctrl Pts',(-6.31898112841336,-10.7625629528365,
4.78500063676127));
#57601=CARTESIAN_POINT('Ctrl Pts',(-5.59077491523255,-11.1486707939545,
4.73266726097718));
#57602=CARTESIAN_POINT('Ctrl Pts',(-5.07008912798835,-11.9264011353096,
4.6803338851931));
#57603=CARTESIAN_POINT('Ctrl Pts',(-4.99037287718051,-12.7466319075856,
4.62800050940901));
#57604=CARTESIAN_POINT('Ctrl Pts',(-4.91065662637267,-13.5668626798615,
4.57566713362493));
#57605=CARTESIAN_POINT('Ctrl Pts',(-5.27190991200121,-14.4295938830583,
4.52333375784085));
#57606=CARTESIAN_POINT('Ctrl Pts',(-5.9121672709983,-14.948847615037,4.47100038205676));
#57607=CARTESIAN_POINT('Ctrl Pts',(-6.55242462999539,-15.4681013470158,
4.41866700627267));
#57608=CARTESIAN_POINT('Ctrl Pts',(-7.47168606236103,-15.6438776077765,
4.36633363048859));
#57609=CARTESIAN_POINT('Ctrl Pts',(-8.25780335304795,-15.3956944886946,
4.31400025470451));
#57610=CARTESIAN_POINT('Ctrl Pts',(-9.04392064373486,-15.1475113696128,
4.26166687892042));
#57611=CARTESIAN_POINT('Ctrl Pts',(-9.69689379274305,-14.4753688706883,
4.20933350313634));
#57612=CARTESIAN_POINT('Ctrl Pts',(-9.92376658082896,-13.6843861063472,
4.15700012735226));
#57613=CARTESIAN_POINT('Ctrl Pts',(-9.98795104401328,-13.460609581425,4.1421945190655));
#57614=CARTESIAN_POINT('Ctrl Pts',(-10.0180313821391,-13.2273213460105,
4.12738891077874));
#57615=CARTESIAN_POINT('Ctrl Pts',(-10.0159862278212,-12.9935669321582,
4.11258330249198));
#57616=CARTESIAN_POINT('Ctrl Pts',(-10.0135514395051,-12.9904666377399,
4.38741669750803));
#57617=CARTESIAN_POINT('Ctrl Pts',(-10.013814729649,-13.3957569451608,4.41294242736929));
#57618=CARTESIAN_POINT('Ctrl Pts',(-9.92124152424158,-13.8009620169255,
4.43846815723057));
#57619=CARTESIAN_POINT('Ctrl Pts',(-9.73520854233975,-14.1573521883653,
4.46399388709184));
#57620=CARTESIAN_POINT('Ctrl Pts',(-9.35379990082332,-14.8880306398367,
4.51632726287592));
#57621=CARTESIAN_POINT('Ctrl Pts',(-8.57954203454297,-15.4135203302294,
4.56866063866001));
#57622=CARTESIAN_POINT('Ctrl Pts',(-7.75970075309617,-15.4983926191754,
4.62099401444409));
#57623=CARTESIAN_POINT('Ctrl Pts',(-6.93985947164937,-15.5832649081213,
4.67332739022818));
#57624=CARTESIAN_POINT('Ctrl Pts',(-6.07443477503611,-15.2275197956205,
4.72566076601226));
#57625=CARTESIAN_POINT('Ctrl Pts',(-5.5513808289996,-14.5905667824841,4.77799414179634));
#57626=CARTESIAN_POINT('Ctrl Pts',(-5.02832688296309,-13.9536137693476,
4.83032751758043));
#57627=CARTESIAN_POINT('Ctrl Pts',(-4.84764368750334,-13.0354528555755,
4.88266089336451));
#57628=CARTESIAN_POINT('Ctrl Pts',(-5.09037368993613,-12.2477921509444,
4.93499426914859));
#57629=CARTESIAN_POINT('Ctrl Pts',(-5.33310369236891,-11.4601314463133,
4.98732764493268));
#57630=CARTESIAN_POINT('Ctrl Pts',(-5.99924689269421,-10.8029709508232,
5.03966102071677));
#57631=CARTESIAN_POINT('Ctrl Pts',(-6.79011830096555,-10.5709280850384,
5.09199439650085));
#57632=CARTESIAN_POINT('Ctrl Pts',(-7.58098970923688,-10.3388852192536,
5.14432777228494));
#57633=CARTESIAN_POINT('Ctrl Pts',(-8.49658932545427,-10.5319599831741,
5.19666114806902));
#57634=CARTESIAN_POINT('Ctrl Pts',(-9.1264120969476,-11.0635984608226,5.2489945238531));
#57635=CARTESIAN_POINT('Ctrl Pts',(-9.68170742388623,-11.532327721848,5.29513524840475));
#57636=CARTESIAN_POINT('Ctrl Pts',(-10.0148568228205,-12.2642362843572,
5.34127597295639));
#57637=CARTESIAN_POINT('Ctrl Pts',(-10.0201378128903,-12.991921413328,5.38741669750803));
#57638=CARTESIAN_POINT('Origin',(-7.50000000000001,-12.9903810567666,7.5));
#57639=CARTESIAN_POINT('',(-10.0170829580245,-12.9882144302548,6.38741669750803));
#57640=CARTESIAN_POINT('',(-10.0137189064297,-12.9898141627747,6.11258330249198));
#57641=CARTESIAN_POINT('',(-10.0175,-12.9903810567666,7.5));
#57642=CARTESIAN_POINT('Ctrl Pts',(-10.0137189064297,-12.9898141627747,
6.11258330249198));
#57643=CARTESIAN_POINT('Ctrl Pts',(-10.0144984482212,-12.6110466544282,
6.08872275352109));
#57644=CARTESIAN_POINT('Ctrl Pts',(-9.93406605373638,-12.2325935036327,
6.06486220455019));
#57645=CARTESIAN_POINT('Ctrl Pts',(-9.77069376862533,-11.8941805898436,
6.04100165557929));
#57646=CARTESIAN_POINT('Ctrl Pts',(-9.41236910476912,-11.151939067693,5.98866827979521));
#57647=CARTESIAN_POINT('Ctrl Pts',(-8.65505620083081,-10.6023139521363,
5.93633490401113));
#57648=CARTESIAN_POINT('Ctrl Pts',(-7.83829991591844,-10.4917303363644,
5.88400152822705));
#57649=CARTESIAN_POINT('Ctrl Pts',(-7.02154363100607,-10.3811467205925,
5.83166815244296));
#57650=CARTESIAN_POINT('Ctrl Pts',(-6.14534396511963,-10.7096046046056,
5.77933477665887));
#57651=CARTESIAN_POINT('Ctrl Pts',(-5.60254926887142,-11.3298421637022,
5.72700140087479));
#57652=CARTESIAN_POINT('Ctrl Pts',(-5.05975457262321,-11.9500797227988,
5.6746680250907));
#57653=CARTESIAN_POINT('Ctrl Pts',(-4.8503648460132,-12.862096956979,5.62233464930662));
#57654=CARTESIAN_POINT('Ctrl Pts',(-5.06826092360056,-13.6569790435728,
5.57000127352254));
#57655=CARTESIAN_POINT('Ctrl Pts',(-5.28615700118792,-14.4518611301666,
5.51766789773845));
#57656=CARTESIAN_POINT('Ctrl Pts',(-5.93133888297262,-15.129608069174,5.46533452195437));
#57657=CARTESIAN_POINT('Ctrl Pts',(-6.71453628267279,-15.3863634879565,
5.41300114617028));
#57658=CARTESIAN_POINT('Ctrl Pts',(-7.49773368237297,-15.6431189067389,
5.3606677703862));
#57659=CARTESIAN_POINT('Ctrl Pts',(-8.41894659998862,-15.4788828052965,
5.30833439460211));
#57660=CARTESIAN_POINT('Ctrl Pts',(-9.06514459915626,-14.9672624236053,
5.25600101881803));
#57661=CARTESIAN_POINT('Ctrl Pts',(-9.65543865112952,-14.4999033965431,
5.20819511337601));
#57662=CARTESIAN_POINT('Ctrl Pts',(-10.0162437157927,-13.7426660344013,
5.160389207934));
#57663=CARTESIAN_POINT('Ctrl Pts',(-10.020701946345,-12.9891728119784,5.11258330249198));
#57664=CARTESIAN_POINT('Ctrl Pts',(-10.0201378128903,-12.991921413328,5.38741669750803));
#57665=CARTESIAN_POINT('Ctrl Pts',(-10.0208465865384,-13.0895856839813,
5.39360934874047));
#57666=CARTESIAN_POINT('Ctrl Pts',(-10.0156494886519,-13.1871738782112,
5.39980199997292));
#57667=CARTESIAN_POINT('Ctrl Pts',(-10.004290929159,-13.2840395347951,5.40599465120536));
#57668=CARTESIAN_POINT('Ctrl Pts',(-9.90830106310784,-14.1026399397423,
5.45832802698944));
#57669=CARTESIAN_POINT('Ctrl Pts',(-9.37227540423617,-14.8696385582602,
5.51066140277353));
#57670=CARTESIAN_POINT('Ctrl Pts',(-8.63654582863995,-15.2411510354214,
5.56299477855761));
#57671=CARTESIAN_POINT('Ctrl Pts',(-7.90081625304375,-15.6126635125827,
5.61532815434169));
#57672=CARTESIAN_POINT('Ctrl Pts',(-6.96538276072302,-15.5886898483873,
5.66766153012578));
#57673=CARTESIAN_POINT('Ctrl Pts',(-6.24965032039424,-15.1799771379828,
5.71999490590986));
#57674=CARTESIAN_POINT('Ctrl Pts',(-5.53391788006544,-14.7712644275784,
5.77232828169395));
#57675=CARTESIAN_POINT('Ctrl Pts',(-5.03788649172861,-13.9778126709648,
5.82466165747803));
#57676=CARTESIAN_POINT('Ctrl Pts',(-4.9839547824182,-13.1553705931073,5.87699503326212));
#57677=CARTESIAN_POINT('Ctrl Pts',(-4.9300230731078,-12.3329285152499,5.9293284090462));
#57678=CARTESIAN_POINT('Ctrl Pts',(-5.31819104282381,-11.4814961161485,
5.98166178483029));
#57679=CARTESIAN_POINT('Ctrl Pts',(-5.97442142669028,-10.9828167750565,
6.03399516061437));
#57680=CARTESIAN_POINT('Ctrl Pts',(-6.63065181055676,-10.4841374339645,
6.08632853639846));
#57681=CARTESIAN_POINT('Ctrl Pts',(-7.5549446085737,-10.338211150882,6.13866191218254));
#57682=CARTESIAN_POINT('Ctrl Pts',(-8.33288886120492,-10.6104648899579,
6.19099528796662));
#57683=CARTESIAN_POINT('Ctrl Pts',(-9.11083311383614,-10.8827186290339,
6.24332866375071));
#57684=CARTESIAN_POINT('Ctrl Pts',(-9.74242882108165,-11.5731523902683,
6.29566203953479));
#57685=CARTESIAN_POINT('Ctrl Pts',(-9.94449694127237,-12.3722067750024,
6.34799541531888));
#57686=CARTESIAN_POINT('Ctrl Pts',(-9.9952343802911,-12.5728419522874,6.36113584271526));
#57687=CARTESIAN_POINT('Ctrl Pts',(-10.0188915771041,-12.7803252875989,
6.37427627011165));
#57688=CARTESIAN_POINT('Ctrl Pts',(-10.0170829580245,-12.9882144302548,
6.38741669750803));
#57689=CARTESIAN_POINT('Origin',(-7.50000000000001,-12.9903810567666,7.5));
#57690=CARTESIAN_POINT('',(-10.0145082114167,-12.9918189296441,7.38741669750803));
#57691=CARTESIAN_POINT('',(-10.018916148665,-12.992363782792,7.11258330249199));
#57692=CARTESIAN_POINT('',(-10.0175,-12.9903810567666,7.5));
#57693=CARTESIAN_POINT('Ctrl Pts',(-10.018916148665,-12.992363782792,7.11258330249199));
#57694=CARTESIAN_POINT('Ctrl Pts',(-10.0130304015467,-12.3102957636159,
7.06938967489226));
#57695=CARTESIAN_POINT('Ctrl Pts',(-9.72554857159998,-11.6238530781169,
7.02619604729253));
#57696=CARTESIAN_POINT('Ctrl Pts',(-9.23088494583046,-11.1568755721922,
6.98300241969281));
#57697=CARTESIAN_POINT('Ctrl Pts',(-8.63155076501069,-10.5910858791674,
6.93066904390873));
#57698=CARTESIAN_POINT('Ctrl Pts',(-7.72807925079087,-10.3474651982644,
6.87833566812465));
#57699=CARTESIAN_POINT('Ctrl Pts',(-6.92554619007859,-10.5352419954014,
6.82600229234057));
#57700=CARTESIAN_POINT('Ctrl Pts',(-6.12301312936631,-10.7230187925383,
6.77366891655648));
#57701=CARTESIAN_POINT('Ctrl Pts',(-5.42141852216156,-11.342193067715,6.72133554077239));
#57702=CARTESIAN_POINT('Ctrl Pts',(-5.13532567649039,-12.1151551330277,
6.6690021649883));
#57703=CARTESIAN_POINT('Ctrl Pts',(-4.84923283081922,-12.8881171983403,
6.61666878920422));
#57704=CARTESIAN_POINT('Ctrl Pts',(-4.97864174668163,-13.8148670537889,
6.56433541342015));
#57705=CARTESIAN_POINT('Ctrl Pts',(-5.46553131494727,-14.4798918223762,
6.51200203763606));
#57706=CARTESIAN_POINT('Ctrl Pts',(-5.95242088321289,-15.1449165909636,
6.45966866185198));
#57707=CARTESIAN_POINT('Ctrl Pts',(-6.79679110388174,-15.5482162726898,
6.40733528606788));
#57708=CARTESIAN_POINT('Ctrl Pts',(-7.62006454012935,-15.5089697827308,
6.3550019102838));
#57709=CARTESIAN_POINT('Ctrl Pts',(-8.44333797637697,-15.4697232927718,
6.30266853449971));
#57710=CARTESIAN_POINT('Ctrl Pts',(-9.24551462820336,-14.9879306311276,
6.25033515871564));
#57711=CARTESIAN_POINT('Ctrl Pts',(-9.6669347422295,-14.2796053359332,6.19800178293155));
#57712=CARTESIAN_POINT('Ctrl Pts',(-9.89621522991991,-13.8942294041248,
6.16952895611836));
#57713=CARTESIAN_POINT('Ctrl Pts',(-10.012788678108,-13.4417979658618,6.14105612930517));
#57714=CARTESIAN_POINT('Ctrl Pts',(-10.0137189064297,-12.9898141627747,
6.11258330249198));
#57715=CARTESIAN_POINT('Ctrl Pts',(-10.0170829580245,-12.9882144302548,
6.38741669750803));
#57716=CARTESIAN_POINT('Ctrl Pts',(-10.0116885281401,-13.6082694857485,
6.42660964589573));
#57717=CARTESIAN_POINT('Ctrl Pts',(-9.77974909684708,-14.2319346209584,
6.46580259428343));
#57718=CARTESIAN_POINT('Ctrl Pts',(-9.36410112291705,-14.688271412029,6.50499554267113));
#57719=CARTESIAN_POINT('Ctrl Pts',(-8.80909665123509,-15.2976066560878,
6.55732891845521));
#57720=CARTESIAN_POINT('Ctrl Pts',(-7.92654717473526,-15.6086021359717,
6.6096622942393));
#57721=CARTESIAN_POINT('Ctrl Pts',(-7.11214796457486,-15.4818215077834,
6.66199567002339));
#57722=CARTESIAN_POINT('Ctrl Pts',(-6.29774875441446,-15.3550408795951,
6.71432904580747));
#57723=CARTESIAN_POINT('Ctrl Pts',(-5.55149981059349,-14.7904841433347,
6.76666242159156));
#57724=CARTESIAN_POINT('Ctrl Pts',(-5.20798543690379,-14.041273034435,6.81899579737564));
#57725=CARTESIAN_POINT('Ctrl Pts',(-4.8644710632141,-13.2920619255352,6.87132917315972));
#57726=CARTESIAN_POINT('Ctrl Pts',(-4.92369125965567,-12.3581964439962,
6.92366254894381));
#57727=CARTESIAN_POINT('Ctrl Pts',(-5.35909436185687,-11.6583796505146,
6.97599592472789));
#57728=CARTESIAN_POINT('Ctrl Pts',(-5.79449746405807,-10.958562857033,7.02832930051198));
#57729=CARTESIAN_POINT('Ctrl Pts',(-6.60608347201889,-10.4927947516089,
7.08066267629606));
#57730=CARTESIAN_POINT('Ctrl Pts',(-7.42997390874126,-10.469904702335,7.13299605208014));
#57731=CARTESIAN_POINT('Ctrl Pts',(-8.25386434546363,-10.4470146530611,
7.18532942786423));
#57732=CARTESIAN_POINT('Ctrl Pts',(-9.09005921094755,-10.8670026599375,
7.23766280364831));
#57733=CARTESIAN_POINT('Ctrl Pts',(-9.56364652484227,-11.5415650835207,
7.2899961794324));
#57734=CARTESIAN_POINT('Ctrl Pts',(-9.8575133022249,-11.9601393986381,7.32246968545761));
#57735=CARTESIAN_POINT('Ctrl Pts',(-10.0117632716449,-12.4767339212603,
7.35494319148282));
#57736=CARTESIAN_POINT('Ctrl Pts',(-10.0145082114167,-12.9918189296441,
7.38741669750803));
#57737=CARTESIAN_POINT('Origin',(-7.50000000000001,-12.9903810567666,7.5));
#57738=CARTESIAN_POINT('',(-10.0214372954169,-12.9905287409231,8.38741669750803));
#57739=CARTESIAN_POINT('',(-10.0184392382435,-12.988301844852,8.11258330249199));
#57740=CARTESIAN_POINT('',(-10.0175,-12.9903810567666,7.5));
#57741=CARTESIAN_POINT('Ctrl Pts',(-10.0184392382435,-12.988301844852,8.11258330249199));
#57742=CARTESIAN_POINT('Ctrl Pts',(-10.0198619759554,-12.8272606230119,
8.10238997204752));
#57743=CARTESIAN_POINT('Ctrl Pts',(-10.0057050234181,-12.6664683956915,
8.09219664160306));
#57744=CARTESIAN_POINT('Ctrl Pts',(-9.97504897913497,-12.5088858958898,
8.08200331115859));
#57745=CARTESIAN_POINT('Ctrl Pts',(-9.81765838984107,-11.699844707237,8.02966993537451));
#57746=CARTESIAN_POINT('Ctrl Pts',(-9.22537188297354,-10.9754080177822,
7.97733655959042));
#57747=CARTESIAN_POINT('Ctrl Pts',(-8.46374395491092,-10.660380492594,7.92500318380633));
#57748=CARTESIAN_POINT('Ctrl Pts',(-7.70211602684831,-10.3453529674058,
7.87266980802225));
#57749=CARTESIAN_POINT('Ctrl Pts',(-6.77114667759061,-10.4397346064841,
7.82033643223817));
#57750=CARTESIAN_POINT('Ctrl Pts',(-6.0882404805551,-10.9012089485628,7.76800305645409));
#57751=CARTESIAN_POINT('Ctrl Pts',(-5.4053342835196,-11.3626832906415,7.71566968067));
#57752=CARTESIAN_POINT('Ctrl Pts',(-4.97049123870628,-12.1912503357206,
7.66333630488591));
#57753=CARTESIAN_POINT('Ctrl Pts',(-4.97867531110115,-13.0154180759185,
7.61100292910183));
#57754=CARTESIAN_POINT('Ctrl Pts',(-4.98685938349602,-13.8395858161164,
7.55866955331774));
#57755=CARTESIAN_POINT('Ctrl Pts',(-5.43807057309907,-14.6593542514331,
7.50633617753366));
#57756=CARTESIAN_POINT('Ctrl Pts',(-6.130006178679,-15.1071762692505,7.45400280174958));
#57757=CARTESIAN_POINT('Ctrl Pts',(-6.82194178425893,-15.554998287068,7.40166942596549));
#57758=CARTESIAN_POINT('Ctrl Pts',(-7.75460180581574,-15.6308738873863,
7.3493360501814));
#57759=CARTESIAN_POINT('Ctrl Pts',(-8.509823648947,-15.3007838855131,7.29700267439732));
#57760=CARTESIAN_POINT('Ctrl Pts',(-9.26504549207826,-14.9706938836398,
7.24466929861323));
#57761=CARTESIAN_POINT('Ctrl Pts',(-9.84282915678396,-14.2346382795751,
7.19233592282916));
#57762=CARTESIAN_POINT('Ctrl Pts',(-9.98412256542695,-13.4226311249693,
7.14000254704507));
#57763=CARTESIAN_POINT('Ctrl Pts',(-10.0087987143617,-13.2808183562381,
7.13086279886071));
#57764=CARTESIAN_POINT('Ctrl Pts',(-10.0201615695645,-13.1366890058931,
7.12172305067635));
#57765=CARTESIAN_POINT('Ctrl Pts',(-10.018916148665,-12.992363782792,7.11258330249199));
#57766=CARTESIAN_POINT('Ctrl Pts',(-10.0145082114167,-12.9918189296441,
7.38741669750803));
#57767=CARTESIAN_POINT('Ctrl Pts',(-10.0161869382632,-13.306830224492,7.4072765672669));
#57768=CARTESIAN_POINT('Ctrl Pts',(-9.96119980531574,-13.6212769313365,
7.42713643702578));
#57769=CARTESIAN_POINT('Ctrl Pts',(-9.84682750368121,-13.9123926462011,
7.44699630678465));
#57770=CARTESIAN_POINT('Ctrl Pts',(-9.54544140631991,-14.6795209450086,
7.49932968256874));
#57771=CARTESIAN_POINT('Ctrl Pts',(-8.83168944929182,-15.2846407023335,
7.55166305835282));
#57772=CARTESIAN_POINT('Ctrl Pts',(-8.02558574588715,-15.4564435717975,
7.60399643413691));
#57773=CARTESIAN_POINT('Ctrl Pts',(-7.21948204248248,-15.6282464412614,
7.65632980992099));
#57774=CARTESIAN_POINT('Ctrl Pts',(-6.32102659270125,-15.3667324228643,
7.70866318570508));
#57775=CARTESIAN_POINT('Ctrl Pts',(-5.73304620733022,-14.789152581525,7.76099656148916));
#57776=CARTESIAN_POINT('Ctrl Pts',(-5.1450658219592,-14.2115727401857,7.81332993727324));
#57777=CARTESIAN_POINT('Ctrl Pts',(-4.86756050099838,-13.3179270759042,
7.86566331305732));
#57778=CARTESIAN_POINT('Ctrl Pts',(-5.02495108614128,-12.5088859085888,
7.91799668884141));
#57779=CARTESIAN_POINT('Ctrl Pts',(-5.18234167128417,-11.6998447412735,
7.9703300646255));
#57780=CARTESIAN_POINT('Ctrl Pts',(-5.77462816253079,-10.9754080709243,
8.02266344040959));
#57781=CARTESIAN_POINT('Ctrl Pts',(-6.53625607050644,-10.6603805540446,
8.07499681619367));
#57782=CARTESIAN_POINT('Ctrl Pts',(-7.29788397848209,-10.3453530371649,
8.12733019197775));
#57783=CARTESIAN_POINT('Ctrl Pts',(-8.22885330318678,-10.4397346737546,
8.17966356776183));
#57784=CARTESIAN_POINT('Ctrl Pts',(-8.91175948221152,-10.9012090036623,
8.23199694354592));
#57785=CARTESIAN_POINT('Ctrl Pts',(-9.5877914836703,-11.3580381032537,8.28380352819995));
#57786=CARTESIAN_POINT('Ctrl Pts',(-10.0207292434803,-12.1746067346983,
8.33561011285399));
#57787=CARTESIAN_POINT('Ctrl Pts',(-10.0214372954169,-12.9905287409231,
8.38741669750803));
#57788=CARTESIAN_POINT('Origin',(-7.50000000000001,-12.9903810567666,7.5));
#57789=CARTESIAN_POINT('',(-10.014824715197,-12.9887562509003,9.38741669750802));
#57790=CARTESIAN_POINT('',(-10.0138589040853,-12.9911961164478,9.11258330249198));
#57791=CARTESIAN_POINT('',(-10.0175,-12.9903810567666,7.5));
#57792=CARTESIAN_POINT('Ctrl Pts',(-10.0138589040853,-12.9911961164478,
9.11258330249198));
#57793=CARTESIAN_POINT('Ctrl Pts',(-10.0124667099841,-12.5225530777913,
9.08305689341869));
#57794=CARTESIAN_POINT('Ctrl Pts',(-9.88655945291767,-12.0532151702485,
9.05353048434541));
#57795=CARTESIAN_POINT('Ctrl Pts',(-9.64090569460772,-11.6583796153827,
9.02400407527212));
#57796=CARTESIAN_POINT('Ctrl Pts',(-9.20550258092411,-10.9585628034427,
8.97167069948803));
#57797=CARTESIAN_POINT('Ctrl Pts',(-8.39391655155678,-10.4927946857384,
8.91933732370393));
#57798=CARTESIAN_POINT('Ctrl Pts',(-7.57002609310491,-10.4699046358618,
8.86700394791985));
#57799=CARTESIAN_POINT('Ctrl Pts',(-6.74613563465304,-10.4470145859851,
8.81467057213576));
#57800=CARTESIAN_POINT('Ctrl Pts',(-5.90994074711664,-10.8670026039362,
8.7623371963517));
#57801=CARTESIAN_POINT('Ctrl Pts',(-5.43635342073195,-11.5415650453096,
8.71000382056761));
#57802=CARTESIAN_POINT('Ctrl Pts',(-4.96276609434725,-12.216127486683,8.65767044478353));
#57803=CARTESIAN_POINT('Ctrl Pts',(-4.85178632911427,-13.1452643514787,
8.60533706899943));
#57804=CARTESIAN_POINT('Ctrl Pts',(-5.15317243442415,-13.9123926705184,
8.55300369321534));
#57805=CARTESIAN_POINT('Ctrl Pts',(-5.45455853973402,-14.6795209895581,
8.50067031743125));
#57806=CARTESIAN_POINT('Ctrl Pts',(-6.16831051558674,-15.2846407628417,
8.44833694164718));
#57807=CARTESIAN_POINT('Ctrl Pts',(-6.97441424025143,-15.4564436368365,
8.3960035658631));
#57808=CARTESIAN_POINT('Ctrl Pts',(-7.78051796491612,-15.6282465108314,
8.34367019007902));
#57809=CARTESIAN_POINT('Ctrl Pts',(-8.67897343839277,-15.3667324855376,
8.29133681429492));
#57810=CARTESIAN_POINT('Ctrl Pts',(-9.26695383927095,-14.7891526289653,
8.23900343851084));
#57811=CARTESIAN_POINT('Ctrl Pts',(-9.74040926576667,-14.324071961446,8.19686339317122));
#57812=CARTESIAN_POINT('Ctrl Pts',(-10.0125575264699,-13.6540591679237,
8.15472334783161));
#57813=CARTESIAN_POINT('Ctrl Pts',(-10.0184392382435,-12.988301844852,8.11258330249199));
#57814=CARTESIAN_POINT('Ctrl Pts',(-10.0214372954169,-12.9905287409231,
8.38741669750803));
#57815=CARTESIAN_POINT('Ctrl Pts',(-10.0214444951867,-12.9988253788613,
8.38794348863808));
#57816=CARTESIAN_POINT('Ctrl Pts',(-10.0214070037996,-13.0071219499406,
8.38847027976813));
#57817=CARTESIAN_POINT('Ctrl Pts',(-10.0213246224021,-13.0154180752574,
8.38899707089817));
#57818=CARTESIAN_POINT('Ctrl Pts',(-10.0131405502232,-13.8395857937195,
8.44133044668226));
#57819=CARTESIAN_POINT('Ctrl Pts',(-9.56192937252059,-14.6593542074181,
8.49366382246634));
#57820=CARTESIAN_POINT('Ctrl Pts',(-8.86999378518945,-15.1071762134239,
8.54599719825042));
#57821=CARTESIAN_POINT('Ctrl Pts',(-8.17805819785831,-15.5549982194297,
8.59833057403451));
#57822=CARTESIAN_POINT('Ctrl Pts',(-7.24539820089864,-15.6308738177427,
8.6506639498186));
#57823=CARTESIAN_POINT('Ctrl Pts',(-6.49017637768564,-15.300783824577,8.70299732560268));
#57824=CARTESIAN_POINT('Ctrl Pts',(-5.73495455447264,-14.9706938314114,
8.75533070138677));
#57825=CARTESIAN_POINT('Ctrl Pts',(-5.15717090500631,-14.2346382467671,
8.80766407717085));
#57826=CARTESIAN_POINT('Ctrl Pts',(-5.01587750008917,-13.4226311135736,
8.85999745295493));
#57827=CARTESIAN_POINT('Ctrl Pts',(-4.87458409517204,-12.6106239803801,
8.91233082873901));
#57828=CARTESIAN_POINT('Ctrl Pts',(-5.16978093480409,-11.7226652986374,
8.96466420452309));
#57829=CARTESIAN_POINT('Ctrl Pts',(-5.76911509981821,-11.1568756205409,
9.01699758030718));
#57830=CARTESIAN_POINT('Ctrl Pts',(-6.36844926483233,-10.5910859424444,
9.06933095609127));
#57831=CARTESIAN_POINT('Ctrl Pts',(-7.27192075522852,-10.3474652679941,
9.12166433187536));
#57832=CARTESIAN_POINT('Ctrl Pts',(-8.07445379477299,-10.5352420601668,
9.17399770765945));
#57833=CARTESIAN_POINT('Ctrl Pts',(-8.87698683431745,-10.7230188523395,
9.22633108344353));
#57834=CARTESIAN_POINT('Ctrl Pts',(-9.5785814230102,-11.3421931111353,9.27866445922761));
#57835=CARTESIAN_POINT('Ctrl Pts',(-9.86467426114011,-12.1151551560838,
9.33099783501169));
#57836=CARTESIAN_POINT('Ctrl Pts',(-9.96748330192147,-12.3929233341375,
9.34980412251047));
#57837=CARTESIAN_POINT('Ctrl Pts',(-10.0166359465243,-12.6905511117478,
9.36861041000925));
#57838=CARTESIAN_POINT('Ctrl Pts',(-10.014824715197,-12.9887562509003,9.38741669750802));
#57839=CARTESIAN_POINT('Origin',(-7.50000000000001,-12.9903810567666,7.5));
#57840=CARTESIAN_POINT('',(-10.0166114900998,-12.9925168768863,10.387416697508));
#57841=CARTESIAN_POINT('',(-10.0209920718673,-12.9913179799917,10.112583302492));
#57842=CARTESIAN_POINT('',(-10.0175,-12.9903810567666,7.5));
#57843=CARTESIAN_POINT('Ctrl Pts',(-10.0209920718673,-12.9913179799917,
10.112583302492));
#57844=CARTESIAN_POINT('Ctrl Pts',(-10.0172626706847,-12.2214467116455,
10.0637238147899));
#57845=CARTESIAN_POINT('Ctrl Pts',(-9.63824845828795,-11.4483937541634,
10.0148643270877));
#57846=CARTESIAN_POINT('Ctrl Pts',(-9.02557861358329,-10.9828167220247,
9.96600483938563));
#57847=CARTESIAN_POINT('Ctrl Pts',(-8.36934821243818,-10.4841373677117,
9.91367146360155));
#57848=CARTESIAN_POINT('Ctrl Pts',(-7.44505538997194,-10.3382110809426,
9.86133808781746));
#57849=CARTESIAN_POINT('Ctrl Pts',(-6.66711111680735,-10.6104648272364,
9.80900471203337));
#57850=CARTESIAN_POINT('Ctrl Pts',(-5.88916684364275,-10.8827185735301,
9.75667133624929));
#57851=CARTESIAN_POINT('Ctrl Pts',(-5.2575711197798,-11.5731523528866,9.70433796046521));
#57852=CARTESIAN_POINT('Ctrl Pts',(-5.05550299426883,-12.3722067586746,
9.65200458468113));
#57853=CARTESIAN_POINT('Ctrl Pts',(-4.85343486875787,-13.1712611644625,
9.59967120889704));
#57854=CARTESIAN_POINT('Ctrl Pts',(-5.08089434159889,-14.0789361966818,
9.54733783311295));
#57855=CARTESIAN_POINT('Ctrl Pts',(-5.63589882791342,-14.6882714568219,
9.49500445732887));
#57856=CARTESIAN_POINT('Ctrl Pts',(-6.19090331422795,-15.297606716962,9.44267108154478));
#57857=CARTESIAN_POINT('Ctrl Pts',(-7.07345281401599,-15.6086022050228,
9.3903377057607));
#57858=CARTESIAN_POINT('Ctrl Pts',(-7.88785204565785,-15.4818215734849,
9.33800432997662));
#57859=CARTESIAN_POINT('Ctrl Pts',(-8.70225127729972,-15.3550409419471,
9.28567095419253));
#57860=CARTESIAN_POINT('Ctrl Pts',(-9.44850024079541,-14.7904841908106,
9.23333757840844));
#57861=CARTESIAN_POINT('Ctrl Pts',(-9.79201462354332,-14.0412730621545,
9.18100420262436));
#57862=CARTESIAN_POINT('Ctrl Pts',(-9.94171872679729,-13.7147656848908,
9.15819723591356));
#57863=CARTESIAN_POINT('Ctrl Pts',(-10.0149342710371,-13.3531881946364,
9.13539026920277));
#57864=CARTESIAN_POINT('Ctrl Pts',(-10.0138589040853,-12.9911961164478,
9.11258330249198));
#57865=CARTESIAN_POINT('Ctrl Pts',(-10.014824715197,-12.9887562509003,9.38741669750802));
#57866=CARTESIAN_POINT('Ctrl Pts',(-10.0115957252851,-13.5203843049831,
9.42094378579333));
#57867=CARTESIAN_POINT('Ctrl Pts',(-9.84639173717802,-14.053847347733,9.45447087407864));
#57868=CARTESIAN_POINT('Ctrl Pts',(-9.53446863140466,-14.4798917831418,
9.48799796236395));
#57869=CARTESIAN_POINT('Ctrl Pts',(-9.04757907597225,-15.1449165341501,
9.54033133814803));
#57870=CARTESIAN_POINT('Ctrl Pts',(-8.20320887754036,-15.5482162050654,
9.59266471393211));
#57871=CARTESIAN_POINT('Ctrl Pts',(-7.37993546302102,-15.5089697162145,
9.6449980897162));
#57872=CARTESIAN_POINT('Ctrl Pts',(-6.55666204850167,-15.4697232273637,
9.69733146550028));
#57873=CARTESIAN_POINT('Ctrl Pts',(-5.75448541789485,-14.9879305787468,
9.74966484128437));
#57874=CARTESIAN_POINT('Ctrl Pts',(-5.3330653149527,-14.2796053021006,9.80199821706846));
#57875=CARTESIAN_POINT('Ctrl Pts',(-4.91164521201054,-13.5712800254544,
9.85433159285254));
#57876=CARTESIAN_POINT('Ctrl Pts',(-4.87098163673303,-12.636422120779,9.90666496863662));
#57877=CARTESIAN_POINT('Ctrl Pts',(-5.22930629119846,-11.8941806184447,
9.95899834442071));
#57878=CARTESIAN_POINT('Ctrl Pts',(-5.58763094566388,-11.1519391161105,
10.0113317202048));
#57879=CARTESIAN_POINT('Ctrl Pts',(-6.34494382987224,-10.6023140161175,
10.0636650959889));
#57880=CARTESIAN_POINT('Ctrl Pts',(-7.1617000931268,-10.4917304028291,10.115998471773));
#57881=CARTESIAN_POINT('Ctrl Pts',(-7.97845635638136,-10.3811467895407,
10.168331847557));
#57882=CARTESIAN_POINT('Ctrl Pts',(-8.85465599868212,-10.7096046629569,
10.2206652233411));
#57883=CARTESIAN_POINT('Ctrl Pts',(-9.39745068084417,-11.3298422064682,
10.2729985991252));
#57884=CARTESIAN_POINT('Ctrl Pts',(-9.79302701821837,-11.781857128182,10.3111379652528));
#57885=CARTESIAN_POINT('Ctrl Pts',(-10.0115266235871,-12.3888409214585,
10.3492773313804));
#57886=CARTESIAN_POINT('Ctrl Pts',(-10.0166114900998,-12.9925168768863,
10.387416697508));
#57887=CARTESIAN_POINT('Origin',(-7.50000000000001,-12.9903810567666,7.5));
#57888=CARTESIAN_POINT('',(-10.0205077525331,-12.989132710429,11.387416697508));
#57889=CARTESIAN_POINT('',(-10.0159021674261,-12.9883695445715,11.112583302492));
#57890=CARTESIAN_POINT('',(-10.0175,-12.9903810567666,7.5));
#57891=CARTESIAN_POINT('',(-5.5865340033349,-11.3543938533917,12.));
#57892=CARTESIAN_POINT('Ctrl Pts',(-10.0205077525331,-12.989132710429,11.387416697508));
#57893=CARTESIAN_POINT('Ctrl Pts',(-10.0157036585105,-13.732988657673,11.4346110043198));
#57894=CARTESIAN_POINT('Ctrl Pts',(-9.66521749773701,-14.4805837586295,
11.4818053111315));
#57895=CARTESIAN_POINT('Ctrl Pts',(-9.08783263489828,-14.9488474815931,
11.5289996179432));
#57896=CARTESIAN_POINT('Ctrl Pts',(-8.44757534455355,-15.468101244079,11.5813329937273));
#57897=CARTESIAN_POINT('Ctrl Pts',(-7.52831414497493,-15.6438777379762,
11.6336663695114));
#57898=CARTESIAN_POINT('Ctrl Pts',(-6.74219676859447,-15.395694540416,11.6859997452955));
#57899=CARTESIAN_POINT('Ctrl Pts',(-5.956079392214,-15.1475113428559,11.7383331210796));
#57900=CARTESIAN_POINT('Ctrl Pts',(-5.3031058390317,-14.4753684538384,11.7906664968637));
#57901=CARTESIAN_POINT('Ctrl Pts',(-5.07623304195856,-13.6843856961865,
11.8429998726477));
#57902=CARTESIAN_POINT('Ctrl Pts',(-4.84936024488542,-12.8934029385347,
11.8953332484318));
#57903=CARTESIAN_POINT('Ctrl Pts',(-5.04858820392145,-11.9835803122485,
11.9476666242159));
#57904=CARTESIAN_POINT('Ctrl Pts',(-5.5865340033349,-11.3543938533917,12.));
#57905=CARTESIAN_POINT('',(-9.41699369782473,-11.3520708274328,12.));
#57906=CARTESIAN_POINT('Origin',(-7.50000000000001,-12.9903810567666,12.));
#57907=CARTESIAN_POINT('Ctrl Pts',(-9.41700750114216,-11.3520617378123,
12.));
#57908=CARTESIAN_POINT('Ctrl Pts',(-8.90328443334769,-10.7549233049312,
11.9500021225376));
#57909=CARTESIAN_POINT('Ctrl Pts',(-8.08591177198773,-10.4146528382252,
11.9000042450751));
#57910=CARTESIAN_POINT('Ctrl Pts',(-7.30082070365003,-10.4769905890799,
11.8500063676127));
#57911=CARTESIAN_POINT('Ctrl Pts',(-6.47905650106146,-10.5422402577977,
11.7976729918286));
#57912=CARTESIAN_POINT('Ctrl Pts',(-5.69266020241076,-11.048589867075,11.7453396160445));
#57913=CARTESIAN_POINT('Ctrl Pts',(-5.29374176559417,-11.769698237016,11.6930062402604));
#57914=CARTESIAN_POINT('Ctrl Pts',(-4.89482332877758,-12.4908066069571,
11.6406728644763));
#57915=CARTESIAN_POINT('Ctrl Pts',(-4.88338275379511,-13.4266737375619,
11.5883394886922));
#57916=CARTESIAN_POINT('Ctrl Pts',(-5.2647914049726,-14.1573521857831,11.5360061129082));
#57917=CARTESIAN_POINT('Ctrl Pts',(-5.64620005615009,-14.8880306340043,
11.4836727371241));
#57918=CARTESIAN_POINT('Ctrl Pts',(-6.42045793348755,-15.413520399842,11.43133936134));
#57919=CARTESIAN_POINT('Ctrl Pts',(-7.24029923554721,-15.4983927042523,
11.3790059855559));
#57920=CARTESIAN_POINT('Ctrl Pts',(-8.06014053760687,-15.5832650086627,
11.3266726097718));
#57921=CARTESIAN_POINT('Ctrl Pts',(-8.92556526438873,-15.2275198516459,
11.2743392339877));
#57922=CARTESIAN_POINT('Ctrl Pts',(-9.44861922536103,-14.5905668140585,
11.2220058582037));
#57923=CARTESIAN_POINT('Ctrl Pts',(-9.81316607095874,-14.146637051602,11.1855316729664));
#57924=CARTESIAN_POINT('Ctrl Pts',(-10.0114059764305,-13.566110281377,11.1490574877292));
#57925=CARTESIAN_POINT('Ctrl Pts',(-10.0159021674261,-12.9883695445715,
11.112583302492));
#57926=CARTESIAN_POINT('Origin',(-7.50000000000001,-12.9903810567666,14.2084234471775));
#57927=CARTESIAN_POINT('',(-10.5774091090731,-12.9889059662574,4.79157655282255));
#57928=CARTESIAN_POINT('',(-10.5686793840393,-12.990485538642,4.70842344717746));
#57929=CARTESIAN_POINT('',(-10.5735,-12.9903810567665,14.2084234471775));
#57930=CARTESIAN_POINT('',(-6.7062007174672,-15.9596040105123,4.));
#57931=CARTESIAN_POINT('Ctrl Pts',(-10.5686793840393,-12.990485538642,4.70842344717746));
#57932=CARTESIAN_POINT('Ctrl Pts',(-10.568341802375,-12.4708360960575,4.68161580125464));
#57933=CARTESIAN_POINT('Ctrl Pts',(-10.1982941291361,-10.9363980734526,
4.60247477954775));
#57934=CARTESIAN_POINT('Ctrl Pts',(-7.78634786537746,-9.38338007605921,
4.47100038205676));
#57935=CARTESIAN_POINT('Ctrl Pts',(-4.64704854581202,-10.7599538374027,
4.31400025470451));
#57936=CARTESIAN_POINT('Ctrl Pts',(-4.0706083548489,-14.143375884847,4.15700012735225));
#57937=CARTESIAN_POINT('Ctrl Pts',(-5.72985994157699,-15.6985866940351,
4.05233337578409));
#57938=CARTESIAN_POINT('Ctrl Pts',(-6.7062007174672,-15.9596040105123,4.));
#57939=CARTESIAN_POINT('',(-8.29574206058843,-15.9643807808206,4.));
#57940=CARTESIAN_POINT('Origin',(-7.50000000000001,-12.9903810567666,4.));
#57941=CARTESIAN_POINT('Ctrl Pts',(-10.5774091090731,-12.9889059662574,
4.79157655282255));
#57942=CARTESIAN_POINT('Ctrl Pts',(-10.5779245754331,-12.90178610915,4.78704908248048));
#57943=CARTESIAN_POINT('Ctrl Pts',(-10.5353931215559,-11.8081560623987,
4.73018823635433));
#57944=CARTESIAN_POINT('Ctrl Pts',(-9.23195310627391,-9.81262424147309,
4.62099401444409));
#57945=CARTESIAN_POINT('Ctrl Pts',(-5.80479621412607,-9.79242646017958,
4.46399388709183));
#57946=CARTESIAN_POINT('Ctrl Pts',(-3.89775220169895,-12.6409121056472,
4.30699375973959));
#57947=CARTESIAN_POINT('Ctrl Pts',(-5.20118245874298,-15.7537141165304,
4.15232913070897));
#57948=CARTESIAN_POINT('Ctrl Pts',(-7.3659421433414,-16.2099240527811,4.04999787746244));
#57949=CARTESIAN_POINT('Ctrl Pts',(-8.2957496623611,-15.9643994715412,4.));
#57950=CARTESIAN_POINT('Origin',(-7.50000000000001,-12.9903810567666,14.2084234471775));
#57951=CARTESIAN_POINT('',(-10.5688838367077,-12.9896889619566,5.79157655282255));
#57952=CARTESIAN_POINT('',(-10.576720384476,-12.9922616072697,5.70842344717746));
#57953=CARTESIAN_POINT('',(-10.5735,-12.9903810567665,14.2084234471775));
#57954=CARTESIAN_POINT('Ctrl Pts',(-10.576720384476,-12.9922616072697,5.70842344717746));
#57955=CARTESIAN_POINT('Ctrl Pts',(-10.5702730665099,-12.1038642909273,
5.66228272262582));
#57956=CARTESIAN_POINT('Ctrl Pts',(-9.70223177580237,-10.196831424253,5.56380862229009));
#57957=CARTESIAN_POINT('Ctrl Pts',(-6.48106313838945,-9.51757559757857,
5.41300114617028));
#57958=CARTESIAN_POINT('Ctrl Pts',(-4.04127232265978,-11.9244666993329,
5.25600101881803));
#57959=CARTESIAN_POINT('Ctrl Pts',(-4.70303574023142,-15.2872880321773,
5.09900089146577));
#57960=CARTESIAN_POINT('Ctrl Pts',(-7.87270740462966,-16.5902265862243,
4.94200076411352));
#57961=CARTESIAN_POINT('Ctrl Pts',(-10.2242698683325,-14.9942184798723,
4.81180828268408));
#57962=CARTESIAN_POINT('Ctrl Pts',(-10.5690008228703,-13.4852858404724,
4.73394917703873));
#57963=CARTESIAN_POINT('Ctrl Pts',(-10.5686793840393,-12.990485538642,4.70842344717746));
#57964=CARTESIAN_POINT('Ctrl Pts',(-10.5688838367077,-12.9896889619566,
5.79157655282255));
#57965=CARTESIAN_POINT('Ctrl Pts',(-10.5698355434391,-12.5272691260468,
5.76771600385165));
#57966=CARTESIAN_POINT('Ctrl Pts',(-10.2562654399242,-11.0518487505808,
5.69152207909667));
#57967=CARTESIAN_POINT('Ctrl Pts',(-7.98558650367391,-9.40388769480238,
5.56299477855761));
#57968=CARTESIAN_POINT('Ctrl Pts',(-4.77645084555843,-10.6068850809164,
5.40599465120535));
#57969=CARTESIAN_POINT('Ctrl Pts',(-4.00954797596254,-13.9472048059447,
5.24899452385311));
#57970=CARTESIAN_POINT('Ctrl Pts',(-6.37256666156175,-16.4294950347898,
5.09199439650084));
#57971=CARTESIAN_POINT('Ctrl Pts',(-9.64926888537511,-15.8453165147797,
4.93952173949067));
#57972=CARTESIAN_POINT('Ctrl Pts',(-10.5719662603729,-13.908811197287,4.83938245826456));
#57973=CARTESIAN_POINT('Ctrl Pts',(-10.5774091090731,-12.9889059662574,
4.79157655282255));
#57974=CARTESIAN_POINT('Origin',(-7.50000000000001,-12.9903810567666,14.2084234471775));
#57975=CARTESIAN_POINT('',(-10.5752289107932,-12.9928016758089,6.79157655282255));
#57976=CARTESIAN_POINT('',(-10.5729908526269,-12.9877359220758,6.70842344717746));
#57977=CARTESIAN_POINT('',(-10.5735,-12.9903810567665,14.2084234471775));
#57978=CARTESIAN_POINT('Ctrl Pts',(-10.5729908526269,-12.9877359220758,
6.70842344717746));
#57979=CARTESIAN_POINT('Ctrl Pts',(-10.5751989125043,-12.733933626166,6.69528301978108));
#57980=CARTESIAN_POINT('Ctrl Pts',(-10.4312908590873,-11.4718008748884,
6.62980921660061));
#57981=CARTESIAN_POINT('Ctrl Pts',(-8.69550592617927,-9.57431407095109,
6.51200203763606));
#57982=CARTESIAN_POINT('Ctrl Pts',(-5.31022618670948,-10.1087781397346,
6.3550019102838));
#57983=CARTESIAN_POINT('Ctrl Pts',(-3.88853690576949,-13.2272021460562,
6.19800178293155));
#57984=CARTESIAN_POINT('Ctrl Pts',(-5.70528265200966,-16.133268450666,6.0410016555793));
#57985=CARTESIAN_POINT('Ctrl Pts',(-9.13136587582039,-16.22107348372,5.88400152822704));
#57986=CARTESIAN_POINT('Ctrl Pts',(-10.5176208014685,-14.2374825953214,
5.77314212542643));
#57987=CARTESIAN_POINT('Ctrl Pts',(-10.5775856936348,-13.1114954248875,
5.7146160984099));
#57988=CARTESIAN_POINT('Ctrl Pts',(-10.576720384476,-12.9922616072697,5.70842344717746));
#57989=CARTESIAN_POINT('Ctrl Pts',(-10.5752289107932,-12.9928016758089,
6.79157655282255));
#57990=CARTESIAN_POINT('Ctrl Pts',(-10.5680432727522,-12.1600961914245,
6.74838292522283));
#57991=CARTESIAN_POINT('Ctrl Pts',(-9.79183080592196,-10.3066734191141,
6.65285592183901));
#57992=CARTESIAN_POINT('Ctrl Pts',(-6.67544463886838,-9.46634131342536,
6.50499554267114));
#57993=CARTESIAN_POINT('Ctrl Pts',(-4.10581084513197,-11.7341055256468,
6.34799541531887));
#57994=CARTESIAN_POINT('Ctrl Pts',(-4.57977903131249,-15.1283843904584,
6.19099528796663));
#57995=CARTESIAN_POINT('Ctrl Pts',(-7.67233737080682,-16.6054945057935,
6.03399516061437));
#57996=CARTESIAN_POINT('Ctrl Pts',(-10.1638447789511,-15.1090784945035,
5.90085558223301));
#57997=CARTESIAN_POINT('Ctrl Pts',(-10.56774816372,-13.5414952057652,5.82004937963574));
#57998=CARTESIAN_POINT('Ctrl Pts',(-10.5688838367077,-12.9896889619566,
5.79157655282255));
#57999=CARTESIAN_POINT('Origin',(-7.50000000000001,-12.9903810567666,14.2084234471775));
#58000=CARTESIAN_POINT('',(-10.574646672787,-12.9878426425384,7.79157655282256));
#58001=CARTESIAN_POINT('',(-10.5698474628756,-12.992136489652,7.70842344717746));
#58002=CARTESIAN_POINT('',(-10.5735,-12.9903810567665,14.2084234471775));
#58003=CARTESIAN_POINT('Ctrl Pts',(-10.5698474628756,-12.9921364896521,
7.70842344717746));
#58004=CARTESIAN_POINT('Ctrl Pts',(-10.5664962921154,-12.3632928855735,
7.67594994115225));
#58005=CARTESIAN_POINT('Ctrl Pts',(-10.0746937830591,-10.7162100151804,
7.59114305934296));
#58006=CARTESIAN_POINT('Ctrl Pts',(-7.39948645351245,-9.37255790644949,
7.45400280174957));
#58007=CARTESIAN_POINT('Ctrl Pts',(-4.42700232783115,-11.078462500715,7.29700267439732));
#58008=CARTESIAN_POINT('Ctrl Pts',(-4.21010468283033,-14.4988027877182,
7.14000254704507));
#58009=CARTESIAN_POINT('Ctrl Pts',(-6.94328775591919,-16.5665268737914,
6.98300241969282));
#58010=CARTESIAN_POINT('Ctrl Pts',(-9.90513870920436,-15.5228207892163,
6.83914271973694));
#58011=CARTESIAN_POINT('Ctrl Pts',(-10.566405041207,-13.7447326303419,6.74761639556516));
#58012=CARTESIAN_POINT('Ctrl Pts',(-10.5729908526269,-12.9877359220758,
6.70842344717746));
#58013=CARTESIAN_POINT('Ctrl Pts',(-10.574646672787,-12.9878426425384,7.79157655282256));
#58014=CARTESIAN_POINT('Ctrl Pts',(-10.5763836278447,-12.7912348191717,
7.78138322237809));
#58015=CARTESIAN_POINT('Ctrl Pts',(-10.4703648087191,-11.5870913412493,
7.71885651614955));
#58016=CARTESIAN_POINT('Ctrl Pts',(-8.88333183851511,-9.64596167231467,
7.60399643413689));
#58017=CARTESIAN_POINT('Ctrl Pts',(-5.47359881574229,-9.99164028328652,
7.44699630678467));
#58018=CARTESIAN_POINT('Ctrl Pts',(-3.88095917534459,-13.0263185113509,
7.28999617943238));
#58019=CARTESIAN_POINT('Ctrl Pts',(-5.53354816193247,-16.0287712850697,
7.13299605208016));
#58020=CARTESIAN_POINT('Ctrl Pts',(-8.94947337693327,-16.3066703804957,
6.97599592472788));
#58021=CARTESIAN_POINT('Ctrl Pts',(-10.4834449578808,-14.3524988668243,
6.86218942497536));
#58022=CARTESIAN_POINT('Ctrl Pts',(-10.5767493879072,-13.1690017048858,
6.80071630100692));
#58023=CARTESIAN_POINT('Ctrl Pts',(-10.5752289107932,-12.9928016758089,
6.79157655282255));
#58024=CARTESIAN_POINT('Origin',(-7.50000000000001,-12.9903810567666,14.2084234471775));
#58025=CARTESIAN_POINT('',(-10.5690547534087,-12.9913761256565,8.79157655282255));
#58026=CARTESIAN_POINT('',(-10.5783068629449,-12.9905613575631,8.70842344717746));
#58027=CARTESIAN_POINT('',(-10.5735,-12.9903810567665,14.2084234471775));
#58028=CARTESIAN_POINT('Ctrl Pts',(-10.5783068629449,-12.9905613575631,
8.70842344717747));
#58029=CARTESIAN_POINT('Ctrl Pts',(-10.5774424348904,-11.99443969475,8.65661686252343));
#58030=CARTESIAN_POINT('Ctrl Pts',(-9.51496026706992,-9.99048048802178,
8.55247690208529));
#58031=CARTESIAN_POINT('Ctrl Pts',(-6.11666819796815,-9.64596176051859,
8.3960035658631));
#58032=CARTESIAN_POINT('Ctrl Pts',(-3.94738216319582,-12.2992560282264,
8.23900343851084));
#58033=CARTESIAN_POINT('Ctrl Pts',(-4.96376262473273,-15.5722887382593,
8.0820033111586));
#58034=CARTESIAN_POINT('Ctrl Pts',(-8.25441147268027,-16.5301000616477,
7.92500318380633));
#58035=CARTESIAN_POINT('Ctrl Pts',(-10.3278659516785,-14.7722228904523,
7.80047656247929));
#58036=CARTESIAN_POINT('Ctrl Pts',(-10.5718969432977,-13.3767192958943,
7.72828331693634));
#58037=CARTESIAN_POINT('Ctrl Pts',(-10.5698474628756,-12.9921364896521,
7.70842344717746));
#58038=CARTESIAN_POINT('Ctrl Pts',(-10.5690547534086,-12.9913761256565,
8.79157655282255));
#58039=CARTESIAN_POINT('Ctrl Pts',(-10.5673550876409,-12.4192313871019,
8.76205014374926));
#58040=CARTESIAN_POINT('Ctrl Pts',(-10.1411933372985,-10.8306504836598,
8.6801903588919));
#58041=CARTESIAN_POINT('Ctrl Pts',(-7.60051354913579,-9.37255781103892,
8.54599719825042));
#58042=CARTESIAN_POINT('Ctrl Pts',(-4.53789787464541,-10.9107899935683,
8.38899707089818));
#58043=CARTESIAN_POINT('Ctrl Pts',(-4.13142759646044,-14.3138114282651,
8.23199694354591));
#58044=CARTESIAN_POINT('Ctrl Pts',(-6.74558850742372,-16.5301001550025,
8.07499681619368));
#58045=CARTESIAN_POINT('Ctrl Pts',(-9.82259002330375,-15.634475301008,7.92819001928586));
#58046=CARTESIAN_POINT('Ctrl Pts',(-10.5674659613129,-13.8006351479846,
7.83371659816217));
#58047=CARTESIAN_POINT('Ctrl Pts',(-10.574646672787,-12.9878426425384,7.79157655282256));
#58048=CARTESIAN_POINT('Origin',(-7.50000000000001,-12.9903810567666,14.2084234471775));
#58049=CARTESIAN_POINT('',(-10.5777633099838,-12.991524903254,9.79157655282255));
#58050=CARTESIAN_POINT('',(-10.5702338677887,-12.98839740599,9.70842344717746));
#58051=CARTESIAN_POINT('',(-10.5735,-12.9903810567665,14.2084234471775));
#58052=CARTESIAN_POINT('Ctrl Pts',(-10.5702338677887,-12.98839740599,9.70842344717746));
#58053=CARTESIAN_POINT('Ctrl Pts',(-10.5724451168391,-12.6243324625202,
9.68961715967868));
#58054=CARTESIAN_POINT('Ctrl Pts',(-10.3454485117827,-11.2498286970771,
9.61847749639582));
#58055=CARTESIAN_POINT('Ctrl Pts',(-8.32455533939524,-9.46634140643289,
9.49500445732887));
#58056=CARTESIAN_POINT('Ctrl Pts',(-5.01553493137219,-10.3586172470561,
9.33800432997662));
#58057=CARTESIAN_POINT('Ctrl Pts',(-3.93435818466818,-13.6108210305748,
9.18100420262436));
#58058=CARTESIAN_POINT('Ctrl Pts',(-6.05052666129351,-16.3066702930228,
9.02400407527212));
#58059=CARTESIAN_POINT('Ctrl Pts',(-9.46645178620579,-16.0287712049414,
8.86700394791984));
#58060=CARTESIAN_POINT('Ctrl Pts',(-10.5737227704402,-14.0170617812033,
8.76181040522164));
#58061=CARTESIAN_POINT('Ctrl Pts',(-10.5783156528128,-13.0006903413578,
8.70895023830751));
#58062=CARTESIAN_POINT('Ctrl Pts',(-10.5783068629449,-12.9905613575631,
8.70842344717747));
#58063=CARTESIAN_POINT('Ctrl Pts',(-10.5777633099838,-12.991524903254,9.79157655282255));
#58064=CARTESIAN_POINT('Ctrl Pts',(-10.5732102555509,-12.0516244689892,
9.74271706512043));
#58065=CARTESIAN_POINT('Ctrl Pts',(-9.61486894310576,-10.0969521595311,
9.64152420163424));
#58066=CARTESIAN_POINT('Ctrl Pts',(-6.30449404219616,-9.57431398106461,
9.48799796236394));
#58067=CARTESIAN_POINT('Ctrl Pts',(-3.99123550321764,-12.1030705501041,
9.33099783501171));
#58068=CARTESIAN_POINT('Ctrl Pts',(-4.82431993989319,-15.4274866909495,
9.17399770765942));
#58069=CARTESIAN_POINT('Ctrl Pts',(-8.05671225877921,-16.5665269680756,
9.0169975803072));
#58070=CARTESIAN_POINT('Ctrl Pts',(-10.2758761800147,-14.8876717402662,
8.88952386202821));
#58071=CARTESIAN_POINT('Ctrl Pts',(-10.5703676194767,-13.4333156101897,
8.81438351953334));
#58072=CARTESIAN_POINT('Ctrl Pts',(-10.5690547534086,-12.9913761256565,
8.79157655282255));
#58073=CARTESIAN_POINT('Origin',(-7.50000000000001,-12.9903810567666,14.2084234471775));
#58074=CARTESIAN_POINT('',(-10.5715492796759,-12.9879252940133,10.7915765528226));
#58075=CARTESIAN_POINT('',(-10.5724152591149,-12.9929885813497,10.7084234471775));
#58076=CARTESIAN_POINT('',(-10.5735,-12.9903810567665,14.2084234471775));
#58077=CARTESIAN_POINT('Ctrl Pts',(-10.5724152591149,-12.9929885813497,
10.7084234471775));
#58078=CARTESIAN_POINT('Ctrl Pts',(-10.5662073793823,-12.2559883632733,
10.6702840810499));
#58079=CARTESIAN_POINT('Ctrl Pts',(-9.93341873530542,-10.4981249983676,
10.5798113391382));
#58080=CARTESIAN_POINT('Ctrl Pts',(-7.01441350972263,-9.40388779191504,
10.4370052214424));
#58081=CARTESIAN_POINT('Ctrl Pts',(-4.2407080682755,-11.4169238334189,10.2800050940901));
#58082=CARTESIAN_POINT('Ctrl Pts',(-4.38964093653616,-14.8408989317544,
10.1230049667379));
#58083=CARTESIAN_POINT('Ctrl Pts',(-7.32766263366035,-16.6054944100355,
9.96600483938563));
#58084=CARTESIAN_POINT('Ctrl Pts',(-10.049778264125,-15.305320221038,9.82781099953216));
#58085=CARTESIAN_POINT('Ctrl Pts',(-10.5662917424682,-13.6374376539438,
9.74195053546276));
#58086=CARTESIAN_POINT('Ctrl Pts',(-10.5702338677887,-12.98839740599,9.70842344717746));
#58087=CARTESIAN_POINT('Ctrl Pts',(-10.5715492796759,-12.9879252940133,
10.7915765528226));
#58088=CARTESIAN_POINT('Ctrl Pts',(-10.5739360130587,-12.6812405681054,
10.7757173622757));
#58089=CARTESIAN_POINT('Ctrl Pts',(-10.3919168575192,-11.3652990254922,
10.7075247959448));
#58090=CARTESIAN_POINT('Ctrl Pts',(-8.51893689306524,-9.51757549146244,
10.5869988538297));
#58091=CARTESIAN_POINT('Ctrl Pts',(-5.16549637569413,-10.2247238388162,
10.4299987264775));
#58092=CARTESIAN_POINT('Ctrl Pts',(-3.90540678666615,-13.4118934459175,
10.2729985991252));
#58093=CARTESIAN_POINT('Ctrl Pts',(-5.86863408021139,-16.2210735713392,
10.115998471773));
#58094=CARTESIAN_POINT('Ctrl Pts',(-9.29471739586239,-16.133268532241,9.9589983444207));
#58095=CARTESIAN_POINT('Ctrl Pts',(-10.5460797704268,-14.1315894099677,
9.85085770477056));
#58096=CARTESIAN_POINT('Ctrl Pts',(-10.5780870301511,-13.0583514106611,
9.79505044090451));
#58097=CARTESIAN_POINT('Ctrl Pts',(-10.5777633099838,-12.991524903254,9.79157655282255));
#58098=CARTESIAN_POINT('Origin',(-7.50000000000001,-12.9903810567666,14.2084234471775));
#58099=CARTESIAN_POINT('',(-10.5702205181091,-12.9936861301783,11.7915765528225));
#58100=CARTESIAN_POINT('',(-10.5771720267767,-12.9888570081198,11.7084234471775));
#58101=CARTESIAN_POINT('',(-10.5735,-12.9903810567665,14.2084234471775));
#58102=CARTESIAN_POINT('',(-8.29379928253297,-15.9596040105122,12.));
#58103=CARTESIAN_POINT('Ctrl Pts',(-8.29379928253297,-15.9596040105122,
12.));
#58104=CARTESIAN_POINT('Ctrl Pts',(-9.27014005842316,-15.698586694035,11.9476666242159));
#58105=CARTESIAN_POINT('Ctrl Pts',(-10.3714986866323,-14.6662860075735,
11.8781921418234));
#58106=CARTESIAN_POINT('Ctrl Pts',(-10.5724951032558,-13.3253966136884,
11.8087176594309));
#58107=CARTESIAN_POINT('Ctrl Pts',(-10.5702205181091,-12.9936861301783,
11.7915765528225));
#58108=CARTESIAN_POINT('',(-6.70425809489808,-15.964380864449,12.));
#58109=CARTESIAN_POINT('Origin',(-7.50000000000001,-12.9903810567666,12.));
#58110=CARTESIAN_POINT('Ctrl Pts',(-6.70425049788239,-15.9643995452956,
12.));
#58111=CARTESIAN_POINT('Ctrl Pts',(-7.63405808481853,-16.2099241868245,
11.9500021225376));
#58112=CARTESIAN_POINT('Ctrl Pts',(-9.69010316575102,-15.7766245762052,
11.8528099382634));
#58113=CARTESIAN_POINT('Ctrl Pts',(-10.571306929268,-13.8969965329875,11.7556177539892));
#58114=CARTESIAN_POINT('Ctrl Pts',(-10.5771720267767,-12.9888570081198,
11.7084234471775));
#58115=CARTESIAN_POINT('Origin',(-7.50000000000001,-12.9903810567666,4.));
#58116=CARTESIAN_POINT('Ctrl Pts',(-9.41346599666503,-11.3543938533916,
4.));
#58117=CARTESIAN_POINT('Ctrl Pts',(-9.47563125999352,-11.4128139360928,
4.));
#58118=CARTESIAN_POINT('Ctrl Pts',(-9.5344254182292,-11.4744857433087,4.));
#58119=CARTESIAN_POINT('Ctrl Pts',(-9.58983450470078,-11.5390333604437,
4.));
#58120=CARTESIAN_POINT('Ctrl Pts',(-9.64659408185619,-11.6051542024983,
4.));
#58121=CARTESIAN_POINT('Ctrl Pts',(-9.69980203857783,-11.6742932390243,
4.));
#58122=CARTESIAN_POINT('Ctrl Pts',(-9.74941453503823,-11.7460926626337,
4.));
#58123=CARTESIAN_POINT('Ctrl Pts',(-9.76241984954432,-11.7649140111248,
4.));
#58124=CARTESIAN_POINT('Ctrl Pts',(-9.77517792533989,-11.7839183899685,
4.));
#58125=CARTESIAN_POINT('Ctrl Pts',(-9.78768759195629,-11.8030997933617,
4.));
#58126=CARTESIAN_POINT('Ctrl Pts',(-9.79776752365911,-11.8185556198114,
4.));
#58127=CARTESIAN_POINT('Ctrl Pts',(-9.8076865335191,-11.8341271625133,4.));
#58128=CARTESIAN_POINT('Ctrl Pts',(-9.81743537915168,-11.8497970439193,
4.));
#58129=CARTESIAN_POINT('Ctrl Pts',(-9.86491247379083,-11.9261097142127,
4.));
#58130=CARTESIAN_POINT('Ctrl Pts',(-9.90840731623012,-12.0048277686438,
4.));
#58131=CARTESIAN_POINT('Ctrl Pts',(-9.94788306281372,-12.0855595944701,
4.));
#58132=CARTESIAN_POINT('Ctrl Pts',(-9.97942487229752,-12.150065730259,4.));
#58133=CARTESIAN_POINT('Ctrl Pts',(-10.0084002601673,-12.2158586031585,
4.));
#58134=CARTESIAN_POINT('Ctrl Pts',(-10.034773868227,-12.2827556582142,4.));
#58135=CARTESIAN_POINT('Ctrl Pts',(-10.0434527794708,-12.3047698476261,
4.));
#58136=CARTESIAN_POINT('Ctrl Pts',(-10.0518498142904,-12.326903713834,4.));
#58137=CARTESIAN_POINT('Ctrl Pts',(-10.0599633247681,-12.3491510331904,
4.));
#58138=CARTESIAN_POINT('Ctrl Pts',(-10.0673313519173,-12.369354230495,4.));
#58139=CARTESIAN_POINT('Ctrl Pts',(-10.0744669979504,-12.3896556179549,
4.));
#58140=CARTESIAN_POINT('Ctrl Pts',(-10.0813595780794,-12.4100219884372,
4.));
#58141=CARTESIAN_POINT('Ctrl Pts',(-10.110937259752,-12.4974188719965,4.));
#58142=CARTESIAN_POINT('Ctrl Pts',(-10.1360761396945,-12.5860974112731,
4.));
#58143=CARTESIAN_POINT('Ctrl Pts',(-10.1567415216565,-12.6756607739627,
4.));
#58144=CARTESIAN_POINT('Ctrl Pts',(-10.1777235800004,-12.7665966059193,
4.));
#58145=CARTESIAN_POINT('Ctrl Pts',(-10.194094489083,-12.8584453915162,4.));
#58146=CARTESIAN_POINT('Ctrl Pts',(-10.205776157801,-12.9508249271276,4.));
#58147=CARTESIAN_POINT('Ctrl Pts',(-10.2173669041142,-13.0424854413619,
4.));
#58148=CARTESIAN_POINT('Ctrl Pts',(-10.2243414700862,-13.1346694027891,
4.00000000000001));
#58149=CARTESIAN_POINT('Ctrl Pts',(-10.2265766240073,-13.2270226781325,
4.00000000000001));
#58150=CARTESIAN_POINT('Ctrl Pts',(-10.2276561070688,-13.2716253318781,
4.00000000000001));
#58151=CARTESIAN_POINT('Ctrl Pts',(-10.2276293996605,-13.3162676791034,
4.00000000000001));
#58152=CARTESIAN_POINT('Ctrl Pts',(-10.2264782755414,-13.360910468216,4.00000000000001));
#58153=CARTESIAN_POINT('Ctrl Pts',(-10.2261080116976,-13.3752700063553,
4.00000000000001));
#58154=CARTESIAN_POINT('Ctrl Pts',(-10.2256213911499,-13.3896295910271,
4.00000000000001));
#58155=CARTESIAN_POINT('Ctrl Pts',(-10.2250177409671,-13.40398791621,4.00000000000001));
#58156=CARTESIAN_POINT('Ctrl Pts',(-10.2243866916487,-13.4189979527825,
4.00000000000001));
#58157=CARTESIAN_POINT('Ctrl Pts',(-10.2236280724728,-13.4339981404011,
4.));
#58158=CARTESIAN_POINT('Ctrl Pts',(-10.2227419311859,-13.4489814918393,
4.));
#58159=CARTESIAN_POINT('Ctrl Pts',(-10.2170924746832,-13.5445055278686,
4.));
#58160=CARTESIAN_POINT('Ctrl Pts',(-10.2062608557766,-13.6394136430286,
4.));
#58161=CARTESIAN_POINT('Ctrl Pts',(-10.1901745261949,-13.7333115332678,
4.));
#58162=CARTESIAN_POINT('Ctrl Pts',(-10.1886860667379,-13.74199985474,4.));
#58163=CARTESIAN_POINT('Ctrl Pts',(-10.1871525835688,-13.7506795401449,
4.));
#58164=CARTESIAN_POINT('Ctrl Pts',(-10.1855739978038,-13.7593502843482,
4.));
#58165=CARTESIAN_POINT('Ctrl Pts',(-10.1691852106353,-13.8493694549782,
4.));
#58166=CARTESIAN_POINT('Ctrl Pts',(-10.1479394797701,-13.9384246529327,
4.));
#58167=CARTESIAN_POINT('Ctrl Pts',(-10.1221390901744,-14.0262810420052,
4.));
#58168=CARTESIAN_POINT('Ctrl Pts',(-10.0957476132678,-14.1161502222633,
4.));
#58169=CARTESIAN_POINT('Ctrl Pts',(-10.0645901923201,-14.2047657338476,
4.));
#58170=CARTESIAN_POINT('Ctrl Pts',(-10.0289360631668,-14.2918733204662,
4.));
#58171=CARTESIAN_POINT('Ctrl Pts',(-10.0090443370482,-14.3404713453517,
4.));
#58172=CARTESIAN_POINT('Ctrl Pts',(-9.98775201258348,-14.3885999003503,
4.));
#58173=CARTESIAN_POINT('Ctrl Pts',(-9.96509914777034,-14.4362131753606,
4.));
#58174=CARTESIAN_POINT('Ctrl Pts',(-9.95876399288502,-14.4495288188465,
4.));
#58175=CARTESIAN_POINT('Ctrl Pts',(-9.95232213153922,-14.4628045348086,
4.));
#58176=CARTESIAN_POINT('Ctrl Pts',(-9.94578145907892,-14.4760254702856,
4.));
#58177=CARTESIAN_POINT('Ctrl Pts',(-9.90302407067229,-14.562452772175,4.));
#58178=CARTESIAN_POINT('Ctrl Pts',(-9.85598091444247,-14.6466834011242,
4.));
#58179=CARTESIAN_POINT('Ctrl Pts',(-9.80499202080536,-14.7284640330205,
4.));
#58180=CARTESIAN_POINT('Ctrl Pts',(-9.75299794500559,-14.8118568676255,
4.));
#58181=CARTESIAN_POINT('Ctrl Pts',(-9.69690071688324,-14.8927029338428,
4.));
#58182=CARTESIAN_POINT('Ctrl Pts',(-9.63700597453379,-14.9707266774082,
4.));
#58183=CARTESIAN_POINT('Ctrl Pts',(-9.57663995749172,-15.049364341567,4.));
#58184=CARTESIAN_POINT('Ctrl Pts',(-9.51241597456512,-15.1251359367173,
4.));
#58185=CARTESIAN_POINT('Ctrl Pts',(-9.44459769690279,-15.1977400638646,
4.));
#58186=CARTESIAN_POINT('Ctrl Pts',(-9.40866340733751,-15.2362101904805,
4.));
#58187=CARTESIAN_POINT('Ctrl Pts',(-9.37171922385876,-15.2737906405076,
4.));
#58188=CARTESIAN_POINT('Ctrl Pts',(-9.33379951949355,-15.3104331478965,
4.));
#58189=CARTESIAN_POINT('Ctrl Pts',(-9.31851290781191,-15.3252048817713,
4.));
#58190=CARTESIAN_POINT('Ctrl Pts',(-9.30306772443973,-15.339824154646,4.));
#58191=CARTESIAN_POINT('Ctrl Pts',(-9.28746608368795,-15.3542876681649,
4.));
#58192=CARTESIAN_POINT('Ctrl Pts',(-9.27676581806402,-15.3642073579572,
4.));
#58193=CARTESIAN_POINT('Ctrl Pts',(-9.26599878272636,-15.3740474389504,
4.));
#58194=CARTESIAN_POINT('Ctrl Pts',(-9.25516737653956,-15.3838058321128,
4.));
#58195=CARTESIAN_POINT('Ctrl Pts',(-9.17938057199806,-15.452084818468,4.));
#58196=CARTESIAN_POINT('Ctrl Pts',(-9.10042438929677,-15.5163865482147,
4.));
#58197=CARTESIAN_POINT('Ctrl Pts',(-9.01862162231471,-15.5764248312756,
4.));
#58198=CARTESIAN_POINT('Ctrl Pts',(-8.93674927983158,-15.636514178546,4.));
#58199=CARTESIAN_POINT('Ctrl Pts',(-8.8520249381574,-15.6923336670045,4.));
#58200=CARTESIAN_POINT('Ctrl Pts',(-8.76472731465809,-15.7435701437727,
4.));
#58201=CARTESIAN_POINT('Ctrl Pts',(-8.67912044767158,-15.7938142864623,
4.));
#58202=CARTESIAN_POINT('Ctrl Pts',(-8.59103835537406,-15.8396519102272,
4.));
#58203=CARTESIAN_POINT('Ctrl Pts',(-8.50070999295064,-15.8807513482254,
4.));
#58204=CARTESIAN_POINT('Ctrl Pts',(-8.47449902628609,-15.8926773476613,
4.));
#58205=CARTESIAN_POINT('Ctrl Pts',(-8.44809873411205,-15.9042041128398,
4.));
#58206=CARTESIAN_POINT('Ctrl Pts',(-8.42151428132428,-15.9153228238725,
4.));
#58207=CARTESIAN_POINT('Ctrl Pts',(-8.38003054177093,-15.9326730291346,
4.));
#58208=CARTESIAN_POINT('Ctrl Pts',(-8.3380984052677,-15.9490297174903,4.));
#58209=CARTESIAN_POINT('Ctrl Pts',(-8.29574966236114,-15.9643994715412,
4.));
#58210=CARTESIAN_POINT('Ctrl Pts',(-6.7062007174672,-15.9596040105123,4.));
#58211=CARTESIAN_POINT('Ctrl Pts',(-6.61134542475377,-15.9249055207219,
4.));
#58212=CARTESIAN_POINT('Ctrl Pts',(-6.51853060534356,-15.8852234998271,
4.));
#58213=CARTESIAN_POINT('Ctrl Pts',(-6.42799851956089,-15.8408762347418,
4.));
#58214=CARTESIAN_POINT('Ctrl Pts',(-6.33621693362306,-15.7959169003098,
4.));
#58215=CARTESIAN_POINT('Ctrl Pts',(-6.24678085823289,-15.7461619565544,
4.));
#58216=CARTESIAN_POINT('Ctrl Pts',(-6.15997674190851,-15.691902411869,4.));
#58217=CARTESIAN_POINT('Ctrl Pts',(-6.13531568434349,-15.6764872701499,
4.));
#58218=CARTESIAN_POINT('Ctrl Pts',(-6.11086730231581,-15.6607083372246,
4.));
#58219=CARTESIAN_POINT('Ctrl Pts',(-6.08663877235659,-15.6445718215519,
4.));
#58220=CARTESIAN_POINT('Ctrl Pts',(-6.06744081682964,-15.6317857337964,
4.));
#58221=CARTESIAN_POINT('Ctrl Pts',(-6.0483789202221,-15.6187736030245,4.));
#58222=CARTESIAN_POINT('Ctrl Pts',(-6.02947561532874,-15.6055520498285,
4.));
#58223=CARTESIAN_POINT('Ctrl Pts',(-5.94677128184633,-15.5477060937462,
4.));
#58224=CARTESIAN_POINT('Ctrl Pts',(-5.86702045523495,-15.485803012119,4.));
#58225=CARTESIAN_POINT('Ctrl Pts',(-5.79049058680189,-15.4201377361794,
4.));
#58226=CARTESIAN_POINT('Ctrl Pts',(-5.73202513270763,-15.3699723529815,
4.));
#58227=CARTESIAN_POINT('Ctrl Pts',(-5.67544017028651,-15.3176103400047,
4.));
#58228=CARTESIAN_POINT('Ctrl Pts',(-5.62087197491949,-15.2631717733717,
4.));
#58229=CARTESIAN_POINT('Ctrl Pts',(-5.59237459351674,-15.2347420885356,
4.));
#58230=CARTESIAN_POINT('Ctrl Pts',(-5.56442750315923,-15.2057459282144,
4.));
#58231=CARTESIAN_POINT('Ctrl Pts',(-5.53705194133909,-15.1761996365986,
4.));
#58232=CARTESIAN_POINT('Ctrl Pts',(-5.52590419986363,-15.1641679412254,
4.));
#58233=CARTESIAN_POINT('Ctrl Pts',(-5.51485102559337,-15.1520446566585,
4.));
#58234=CARTESIAN_POINT('Ctrl Pts',(-5.50390395570898,-15.1398423958921,
4.));
#58235=CARTESIAN_POINT('Ctrl Pts',(-5.43813919199008,-15.0665370452716,
4.));
#58236=CARTESIAN_POINT('Ctrl Pts',(-5.37610812852687,-14.9902855415477,
4.));
#58237=CARTESIAN_POINT('Ctrl Pts',(-5.31805567958009,-14.9113640105217,
4.));
#58238=CARTESIAN_POINT('Ctrl Pts',(-5.26107088016972,-14.8338939348183,
4.));
#58239=CARTESIAN_POINT('Ctrl Pts',(-5.20791934818337,-14.7538503489036,
4.));
#58240=CARTESIAN_POINT('Ctrl Pts',(-5.15887699703074,-14.6714727381725,
4.));
#58241=CARTESIAN_POINT('Ctrl Pts',(-5.11076871641508,-14.5906641080731,
4.));
#58242=CARTESIAN_POINT('Ctrl Pts',(-5.0666142946296,-14.5076088453843,4.));
#58243=CARTESIAN_POINT('Ctrl Pts',(-5.02672179249125,-14.4225226052514,
4.));
#58244=CARTESIAN_POINT('Ctrl Pts',(-5.00642778712802,-14.3792377642152,
4.));
#58245=CARTESIAN_POINT('Ctrl Pts',(-4.98723753203067,-14.3354272137238,
4.));
#58246=CARTESIAN_POINT('Ctrl Pts',(-4.96919681035721,-14.2911191061582,
4.));
#58247=CARTESIAN_POINT('Ctrl Pts',(-4.96034382211253,-14.2693761203441,
4.));
#58248=CARTESIAN_POINT('Ctrl Pts',(-4.95176770738618,-14.2475133193776,
4.));
#58249=CARTESIAN_POINT('Ctrl Pts',(-4.94347420847157,-14.2255340469214,
4.));
#58250=CARTESIAN_POINT('Ctrl Pts',(-4.93874143956184,-14.2129913531307,
4.));
#58251=CARTESIAN_POINT('Ctrl Pts',(-4.93410201278753,-14.2004140677721,
4.));
#58252=CARTESIAN_POINT('Ctrl Pts',(-4.92955955708199,-14.1878106688628,
4.));
#58253=CARTESIAN_POINT('Ctrl Pts',(-4.89805327414987,-14.1003940207578,
4.));
#58254=CARTESIAN_POINT('Ctrl Pts',(-4.87116570943181,-14.0116107665047,
4.));
#58255=CARTESIAN_POINT('Ctrl Pts',(-4.8491500138814,-13.9216823090563,4.));
#58256=CARTESIAN_POINT('Ctrl Pts',(-4.84589778208928,-13.9083977781333,
4.));
#58257=CARTESIAN_POINT('Ctrl Pts',(-4.84275195632634,-13.8950882390595,
4.));
#58258=CARTESIAN_POINT('Ctrl Pts',(-4.8397134492654,-13.8817543903633,4.));
#58259=CARTESIAN_POINT('Ctrl Pts',(-4.81880165443801,-13.7899873802489,
4.));
#58260=CARTESIAN_POINT('Ctrl Pts',(-4.80296876416446,-13.6970686989268,
4.));
#58261=CARTESIAN_POINT('Ctrl Pts',(-4.7921064004091,-13.6033902081318,4.));
#58262=CARTESIAN_POINT('Ctrl Pts',(-4.78082403916422,-13.5060896023125,
4.));
#58263=CARTESIAN_POINT('Ctrl Pts',(-4.77490405625791,-13.4079680956598,
4.));
#58264=CARTESIAN_POINT('Ctrl Pts',(-4.77428165528829,-13.3094781487529,
4.));
#58265=CARTESIAN_POINT('Ctrl Pts',(-4.77410059584044,-13.2808269475559,
4.));
#58266=CARTESIAN_POINT('Ctrl Pts',(-4.77436819825548,-13.2521447164312,
4.));
#58267=CARTESIAN_POINT('Ctrl Pts',(-4.77508370765677,-13.2234430275403,
4.));
#58268=CARTESIAN_POINT('Ctrl Pts',(-4.77547928901581,-13.2075748180131,
4.));
#58269=CARTESIAN_POINT('Ctrl Pts',(-4.77601178481995,-13.19170066513,4.));
#58270=CARTESIAN_POINT('Ctrl Pts',(-4.77668111451686,-13.175822557735,4.));
#58271=CARTESIAN_POINT('Ctrl Pts',(-4.77726173830688,-13.1620487674244,
4.));
#58272=CARTESIAN_POINT('Ctrl Pts',(-4.77794533193815,-13.1482734031105,
4.));
#58273=CARTESIAN_POINT('Ctrl Pts',(-4.77873092865176,-13.1345098810533,
4.));
#58274=CARTESIAN_POINT('Ctrl Pts',(-4.78403323232826,-13.0416144140266,
4.));
#58275=CARTESIAN_POINT('Ctrl Pts',(-4.79398378921199,-12.9491067853577,
4.));
#58276=CARTESIAN_POINT('Ctrl Pts',(-4.8084638797429,-12.8573599583,4.));
#58277=CARTESIAN_POINT('Ctrl Pts',(-4.82290323568455,-12.7658712283383,
4.));
#58278=CARTESIAN_POINT('Ctrl Pts',(-4.84184708120934,-12.6751380809488,
4.));
#58279=CARTESIAN_POINT('Ctrl Pts',(-4.86522624014646,-12.5855474359577,
4.));
#58280=CARTESIAN_POINT('Ctrl Pts',(-4.88820176586815,-12.4975035429353,
4.));
#58281=CARTESIAN_POINT('Ctrl Pts',(-4.9154612393753,-12.4105622603287,4.));
#58282=CARTESIAN_POINT('Ctrl Pts',(-4.94697939694318,-12.3251200100783,
4.));
#58283=CARTESIAN_POINT('Ctrl Pts',(-4.96237184169077,-12.2833927894037,
4.));
#58284=CARTESIAN_POINT('Ctrl Pts',(-4.9787805689918,-12.2420236106898,4.));
#58285=CARTESIAN_POINT('Ctrl Pts',(-4.99620574112456,-12.2010620870672,
4.));
#58286=CARTESIAN_POINT('Ctrl Pts',(-5.00196784663073,-12.1875170489459,
4.));
#58287=CARTESIAN_POINT('Ctrl Pts',(-5.00784111328384,-12.1740166075363,
4.));
#58288=CARTESIAN_POINT('Ctrl Pts',(-5.01382559232837,-12.160562620369,4.));
#58289=CARTESIAN_POINT('Ctrl Pts',(-5.01951333079912,-12.1477757495608,
4.));
#58290=CARTESIAN_POINT('Ctrl Pts',(-5.02529810648898,-12.135038576554,4.));
#58291=CARTESIAN_POINT('Ctrl Pts',(-5.0311780316899,-12.1223558509962,4.));
#58292=CARTESIAN_POINT('Ctrl Pts',(-5.06862974733614,-12.0415742398394,
4.));
#58293=CARTESIAN_POINT('Ctrl Pts',(-5.10995835566621,-11.9629538753605,
4.));
#58294=CARTESIAN_POINT('Ctrl Pts',(-5.15509810659155,-11.8868432541903,
4.));
#58295=CARTESIAN_POINT('Ctrl Pts',(-5.19948167106006,-11.8120076471655,
4.));
#58296=CARTESIAN_POINT('Ctrl Pts',(-5.24755020547363,-11.739597730264,4.));
#58297=CARTESIAN_POINT('Ctrl Pts',(-5.29927754869182,-11.6699789932549,
4.));
#58298=CARTESIAN_POINT('Ctrl Pts',(-5.34947355289339,-11.6024212530347,
4.));
#58299=CARTESIAN_POINT('Ctrl Pts',(-5.40311537622297,-11.5374914288171,
4.));
#58300=CARTESIAN_POINT('Ctrl Pts',(-5.46020711675472,-11.4755639671884,
4.));
#58301=CARTESIAN_POINT('Ctrl Pts',(-5.47440621920022,-11.4601621881628,
4.));
#58302=CARTESIAN_POINT('Ctrl Pts',(-5.48881883821923,-11.4449463392586,
4.));
#58303=CARTESIAN_POINT('Ctrl Pts',(-5.50344527039708,-11.4299226339363,
4.));
#58304=CARTESIAN_POINT('Ctrl Pts',(-5.52930152881858,-11.4033640855126,
4.));
#58305=CARTESIAN_POINT('Ctrl Pts',(-5.55582596313967,-11.37740591447,4.));
#58306=CARTESIAN_POINT('Ctrl Pts',(-5.58299257280551,-11.3520616136783,
4.));
#58307=CARTESIAN_POINT('Origin',(-7.50000000000001,-12.9903810567666,14.2084234471775));
#58308=CARTESIAN_POINT('Ctrl Pts',(-10.5771720267767,-12.9888570081198,
11.7084234471775));
#58309=CARTESIAN_POINT('Ctrl Pts',(-10.5778106872988,-12.8899681384638,
11.7032843782051));
#58310=CARTESIAN_POINT('Ctrl Pts',(-10.5289895265855,-11.7846562178796,
11.6458119334487));
#58311=CARTESIAN_POINT('Ctrl Pts',(-9.19520367525283,-9.79242641580684,
11.5360061129082));
#58312=CARTESIAN_POINT('Ctrl Pts',(-5.76804697299906,-9.81262440187857,
11.3790059855559));
#58313=CARTESIAN_POINT('Ctrl Pts',(-3.89395285925593,-12.6818121943635,
11.2220058582037));
#58314=CARTESIAN_POINT('Ctrl Pts',(-5.25343392007517,-15.8279700706855,
11.0650057308514));
#58315=CARTESIAN_POINT('Ctrl Pts',(-8.62743330425189,-16.429494929522,10.9080056034992));
#58316=CARTESIAN_POINT('Ctrl Pts',(-10.4164139750736,-14.5502168635008,
10.7891448422745));
#58317=CARTESIAN_POINT('Ctrl Pts',(-10.5747255939164,-13.2672718029744,
10.7226174568339));
#58318=CARTESIAN_POINT('Ctrl Pts',(-10.5724152591149,-12.9929885813497,
10.7084234471775));
#58319=CARTESIAN_POINT('Ctrl Pts',(-10.5702205181091,-12.9936861301783,
11.7915765528225));
#58320=CARTESIAN_POINT('Ctrl Pts',(-10.5655505854978,-12.3126539838428,
11.7563842836469));
#58321=CARTESIAN_POINT('Ctrl Pts',(-10.0102062672903,-10.6096615213504,
11.6688586386871));
#58322=CARTESIAN_POINT('Ctrl Pts',(-7.21365210721562,-9.38337955935061,
11.5289996179432));
#58323=CARTESIAN_POINT('Ctrl Pts',(-4.33342685529555,-11.2379164301912,
11.371999490591));
#58324=CARTESIAN_POINT('Ctrl Pts',(-4.29152503935676,-14.6655878811314,
11.2149993632387));
#58325=CARTESIAN_POINT('Ctrl Pts',(-7.12729256983938,-16.5902267633183,
11.0579992358865));
#58326=CARTESIAN_POINT('Ctrl Pts',(-9.97678353025252,-15.4189029291823,
10.9168582990811));
#58327=CARTESIAN_POINT('Ctrl Pts',(-10.5660600868159,-13.6932623961271,
10.8280507380598));
#58328=CARTESIAN_POINT('Ctrl Pts',(-10.5715492796759,-12.9879252940133,
10.7915765528226));
#58329=CARTESIAN_POINT('Ctrl Pts',(-5.5865340033349,-11.3543938533917,12.));
#58330=CARTESIAN_POINT('Ctrl Pts',(-5.04858820392145,-11.9835803122485,
11.9476666242159));
#58331=CARTESIAN_POINT('Ctrl Pts',(-4.6501322858494,-13.8032255648209,11.8429998726477));
#58332=CARTESIAN_POINT('Ctrl Pts',(-6.60905294539631,-15.8196542318734,
11.6859997452955));
#58333=CARTESIAN_POINT('Ctrl Pts',(-9.36683654413216,-15.2923247501818,
11.5289996179432));
#58334=CARTESIAN_POINT('Ctrl Pts',(-10.4505966874647,-12.7041316569579,
11.371999490591));
#58335=CARTESIAN_POINT('Ctrl Pts',(-8.88853920691362,-10.3709404162538,
11.2149993632387));
#58336=CARTESIAN_POINT('Ctrl Pts',(-6.08135944510335,-10.3874845613442,
11.0579992358865));
#58337=CARTESIAN_POINT('Ctrl Pts',(-4.54629130410829,-12.737632688099,10.9009991085342));
#58338=CARTESIAN_POINT('Ctrl Pts',(-5.65984053808011,-15.31464666358,10.743998981182));
#58339=CARTESIAN_POINT('Ctrl Pts',(-8.42347920724065,-15.8073549219566,
10.5869988538297));
#58340=CARTESIAN_POINT('Ctrl Pts',(-10.3590248070529,-13.7741141771921,
10.4299987264775));
#58341=CARTESIAN_POINT('Ctrl Pts',(-9.73085564098287,-11.0380625363732,
10.2729985991252));
#58342=CARTESIAN_POINT('Ctrl Pts',(-7.1022567140806,-10.0526889161244,10.115998471773));
#58343=CARTESIAN_POINT('Ctrl Pts',(-4.83031806145553,-11.7015642161036,
9.9589983444207));
#58344=CARTESIAN_POINT('Ctrl Pts',(-4.95230878728804,-14.5061379301299,
9.80199821706846));
#58345=CARTESIAN_POINT('Ctrl Pts',(-7.35883867910848,-15.9515158759806,
9.64499808971619));
#58346=CARTESIAN_POINT('Ctrl Pts',(-9.89194927440413,-14.7416168632348,
9.48799796236395));
#58347=CARTESIAN_POINT('Ctrl Pts',(-10.2801760117029,-11.961367369931,9.33099783501168));
#58348=CARTESIAN_POINT('Ctrl Pts',(-8.17539224562471,-10.1038445935438,
9.17399770765945));
#58349=CARTESIAN_POINT('Ctrl Pts',(-5.46497777443614,-10.8347066168947,
9.01699758030717));
#58350=CARTESIAN_POINT('Ctrl Pts',(-4.57938725553999,-13.4985826621227,
8.85999745295493));
#58351=CARTESIAN_POINT('Ctrl Pts',(-6.31273820393898,-15.7067494160557,
8.70299732560268));
#58352=CARTESIAN_POINT('Ctrl Pts',(-9.11071819481798,-15.4791226211167,
8.54599719825042));
#58353=CARTESIAN_POINT('Ctrl Pts',(-10.4643517279258,-13.0198173800209,
8.38899707089818));
#58354=CARTESIAN_POINT('Ctrl Pts',(-9.15982262789147,-10.5341163103444,
8.23199694354591));
#58355=CARTESIAN_POINT('Ctrl Pts',(-6.3669146537774,-10.2509714005752,8.07499681619367));
#58356=CARTESIAN_POINT('Ctrl Pts',(-4.59005518003756,-12.4242814116226,
7.9179966888414));
#58357=CARTESIAN_POINT('Ctrl Pts',(-5.42257114292002,-15.1052184044673,
7.76099656148916));
#58358=CARTESIAN_POINT('Ctrl Pts',(-8.11793749226372,-15.8897604596585,
7.60399643413691));
#58359=CARTESIAN_POINT('Ctrl Pts',(-10.259193363348,-14.0744011876836,7.44699630678465));
#58360=CARTESIAN_POINT('Ctrl Pts',(-9.92625407643148,-11.286990666814,7.2899961794324));
#58361=CARTESIAN_POINT('Ctrl Pts',(-7.4176694799797,-10.0270266461848,7.13299605208014));
#58362=CARTESIAN_POINT('Ctrl Pts',(-4.98291145609725,-11.4243309624572,
6.97599592472789));
#58363=CARTESIAN_POINT('Ctrl Pts',(-4.80525086677252,-14.2259274070742,
6.81899579737564));
#58364=CARTESIAN_POINT('Ctrl Pts',(-7.04399769823543,-15.9195976158556,
6.66199567002339));
#58365=CARTESIAN_POINT('Ctrl Pts',(-9.69164612773492,-14.986611176204,6.50499554267113));
#58366=CARTESIAN_POINT('Ctrl Pts',(-10.3740245283272,-12.2635861515028,
6.34799541531888));
#58367=CARTESIAN_POINT('Ctrl Pts',(-8.47923740659063,-10.1922848677994,
6.19099528796662));
#58368=CARTESIAN_POINT('Ctrl Pts',(-5.70635901253982,-10.630063717047,6.03399516061437));
#58369=CARTESIAN_POINT('Ctrl Pts',(-4.54185510339179,-13.1843609143513,
5.87699503326211));
#58370=CARTESIAN_POINT('Ctrl Pts',(-6.02994926840226,-15.5647161841919,
5.71999490590987));
#58371=CARTESIAN_POINT('Ctrl Pts',(-8.83624974536451,-15.636637176778,5.5629947785576));
#58372=CARTESIAN_POINT('Ctrl Pts',(-10.4443267219795,-13.3356413212244,
5.40599465120536));
#58373=CARTESIAN_POINT('Ctrl Pts',(-9.41218894167164,-10.7250347470945,
5.2489945238531));
#58374=CARTESIAN_POINT('Ctrl Pts',(-6.66539009301951,-10.1458104553331,
5.09199439650085));
#58375=CARTESIAN_POINT('Ctrl Pts',(-4.66696049204361,-12.1172919418034,
4.93499426914859));
#58376=CARTESIAN_POINT('Ctrl Pts',(-5.20901007842283,-14.8717746831197,
4.77799414179635));
#58377=CARTESIAN_POINT('Ctrl Pts',(-7.80528416826264,-15.9390100206221,
4.62099401444409));
#58378=CARTESIAN_POINT('Ctrl Pts',(-10.1280577671037,-14.362540949444,4.46399388709183));
#58379=CARTESIAN_POINT('Ctrl Pts',(-10.0937360173612,-11.5549393117934,
4.30699375973958));
#58380=CARTESIAN_POINT('Ctrl Pts',(-7.73454717783886,-10.0358910717557,
4.14999363238733));
#58381=CARTESIAN_POINT('Ctrl Pts',(-5.16315103760592,-11.163440915316,3.99299350503507));
#58382=CARTESIAN_POINT('Ctrl Pts',(-4.69098959926211,-13.9347976761557,
3.83599337768283));
#58383=CARTESIAN_POINT('Ctrl Pts',(-6.05008049550027,-15.2086689018369,
3.73132662611465));
#58384=CARTESIAN_POINT('Ctrl Pts',(-6.84980000202495,-15.4224678588017,
3.67899325033057));
#58385=CARTESIAN_POINT('Ctrl Pts',(-5.44566844965787,-11.2339557355398,
12.1070022498898));
#58386=CARTESIAN_POINT('Ctrl Pts',(-4.86812015246569,-11.9094616477066,
12.0546688741057));
#58387=CARTESIAN_POINT('Ctrl Pts',(-4.44033070371531,-13.8630655577342,
11.9500021225376));
#58388=CARTESIAN_POINT('Ctrl Pts',(-6.54346319864229,-16.0279396850822,
11.7930019951853));
#58389=CARTESIAN_POINT('Ctrl Pts',(-9.50426933043305,-15.4617892577673,
11.6360018678331));
#58390=CARTESIAN_POINT('Ctrl Pts',(-10.6678137358898,-12.6830585465582,
11.4790017404808));
#58391=CARTESIAN_POINT('Ctrl Pts',(-8.99076069636001,-10.1781024161048,
11.3220016131285));
#58392=CARTESIAN_POINT('Ctrl Pts',(-5.97692195440192,-10.195864508189,11.1650014857763));
#58393=CARTESIAN_POINT('Ctrl Pts',(-4.32884515582416,-12.7190258568539,
11.008001358424));
#58394=CARTESIAN_POINT('Ctrl Pts',(-5.52437166541181,-15.4857544659485,
10.8510012310718));
#58395=CARTESIAN_POINT('Ctrl Pts',(-8.49146390624439,-16.0147349244784,
10.6940011037195));
#58396=CARTESIAN_POINT('Ctrl Pts',(-10.569500516119,-13.831811047759,10.5370009763673));
#58397=CARTESIAN_POINT('Ctrl Pts',(-9.89508678780663,-10.8943367373214,
10.380000849015));
#58398=CARTESIAN_POINT('Ctrl Pts',(-7.07297564596128,-9.83642187472128,
10.2230007216628));
#58399=CARTESIAN_POINT('Ctrl Pts',(-4.6337813970622,-11.606684088542,10.0660005943105));
#58400=CARTESIAN_POINT('Ctrl Pts',(-4.76475283703741,-14.6177249306714,
9.90900046695826));
#58401=CARTESIAN_POINT('Ctrl Pts',(-7.34844666395912,-16.1695087206656,
9.75200033960601));
#58402=CARTESIAN_POINT('Ctrl Pts',(-10.0680398135062,-14.8705393535885,
9.59500021225375));
#58403=CARTESIAN_POINT('Ctrl Pts',(-10.4848470295787,-11.8856134328399,
9.43800008490151));
#58404=CARTESIAN_POINT('Ctrl Pts',(-8.22511327688156,-9.89134353117351,
9.28099995754925));
#58405=CARTESIAN_POINT('Ctrl Pts',(-5.31516349341482,-10.6760101602818,
9.123999830197));
#58406=CARTESIAN_POINT('Ctrl Pts',(-4.36437756524938,-13.5359954516068,
8.96699970284473));
#58407=CARTESIAN_POINT('Ctrl Pts',(-6.22533435639049,-15.9067230417114,
8.80999957549251));
#58408=CARTESIAN_POINT('Ctrl Pts',(-9.22929605861391,-15.6623388157249,
8.65299944814021));
#58409=CARTESIAN_POINT('Ctrl Pts',(-10.6825813950197,-13.0219844234806,
8.495999320788));
#58410=CARTESIAN_POINT('Ctrl Pts',(-9.28201546219901,-10.3532909943549,
8.33899919343572));
#58411=CARTESIAN_POINT('Ctrl Pts',(-6.28349916850765,-10.0493015205563,
8.18199906608348));
#58412=CARTESIAN_POINT('Ctrl Pts',(-4.37583084109032,-12.3826062838239,
8.02499893873122));
#58413=CARTESIAN_POINT('Ctrl Pts',(-5.26963497019092,-15.2609085157313,
7.86799881137897));
#58414=CARTESIAN_POINT('Ctrl Pts',(-8.16342881906923,-16.1032069936549,
7.71099868402671));
#58415=CARTESIAN_POINT('Ctrl Pts',(-10.4623196804644,-14.1542045895756,
7.55399855667447));
#58416=CARTESIAN_POINT('Ctrl Pts',(-10.1048700666991,-11.1615904606817,
7.3969984293222));
#58417=CARTESIAN_POINT('Ctrl Pts',(-7.41160847115729,-9.80887039960631,
7.23999830196995));
#58418=CARTESIAN_POINT('Ctrl Pts',(-4.79760841334188,-11.3090414752098,
7.08299817461771));
#58419=CARTESIAN_POINT('Ctrl Pts',(-4.60686880545846,-14.3168858672889,
6.92599804726544));
#58420=CARTESIAN_POINT('Ctrl Pts',(-7.01042771746335,-16.1352407018342,
6.7689979199132));
#58421=CARTESIAN_POINT('Ctrl Pts',(-9.85299074832685,-15.133569659674,6.61199779256094));
#58422=CARTESIAN_POINT('Ctrl Pts',(-10.5856044869832,-12.2100809588743,
6.45499766520869));
#58423=CARTESIAN_POINT('Ctrl Pts',(-8.55132691312017,-9.98629460218332,
6.29799753785643));
#58424=CARTESIAN_POINT('Ctrl Pts',(-5.57431473726304,-10.4563018579429,
6.14099741050418));
#58425=CARTESIAN_POINT('Ctrl Pts',(-4.32408237085103,-13.1986413249196,
5.98399728315193));
#58426=CARTESIAN_POINT('Ctrl Pts',(-5.92172706293806,-15.75423360635,5.82699715579966));
#58427=CARTESIAN_POINT('Ctrl Pts',(-8.9346217888498,-15.831449279092,5.66999702844743));
#58428=CARTESIAN_POINT('Ctrl Pts',(-10.6610821880398,-13.3610586938876,
5.51299690109516));
#58429=CARTESIAN_POINT('Ctrl Pts',(-9.55296048110486,-10.558264465972,5.35599677374292));
#58430=CARTESIAN_POINT('Ctrl Pts',(-6.60394777480949,-9.93639883608159,
5.19899664639066));
#58431=CARTESIAN_POINT('Ctrl Pts',(-4.45839776891566,-12.0530168609799,
5.04199651903841));
#58432=CARTESIAN_POINT('Ctrl Pts',(-5.04035196569236,-15.0102791328056,
4.88499639168615));
#58433=CARTESIAN_POINT('Ctrl Pts',(-7.82775858038497,-16.1560822091562,
4.72799626433391));
#58434=CARTESIAN_POINT('Ctrl Pts',(-10.3215301429408,-14.4635566264157,
4.57099613698164));
#58435=CARTESIAN_POINT('Ctrl Pts',(-10.2846816943758,-11.4492649509585,
4.4139960096294));
#58436=CARTESIAN_POINT('Ctrl Pts',(-7.75181407368507,-9.81838740652354,
4.25699588227714));
#58437=CARTESIAN_POINT('Ctrl Pts',(-4.99111687367461,-11.0289452226782,
4.09999575492489));
#58438=CARTESIAN_POINT('Ctrl Pts',(-4.48419585112438,-14.0043237457194,
3.94299562757263));
#58439=CARTESIAN_POINT('Ctrl Pts',(-5.94334031085918,-15.3719748325696,
3.83832887600446));
#58440=CARTESIAN_POINT('Ctrl Pts',(-6.80193357383903,-15.6015132427052,
3.78599550022038));
#58441=CARTESIAN_POINT('Ctrl Pts',(-5.30480289598084,-11.1135176176879,
12.2140044997796));
#58442=CARTESIAN_POINT('Ctrl Pts',(-4.68765210100992,-11.8353429831648,
12.1616711239955));
#58443=CARTESIAN_POINT('Ctrl Pts',(-4.23052912158122,-13.9229055506476,
12.0570043724274));
#58444=CARTESIAN_POINT('Ctrl Pts',(-6.47787345188828,-16.2362251382909,
11.9000042450751));
#58445=CARTESIAN_POINT('Ctrl Pts',(-9.64170211673396,-15.6312537653527,
11.7430041177229));
#58446=CARTESIAN_POINT('Ctrl Pts',(-10.8850307843148,-12.6619854361585,
11.5860039903706));
#58447=CARTESIAN_POINT('Ctrl Pts',(-9.09298218580643,-9.98526441595581,
11.4290038630183));
#58448=CARTESIAN_POINT('Ctrl Pts',(-5.87248446370049,-10.0042444550338,
11.2720037356661));
#58449=CARTESIAN_POINT('Ctrl Pts',(-4.11139900754004,-12.7004190256087,
11.1150036083138));
#58450=CARTESIAN_POINT('Ctrl Pts',(-5.3889027927435,-15.656862268317,10.9580034809616));
#58451=CARTESIAN_POINT('Ctrl Pts',(-8.55944860524813,-16.2221149270002,
10.8010033536093));
#58452=CARTESIAN_POINT('Ctrl Pts',(-10.7799762251851,-13.889507918326,10.6440032262571));
#58453=CARTESIAN_POINT('Ctrl Pts',(-10.0593179346304,-10.7506109382696,
10.4870030989048));
#58454=CARTESIAN_POINT('Ctrl Pts',(-7.04369457784195,-9.62015483331818,
10.3300029715526));
#58455=CARTESIAN_POINT('Ctrl Pts',(-4.43724473266885,-11.5118039609805,
10.1730028442003));
#58456=CARTESIAN_POINT('Ctrl Pts',(-4.57719688678678,-14.7293119312129,
10.0160027168481));
#58457=CARTESIAN_POINT('Ctrl Pts',(-7.33805464880973,-16.3875015653505,
9.85900258949582));
#58458=CARTESIAN_POINT('Ctrl Pts',(-10.2441303526083,-14.9994618439422,
9.70200246214357));
#58459=CARTESIAN_POINT('Ctrl Pts',(-10.6895180474545,-11.8098594957488,
9.5450023347913));
#58460=CARTESIAN_POINT('Ctrl Pts',(-8.2748343081384,-9.6788424688032,9.38800220743907));
#58461=CARTESIAN_POINT('Ctrl Pts',(-5.1653492123935,-10.517313703669,9.2310020800868));
#58462=CARTESIAN_POINT('Ctrl Pts',(-4.14936787495879,-13.5734082410908,
9.07400195273456));
#58463=CARTESIAN_POINT('Ctrl Pts',(-6.137930508842,-16.1066966673671,8.9170018253823));
#58464=CARTESIAN_POINT('Ctrl Pts',(-9.34787392240984,-15.8455550103332,
8.76000169803005));
#58465=CARTESIAN_POINT('Ctrl Pts',(-10.9008110621136,-13.0241514669403,
8.60300157067779));
#58466=CARTESIAN_POINT('Ctrl Pts',(-9.40420829650654,-10.1724656783654,
8.44600144332554));
#58467=CARTESIAN_POINT('Ctrl Pts',(-6.20008368323791,-9.84763164053746,
8.28900131597328));
#58468=CARTESIAN_POINT('Ctrl Pts',(-4.16160650214306,-12.3409311560251,
8.13200118862103));
#58469=CARTESIAN_POINT('Ctrl Pts',(-5.11669879746183,-15.4165986269953,
7.97500106126878));
#58470=CARTESIAN_POINT('Ctrl Pts',(-8.20892014587475,-16.3166535276513,
7.81800093391653));
#58471=CARTESIAN_POINT('Ctrl Pts',(-10.6654459975808,-14.2340079914677,
7.66100080656427));
#58472=CARTESIAN_POINT('Ctrl Pts',(-10.2834860569666,-11.0361902545495,
7.50400067921202));
#58473=CARTESIAN_POINT('Ctrl Pts',(-7.40554746233487,-9.59071415302789,
7.34700055185976));
#58474=CARTESIAN_POINT('Ctrl Pts',(-4.61230537058651,-11.1937519879624,
7.19000042450751));
#58475=CARTESIAN_POINT('Ctrl Pts',(-4.40848674414439,-14.4078443275035,
7.03300029715526));
#58476=CARTESIAN_POINT('Ctrl Pts',(-6.97685773669127,-16.3508837878128,
6.876000169803));
#58477=CARTESIAN_POINT('Ctrl Pts',(-10.0143353689188,-15.280528143144,6.71900004245075));
#58478=CARTESIAN_POINT('Ctrl Pts',(-10.7971844456393,-12.1565757662458,
6.5619999150985));
#58479=CARTESIAN_POINT('Ctrl Pts',(-8.62341641964973,-9.78030433656719,
6.40499978774624));
#58480=CARTESIAN_POINT('Ctrl Pts',(-5.44227046198626,-10.2825399988388,
6.24799966039399));
#58481=CARTESIAN_POINT('Ctrl Pts',(-4.10630963831026,-13.2129217354879,
6.09099953304174));
#58482=CARTESIAN_POINT('Ctrl Pts',(-5.81350485747386,-15.943751028508,5.93399940568949));
#58483=CARTESIAN_POINT('Ctrl Pts',(-9.0329938323351,-16.026261381406,5.77699927833723));
#58484=CARTESIAN_POINT('Ctrl Pts',(-10.8778376541001,-13.3864760665508,
5.61999915098497));
#58485=CARTESIAN_POINT('Ctrl Pts',(-9.69373202053811,-10.3914941848495,
5.46299902363273));
#58486=CARTESIAN_POINT('Ctrl Pts',(-6.54250545659946,-9.72698721683007,
5.30599889628047));
#58487=CARTESIAN_POINT('Ctrl Pts',(-4.24983504578773,-11.9887417801564,
5.14899876892822));
#58488=CARTESIAN_POINT('Ctrl Pts',(-4.87169385296189,-15.1487835824914,
4.99199864157596));
#58489=CARTESIAN_POINT('Ctrl Pts',(-7.85023299250732,-16.3731543976903,
4.83499851422371));
#58490=CARTESIAN_POINT('Ctrl Pts',(-10.5150025187778,-14.5645723033874,
4.67799838687146));
#58491=CARTESIAN_POINT('Ctrl Pts',(-10.4756273713904,-11.3435905901237,
4.5209982595192));
#58492=CARTESIAN_POINT('Ctrl Pts',(-7.76908096953125,-9.60088374129137,
4.36399813216695));
#58493=CARTESIAN_POINT('Ctrl Pts',(-4.81908270974332,-10.8944495300405,
4.2069980048147));
#58494=CARTESIAN_POINT('Ctrl Pts',(-4.27740210298664,-14.0738498152832,
4.04999787746244));
#58495=CARTESIAN_POINT('Ctrl Pts',(-5.83660012621808,-15.5352807633023,
3.94533112589427));
#58496=CARTESIAN_POINT('Ctrl Pts',(-6.75406714565312,-15.7805586266087,
3.89299775011019));
#58497=CARTESIAN_POINT('Ctrl Pts',(-5.1639373423038,-10.993079499836,12.3210067496694));
#58498=CARTESIAN_POINT('Ctrl Pts',(-4.50718404955416,-11.761224318623,12.2686733738853));
#58499=CARTESIAN_POINT('Ctrl Pts',(-4.02072753944713,-13.9827455435609,
12.1640066223172));
#58500=CARTESIAN_POINT('Ctrl Pts',(-6.41228370513427,-16.4445105914997,
12.0070064949649));
#58501=CARTESIAN_POINT('Ctrl Pts',(-9.77913490303484,-15.8007182729381,
11.8500063676127));
#58502=CARTESIAN_POINT('Ctrl Pts',(-11.1022478327399,-12.6409123257588,
11.6930062402604));
#58503=CARTESIAN_POINT('Ctrl Pts',(-9.19520367525283,-9.79242641580684,
11.5360061129082));
#58504=CARTESIAN_POINT('Ctrl Pts',(-5.76804697299906,-9.81262440187857,
11.3790059855559));
#58505=CARTESIAN_POINT('Ctrl Pts',(-3.89395285925593,-12.6818121943635,
11.2220058582037));
#58506=CARTESIAN_POINT('Ctrl Pts',(-5.25343392007517,-15.8279700706855,
11.0650057308514));
#58507=CARTESIAN_POINT('Ctrl Pts',(-8.62743330425189,-16.429494929522,10.9080056034992));
#58508=CARTESIAN_POINT('Ctrl Pts',(-10.9904519342511,-13.9472047888929,
10.7510054761469));
#58509=CARTESIAN_POINT('Ctrl Pts',(-10.2235490814542,-10.6068851392178,
10.5940053487946));
#58510=CARTESIAN_POINT('Ctrl Pts',(-7.01441350972263,-9.40388779191504,
10.4370052214424));
#58511=CARTESIAN_POINT('Ctrl Pts',(-4.2407080682755,-11.4169238334189,10.2800050940901));
#58512=CARTESIAN_POINT('Ctrl Pts',(-4.38964093653616,-14.8408989317544,
10.1230049667379));
#58513=CARTESIAN_POINT('Ctrl Pts',(-7.32766263366035,-16.6054944100355,
9.96600483938563));
#58514=CARTESIAN_POINT('Ctrl Pts',(-10.4202208917104,-15.1283843342959,
9.80900471203338));
#58515=CARTESIAN_POINT('Ctrl Pts',(-10.8941890653303,-11.7341055586577,
9.65200458468112));
#58516=CARTESIAN_POINT('Ctrl Pts',(-8.32455533939524,-9.46634140643289,
9.49500445732887));
#58517=CARTESIAN_POINT('Ctrl Pts',(-5.01553493137219,-10.3586172470561,
9.33800432997662));
#58518=CARTESIAN_POINT('Ctrl Pts',(-3.93435818466818,-13.6108210305748,
9.18100420262436));
#58519=CARTESIAN_POINT('Ctrl Pts',(-6.05052666129351,-16.3066702930228,
9.02400407527212));
#58520=CARTESIAN_POINT('Ctrl Pts',(-9.46645178620579,-16.0287712049414,
8.86700394791984));
#58521=CARTESIAN_POINT('Ctrl Pts',(-11.1190407292075,-13.0263185104,8.71000382056762));
#58522=CARTESIAN_POINT('Ctrl Pts',(-9.52640113081409,-9.99164036237588,
8.55300369321534));
#58523=CARTESIAN_POINT('Ctrl Pts',(-6.11666819796815,-9.64596176051859,
8.3960035658631));
#58524=CARTESIAN_POINT('Ctrl Pts',(-3.94738216319582,-12.2992560282264,
8.23900343851084));
#58525=CARTESIAN_POINT('Ctrl Pts',(-4.96376262473273,-15.5722887382593,
8.0820033111586));
#58526=CARTESIAN_POINT('Ctrl Pts',(-8.25441147268027,-16.5301000616477,
7.92500318380633));
#58527=CARTESIAN_POINT('Ctrl Pts',(-10.8685723146971,-14.3138113933598,
7.76800305645408));
#58528=CARTESIAN_POINT('Ctrl Pts',(-10.4621020472342,-10.9107900484173,
7.61100292910183));
#58529=CARTESIAN_POINT('Ctrl Pts',(-7.39948645351245,-9.37255790644949,
7.45400280174957));
#58530=CARTESIAN_POINT('Ctrl Pts',(-4.42700232783115,-11.078462500715,7.29700267439732));
#58531=CARTESIAN_POINT('Ctrl Pts',(-4.21010468283033,-14.4988027877182,
7.14000254704507));
#58532=CARTESIAN_POINT('Ctrl Pts',(-6.94328775591919,-16.5665268737914,
6.98300241969282));
#58533=CARTESIAN_POINT('Ctrl Pts',(-10.1756799895107,-15.427486626614,6.82600229234056));
#58534=CARTESIAN_POINT('Ctrl Pts',(-11.0087644042953,-12.1030705736173,
6.66900216498831));
#58535=CARTESIAN_POINT('Ctrl Pts',(-8.69550592617927,-9.57431407095109,
6.51200203763606));
#58536=CARTESIAN_POINT('Ctrl Pts',(-5.31022618670948,-10.1087781397346,
6.3550019102838));
#58537=CARTESIAN_POINT('Ctrl Pts',(-3.88853690576949,-13.2272021460562,
6.19800178293155));
#58538=CARTESIAN_POINT('Ctrl Pts',(-5.70528265200966,-16.133268450666,6.0410016555793));
#58539=CARTESIAN_POINT('Ctrl Pts',(-9.13136587582039,-16.22107348372,5.88400152822704));
#58540=CARTESIAN_POINT('Ctrl Pts',(-11.0945931201605,-13.4118934392139,
5.72700140087479));
#58541=CARTESIAN_POINT('Ctrl Pts',(-9.83450355997132,-10.224723903727,5.57000127352253));
#58542=CARTESIAN_POINT('Ctrl Pts',(-6.48106313838945,-9.51757559757857,
5.41300114617028));
#58543=CARTESIAN_POINT('Ctrl Pts',(-4.04127232265978,-11.9244666993329,
5.25600101881803));
#58544=CARTESIAN_POINT('Ctrl Pts',(-4.70303574023142,-15.2872880321773,
5.09900089146577));
#58545=CARTESIAN_POINT('Ctrl Pts',(-7.87270740462966,-16.5902265862243,
4.94200076411352));
#58546=CARTESIAN_POINT('Ctrl Pts',(-10.7084748946149,-14.6655879803591,
4.78500063676127));
#58547=CARTESIAN_POINT('Ctrl Pts',(-10.666573048405,-11.2379162292888,4.62800050940902));
#58548=CARTESIAN_POINT('Ctrl Pts',(-7.78634786537746,-9.38338007605921,
4.47100038205676));
#58549=CARTESIAN_POINT('Ctrl Pts',(-4.64704854581202,-10.7599538374027,
4.31400025470451));
#58550=CARTESIAN_POINT('Ctrl Pts',(-4.0706083548489,-14.143375884847,4.15700012735225));
#58551=CARTESIAN_POINT('Ctrl Pts',(-5.72985994157699,-15.6985866940351,
4.05233337578409));
#58552=CARTESIAN_POINT('Ctrl Pts',(-6.7062007174672,-15.9596040105123,4.));
#58553=CARTESIAN_POINT('Ctrl Pts',(-5.5865340033349,-11.3543938533917,12.));
#58554=CARTESIAN_POINT('Ctrl Pts',(-5.52489675159201,-11.412317734857,12.));
#58555=CARTESIAN_POINT('Ctrl Pts',(-5.46662466733851,-11.4733903391465,
12.));
#58556=CARTESIAN_POINT('Ctrl Pts',(-5.41171731080853,-11.5372273647712,
12.));
#58557=CARTESIAN_POINT('Ctrl Pts',(-5.35535954826471,-11.6027506782036,
12.));
#58558=CARTESIAN_POINT('Ctrl Pts',(-5.30254618320446,-11.6711868211063,
12.));
#58559=CARTESIAN_POINT('Ctrl Pts',(-5.25330217107373,-11.7421687765855,
12.));
#58560=CARTESIAN_POINT('Ctrl Pts',(-5.20312956815832,-11.8144892336791,
12.));
#58561=CARTESIAN_POINT('Ctrl Pts',(-5.1566617252503,-11.8894530177238,12.));
#58562=CARTESIAN_POINT('Ctrl Pts',(-5.11395808422126,-11.9667137220828,
12.));
#58563=CARTESIAN_POINT('Ctrl Pts',(-5.09461562078295,-12.0017086853522,
12.));
#58564=CARTESIAN_POINT('Ctrl Pts',(-5.07604591099636,-12.0371753912937,
12.));
#58565=CARTESIAN_POINT('Ctrl Pts',(-5.05825705836343,-12.0730838611618,
12.));
#58566=CARTESIAN_POINT('Ctrl Pts',(-5.04815218455416,-12.093481498052,12.));
#58567=CARTESIAN_POINT('Ctrl Pts',(-5.03829930483427,-12.1140217037901,
12.));
#58568=CARTESIAN_POINT('Ctrl Pts',(-5.02870015601257,-12.1346991425122,
12.));
#58569=CARTESIAN_POINT('Ctrl Pts',(-5.02048318017586,-12.1523992550431,
12.));
#58570=CARTESIAN_POINT('Ctrl Pts',(-5.01244999988763,-12.1702050672847,
12.));
#58571=CARTESIAN_POINT('Ctrl Pts',(-5.00461448908043,-12.1880835326347,
12.));
#58572=CARTESIAN_POINT('Ctrl Pts',(-4.96800851502513,-12.2716082261557,
12.));
#58573=CARTESIAN_POINT('Ctrl Pts',(-4.93566438777708,-12.3568162975634,
12.));
#58574=CARTESIAN_POINT('Ctrl Pts',(-4.9076092477584,-12.4433098844385,12.));
#58575=CARTESIAN_POINT('Ctrl Pts',(-4.87909470826589,-12.531219793181,12.));
#58576=CARTESIAN_POINT('Ctrl Pts',(-4.85501027288513,-12.6204584164563,
12.));
#58577=CARTESIAN_POINT('Ctrl Pts',(-4.83542346103633,-12.7106451238744,
12.));
#58578=CARTESIAN_POINT('Ctrl Pts',(-4.81671890332471,-12.7967695266993,
12.));
#58579=CARTESIAN_POINT('Ctrl Pts',(-4.80211587003395,-12.8837594508039,
12.));
#58580=CARTESIAN_POINT('Ctrl Pts',(-4.79171175017421,-12.9713041908118,
12.));
#58581=CARTESIAN_POINT('Ctrl Pts',(-4.7871219669274,-13.0099246014234,12.));
#58582=CARTESIAN_POINT('Ctrl Pts',(-4.78334987321312,-13.0486531860177,
12.));
#58583=CARTESIAN_POINT('Ctrl Pts',(-4.78040642509842,-13.0874639619222,
12.));
#58584=CARTESIAN_POINT('Ctrl Pts',(-4.7790340847621,-13.1055589278201,12.));
#58585=CARTESIAN_POINT('Ctrl Pts',(-4.77784189531648,-13.1236717640034,
12.));
#58586=CARTESIAN_POINT('Ctrl Pts',(-4.77683109303951,-13.1417998520234,
12.));
#58587=CARTESIAN_POINT('Ctrl Pts',(-4.7758570840318,-13.1592680764492,12.));
#58588=CARTESIAN_POINT('Ctrl Pts',(-4.77505149943043,-13.1767532882224,
12.));
#58589=CARTESIAN_POINT('Ctrl Pts',(-4.77441609878784,-13.1942285673893,
12.));
#58590=CARTESIAN_POINT('Ctrl Pts',(-4.77095265346117,-13.2894829154418,
12.));
#58591=CARTESIAN_POINT('Ctrl Pts',(-4.77253183089421,-13.3845892743107,
12.));
#58592=CARTESIAN_POINT('Ctrl Pts',(-4.77921580433521,-13.4791489989792,
12.));
#58593=CARTESIAN_POINT('Ctrl Pts',(-4.78586481725455,-13.5732141290278,
12.));
#58594=CARTESIAN_POINT('Ctrl Pts',(-4.79756501411883,-13.6667392834721,
12.));
#58595=CARTESIAN_POINT('Ctrl Pts',(-4.81442558423848,-13.7593498298833,
12.));
#58596=CARTESIAN_POINT('Ctrl Pts',(-4.830924328857,-13.8499729667865,12.));
#58597=CARTESIAN_POINT('Ctrl Pts',(-4.85236399681968,-13.9397212614334,
12.));
#58598=CARTESIAN_POINT('Ctrl Pts',(-4.87847000308199,-14.0283529813775,
12.));
#58599=CARTESIAN_POINT('Ctrl Pts',(-4.89379441408366,-14.0803804301784,
12.));
#58600=CARTESIAN_POINT('Ctrl Pts',(-4.91072775850773,-14.1320231162836,
12.));
#58601=CARTESIAN_POINT('Ctrl Pts',(-4.92922261500886,-14.1832309956159,
12.));
#58602=CARTESIAN_POINT('Ctrl Pts',(-4.93398351814407,-14.1964128093404,
12.));
#58603=CARTESIAN_POINT('Ctrl Pts',(-4.93884875001307,-14.2095679810762,
12.));
#58604=CARTESIAN_POINT('Ctrl Pts',(-4.94381485137731,-14.2226885070165,
12.));
#58605=CARTESIAN_POINT('Ctrl Pts',(-4.97686325186981,-14.310002954335,12.));
#58606=CARTESIAN_POINT('Ctrl Pts',(-5.01429440116268,-14.3955759829307,
12.));
#58607=CARTESIAN_POINT('Ctrl Pts',(-5.05577732713123,-14.4791717978631,
12.));
#58608=CARTESIAN_POINT('Ctrl Pts',(-5.09882663969929,-14.5659241732654,
12.));
#58609=CARTESIAN_POINT('Ctrl Pts',(-5.1462396027634,-14.6505479156747,12.));
#58610=CARTESIAN_POINT('Ctrl Pts',(-5.19770241499811,-14.7327775666312,
12.));
#58611=CARTESIAN_POINT('Ctrl Pts',(-5.24979009521262,-14.8160056604173,
12.));
#58612=CARTESIAN_POINT('Ctrl Pts',(-5.30602696260126,-14.8967819927061,
12.));
#58613=CARTESIAN_POINT('Ctrl Pts',(-5.36613986514052,-14.9748175661494,
12.));
#58614=CARTESIAN_POINT('Ctrl Pts',(-5.40561376259492,-15.0260606120477,
12.));
#58615=CARTESIAN_POINT('Ctrl Pts',(-5.44676008901899,-15.076121523717,12.));
#58616=CARTESIAN_POINT('Ctrl Pts',(-5.48951221838806,-15.1249126475777,
12.));
#58617=CARTESIAN_POINT('Ctrl Pts',(-5.50097170290556,-15.1379908529612,
12.));
#58618=CARTESIAN_POINT('Ctrl Pts',(-5.51254660460158,-15.1509777948558,
12.));
#58619=CARTESIAN_POINT('Ctrl Pts',(-5.52423573327417,-15.1638717111488,
12.));
#58620=CARTESIAN_POINT('Ctrl Pts',(-5.5353884173992,-15.1761738920537,12.));
#58621=CARTESIAN_POINT('Ctrl Pts',(-5.54663940936984,-15.1883850930378,
12.));
#58622=CARTESIAN_POINT('Ctrl Pts',(-5.55798428070717,-15.2005008010861,
12.));
#58623=CARTESIAN_POINT('Ctrl Pts',(-5.62980603833238,-15.2772025477193,
12.));
#58624=CARTESIAN_POINT('Ctrl Pts',(-5.70542358612169,-15.3501207786779,
12.));
#58625=CARTESIAN_POINT('Ctrl Pts',(-5.7844933991545,-15.4189223872958,12.));
#58626=CARTESIAN_POINT('Ctrl Pts',(-5.8437957589291,-15.4705235937591,12.));
#58627=CARTESIAN_POINT('Ctrl Pts',(-5.90504133108183,-15.519808942512,12.));
#58628=CARTESIAN_POINT('Ctrl Pts',(-5.968104244788,-15.5666263507592,12.));
#58629=CARTESIAN_POINT('Ctrl Pts',(-5.99074690383604,-15.5834360817113,
12.));
#58630=CARTESIAN_POINT('Ctrl Pts',(-6.01362398614045,-15.5999275418789,
12.));
#58631=CARTESIAN_POINT('Ctrl Pts',(-6.03673011024537,-15.6160932756601,
12.));
#58632=CARTESIAN_POINT('Ctrl Pts',(-6.05604444624562,-15.6296061613575,
12.));
#58633=CARTESIAN_POINT('Ctrl Pts',(-6.07552135620629,-15.6428929845117,
12.));
#58634=CARTESIAN_POINT('Ctrl Pts',(-6.09513705214722,-15.655935902686,12.));
#58635=CARTESIAN_POINT('Ctrl Pts',(-6.1801078936968,-15.7124349296322,12.));
#58636=CARTESIAN_POINT('Ctrl Pts',(-6.26775546621735,-15.7644144018326,
12.));
#58637=CARTESIAN_POINT('Ctrl Pts',(-6.3577924589883,-15.8115622787044,12.));
#58638=CARTESIAN_POINT('Ctrl Pts',(-6.42986829724945,-15.8493047958986,
12.));
#58639=CARTESIAN_POINT('Ctrl Pts',(-6.50347629812978,-15.8839507974289,
12.));
#58640=CARTESIAN_POINT('Ctrl Pts',(-6.57848586659695,-15.9153228867674,
12.));
#58641=CARTESIAN_POINT('Ctrl Pts',(-6.61998922672564,-15.9326813004793,
12.));
#58642=CARTESIAN_POINT('Ctrl Pts',(-6.66192191928759,-15.9490371078547,
12.));
#58643=CARTESIAN_POINT('Ctrl Pts',(-6.70425049788235,-15.9643995452955,
12.));
#58644=CARTESIAN_POINT('Ctrl Pts',(-10.0166114900998,-12.9925168768863,
10.387416697508));
#58645=CARTESIAN_POINT('Ctrl Pts',(-10.0185038824417,-13.21718192014,10.4016107071645));
#58646=CARTESIAN_POINT('Ctrl Pts',(-9.99083741615502,-13.441388813634,10.415804716821));
#58647=CARTESIAN_POINT('Ctrl Pts',(-9.93173901273922,-13.6569790278497,
10.4299987264775));
#58648=CARTESIAN_POINT('Ctrl Pts',(-9.71384294044885,-14.4518610921136,
10.4823321022616));
#58649=CARTESIAN_POINT('Ctrl Pts',(-9.06866107384475,-15.1296080070351,
10.5346654780456));
#58650=CARTESIAN_POINT('Ctrl Pts',(-8.28546369568261,-15.3863634214331,
10.5869988538297));
#58651=CARTESIAN_POINT('Ctrl Pts',(-7.50226631752047,-15.6431188358311,
10.6393322296138));
#58652=CARTESIAN_POINT('Ctrl Pts',(-6.58105342780029,-15.4788827497055,
10.6916656053979));
#58653=CARTESIAN_POINT('Ctrl Pts',(-5.9348554439449,-14.9672623773959,10.743998981182));
#58654=CARTESIAN_POINT('Ctrl Pts',(-5.2886574600895,-14.4556420050863,10.7963323569661));
#58655=CARTESIAN_POINT('Ctrl Pts',(-4.91747438209889,-13.5966373465927,
10.8486657327501));
#58656=CARTESIAN_POINT('Ctrl Pts',(-4.98772753326943,-12.7754436628867,
10.9009991085342));
#58657=CARTESIAN_POINT('Ctrl Pts',(-5.05798068443997,-11.9542499791808,
10.9533324843183));
#58658=CARTESIAN_POINT('Ctrl Pts',(-5.56967006477166,-11.1708672702625,
11.0056658601024));
#58659=CARTESIAN_POINT('Ctrl Pts',(-6.29337804857255,-10.7764185582883,
11.0579992358865));
#58660=CARTESIAN_POINT('Ctrl Pts',(-7.01708603237344,-10.3819698463141,
11.1103326116706));
#58661=CARTESIAN_POINT('Ctrl Pts',(-7.95281261964353,-10.3764551312839,
11.1626659874547));
#58662=CARTESIAN_POINT('Ctrl Pts',(-8.68101882670376,-10.7625629805529,
11.2149993632387));
#58663=CARTESIAN_POINT('Ctrl Pts',(-9.40922503376398,-11.1486708298218,
11.2673327390228));
#58664=CARTESIAN_POINT('Ctrl Pts',(-9.92991086061434,-11.9264012433898,
11.3196661148069));
#58665=CARTESIAN_POINT('Ctrl Pts',(-10.0096270834841,-12.7466319657112,
11.371999490591));
#58666=CARTESIAN_POINT('Ctrl Pts',(-10.0174551121829,-12.8271775485652,
11.3771385595633));
#58667=CARTESIAN_POINT('Ctrl Pts',(-10.0210308785667,-12.9081329611663,
11.3822776285357));
#58668=CARTESIAN_POINT('Ctrl Pts',(-10.0205077525331,-12.989132710429,11.387416697508));
#58669=CARTESIAN_POINT('Ctrl Pts',(-8.29379928253297,-15.9596040105122,
12.));
#58670=CARTESIAN_POINT('Ctrl Pts',(-9.27014005842316,-15.698586694035,11.9476666242159));
#58671=CARTESIAN_POINT('Ctrl Pts',(-10.9293914260692,-14.1433745388278,
11.8429998726477));
#58672=CARTESIAN_POINT('Ctrl Pts',(-10.3529516457367,-10.7599545073216,
11.6859997452955));
#58673=CARTESIAN_POINT('Ctrl Pts',(-7.21365210721562,-9.38337955935061,
11.5289996179432));
#58674=CARTESIAN_POINT('Ctrl Pts',(-4.33342685529555,-11.2379164301912,
11.371999490591));
#58675=CARTESIAN_POINT('Ctrl Pts',(-4.29152503935676,-14.6655878811314,
11.2149993632387));
#58676=CARTESIAN_POINT('Ctrl Pts',(-7.12729256983938,-16.5902267633183,
11.0579992358865));
#58677=CARTESIAN_POINT('Ctrl Pts',(-10.296964344732,-15.2872880462285,10.9009991085342));
#58678=CARTESIAN_POINT('Ctrl Pts',(-10.9587277612158,-11.9244666973206,
10.743998981182));
#58679=CARTESIAN_POINT('Ctrl Pts',(-8.51893689306524,-9.51757549146244,
10.5869988538297));
#58680=CARTESIAN_POINT('Ctrl Pts',(-5.16549637569413,-10.2247238388162,
10.4299987264775));
#58681=CARTESIAN_POINT('Ctrl Pts',(-3.90540678666615,-13.4118934459175,
10.2729985991252));
#58682=CARTESIAN_POINT('Ctrl Pts',(-5.86863408021139,-16.2210735713392,
10.115998471773));
#58683=CARTESIAN_POINT('Ctrl Pts',(-9.29471739586239,-16.133268532241,9.9589983444207));
#58684=CARTESIAN_POINT('Ctrl Pts',(-11.1114631891741,-13.227202153015,9.80199821706844));
#58685=CARTESIAN_POINT('Ctrl Pts',(-9.68977387121298,-10.1087780633504,
9.64499808971621));
#58686=CARTESIAN_POINT('Ctrl Pts',(-6.30449404219616,-9.57431398106461,
9.48799796236394));
#58687=CARTESIAN_POINT('Ctrl Pts',(-3.99123550321764,-12.1030705501041,
9.33099783501171));
#58688=CARTESIAN_POINT('Ctrl Pts',(-4.82431993989319,-15.4274866909495,
9.17399770765942));
#58689=CARTESIAN_POINT('Ctrl Pts',(-8.05671225877921,-16.5665269680756,
9.0169975803072));
#58690=CARTESIAN_POINT('Ctrl Pts',(-10.789895403928,-14.4988028275178,8.85999745295491));
#58691=CARTESIAN_POINT('Ctrl Pts',(-10.5729977532197,-11.0784624502813,
8.70299732560269));
#58692=CARTESIAN_POINT('Ctrl Pts',(-7.60051354913579,-9.37255781103892,
8.54599719825042));
#58693=CARTESIAN_POINT('Ctrl Pts',(-4.53789787464541,-10.9107899935683,
8.38899707089818));
#58694=CARTESIAN_POINT('Ctrl Pts',(-4.13142759646044,-14.3138114282651,
8.23199694354591));
#58695=CARTESIAN_POINT('Ctrl Pts',(-6.74558850742372,-16.5301001550025,
8.07499681619368));
#58696=CARTESIAN_POINT('Ctrl Pts',(-10.0362374421571,-15.5722888063543,
7.9179966888414));
#58697=CARTESIAN_POINT('Ctrl Pts',(-11.0526179305001,-12.2992560099981,
7.76099656148917));
#58698=CARTESIAN_POINT('Ctrl Pts',(-8.88333183851511,-9.64596167231467,
7.60399643413689));
#58699=CARTESIAN_POINT('Ctrl Pts',(-5.47359881574229,-9.99164028328652,
7.44699630678467));
#58700=CARTESIAN_POINT('Ctrl Pts',(-3.88095917534459,-13.0263185113509,
7.28999617943238));
#58701=CARTESIAN_POINT('Ctrl Pts',(-5.53354816193247,-16.0287712850697,
7.13299605208016));
#58702=CARTESIAN_POINT('Ctrl Pts',(-8.94947337693327,-16.3066703804957,
6.97599592472788));
#58703=CARTESIAN_POINT('Ctrl Pts',(-11.0656419093738,-13.610821046919,6.81899579737565));
#58704=CARTESIAN_POINT('Ctrl Pts',(-9.98446513414696,-10.3586171776818,
6.66199567002337));
#58705=CARTESIAN_POINT('Ctrl Pts',(-6.67544463886838,-9.46634131342536,
6.50499554267114));
#58706=CARTESIAN_POINT('Ctrl Pts',(-4.10581084513197,-11.7341055256468,
6.34799541531887));
#58707=CARTESIAN_POINT('Ctrl Pts',(-4.57977903131249,-15.1283843904584,
6.19099528796663));
#58708=CARTESIAN_POINT('Ctrl Pts',(-7.67233737080682,-16.6054945057935,
6.03399516061437));
#58709=CARTESIAN_POINT('Ctrl Pts',(-10.610359145649,-14.8408989797994,5.87699503326212));
#58710=CARTESIAN_POINT('Ctrl Pts',(-10.7592920173832,-11.4169237933092,
5.71999490590986));
#58711=CARTESIAN_POINT('Ctrl Pts',(-7.98558650367391,-9.40388769480238,
5.56299477855761));
#58712=CARTESIAN_POINT('Ctrl Pts',(-4.77645084555843,-10.6068850809164,
5.40599465120535));
#58713=CARTESIAN_POINT('Ctrl Pts',(-4.00954797596254,-13.9472048059447,
5.24899452385311));
#58714=CARTESIAN_POINT('Ctrl Pts',(-6.37256666156175,-16.4294950347898,
5.09199439650084));
#58715=CARTESIAN_POINT('Ctrl Pts',(-9.74656614790733,-15.8279701198543,
4.9349942691486));
#58716=CARTESIAN_POINT('Ctrl Pts',(-11.1060472187217,-12.6818122309103,
4.77799414179634));
#58717=CARTESIAN_POINT('Ctrl Pts',(-9.23195310627391,-9.81262424147309,
4.62099401444409));
#58718=CARTESIAN_POINT('Ctrl Pts',(-5.80479621412607,-9.79242646017958,
4.46399388709183));
#58719=CARTESIAN_POINT('Ctrl Pts',(-3.89775220169895,-12.6409121056472,
4.30699375973959));
#58720=CARTESIAN_POINT('Ctrl Pts',(-5.22086478169416,-15.8007186832344,
4.14999363238732));
#58721=CARTESIAN_POINT('Ctrl Pts',(-8.58771683219162,-16.4445101479194,
3.99299350503508));
#58722=CARTESIAN_POINT('Ctrl Pts',(-10.979271517566,-13.9827465287205,3.83599337768283));
#58723=CARTESIAN_POINT('Ctrl Pts',(-10.4928159504458,-11.7612243186229,
3.73132662611465));
#58724=CARTESIAN_POINT('Ctrl Pts',(-9.83606265769611,-10.9930794998359,
3.67899325033057));
#58725=CARTESIAN_POINT('Ctrl Pts',(-8.24593285434704,-15.7805586266087,
12.1070022498898));
#58726=CARTESIAN_POINT('Ctrl Pts',(-9.16339987378206,-15.5352807633023,
12.0546688741057));
#58727=CARTESIAN_POINT('Ctrl Pts',(-10.7225976911422,-14.0738485504296,
11.9500021225376));
#58728=CARTESIAN_POINT('Ctrl Pts',(-10.180917470255,-10.8944501595629,11.7930019951853));
#58729=CARTESIAN_POINT('Ctrl Pts',(-7.23091900471447,-9.60088325574055,
11.6360018678331));
#58730=CARTESIAN_POINT('Ctrl Pts',(-4.52437253811706,-11.3435907789116,
11.4790017404808));
#58731=CARTESIAN_POINT('Ctrl Pts',(-4.48499741917537,-14.5645722101431,
11.3220016131286));
#58732=CARTESIAN_POINT('Ctrl Pts',(-7.14976698350127,-16.3731545641054,
11.1650014857763));
#58733=CARTESIAN_POINT('Ctrl Pts',(-10.1283062268782,-15.1487835956953,
11.008001358424));
#58734=CARTESIAN_POINT('Ctrl Pts',(-10.7501650330301,-11.9887417782655,
10.8510012310718));
#58735=CARTESIAN_POINT('Ctrl Pts',(-8.45749457295849,-9.72698711711278,
10.6940011037196));
#58736=CARTESIAN_POINT('Ctrl Pts',(-5.30626791900676,-10.3914941238528,
10.5370009763673));
#58737=CARTESIAN_POINT('Ctrl Pts',(-4.12216225834487,-13.3864760728501,
10.380000849015));
#58738=CARTESIAN_POINT('Ctrl Pts',(-5.96700612634799,-16.0262614637418,
10.2230007216628));
#58739=CARTESIAN_POINT('Ctrl Pts',(-9.18649518751149,-15.9437511051639,
10.0660005943105));
#58740=CARTESIAN_POINT('Ctrl Pts',(-10.8936904509082,-13.2129217420271,
9.90900046695826));
#58741=CARTESIAN_POINT('Ctrl Pts',(-9.55772959244346,-10.2825399270605,
9.75200033960601));
#58742=CARTESIAN_POINT('Ctrl Pts',(-6.37658355063268,-9.78030425210093,
9.59500021225375));
#58743=CARTESIAN_POINT('Ctrl Pts',(-4.20281546745071,-12.1565757441505,
9.43800008490151));
#58744=CARTESIAN_POINT('Ctrl Pts',(-4.9856645647421,-15.2805282036001,9.28099995754924));
#58745=CARTESIAN_POINT('Ctrl Pts',(-8.02314227712081,-16.3508838764116,
9.12399983019701));
#58746=CARTESIAN_POINT('Ctrl Pts',(-10.5915133373824,-14.4078443649032,
8.96699970284473));
#58747=CARTESIAN_POINT('Ctrl Pts',(-10.387694705577,-11.1937519405699,8.8099995754925));
#58748=CARTESIAN_POINT('Ctrl Pts',(-7.59445254015368,-9.59071406337065,
8.65299944814022));
#58749=CARTESIAN_POINT('Ctrl Pts',(-4.71651386962368,-11.0361902030079,
8.49599932078799));
#58750=CARTESIAN_POINT('Ctrl Pts',(-4.33455391893407,-14.2340080242683,
8.33899919343572));
#58751=CARTESIAN_POINT('Ctrl Pts',(-6.79107983542896,-16.3166536153767,
8.18199906608348));
#58752=CARTESIAN_POINT('Ctrl Pts',(-9.88330126539458,-15.4165986909841,
8.02499893873122));
#58753=CARTESIAN_POINT('Ctrl Pts',(-10.8383935859029,-12.340931138896,7.86799881137898));
#58754=CARTESIAN_POINT('Ctrl Pts',(-8.79991635104542,-9.84763155765228,
7.7109986840267));
#58755=CARTESIAN_POINT('Ctrl Pts',(-5.59579165327249,-10.1724656040451,
7.55399855667448));
#58756=CARTESIAN_POINT('Ctrl Pts',(-4.09918884819405,-13.0241514678338,
7.3969984293222));
#58757=CARTESIAN_POINT('Ctrl Pts',(-5.65212602885569,-15.8455550856297,
7.23999830196996));
#58758=CARTESIAN_POINT('Ctrl Pts',(-8.8620695270797,-16.1066967495653,7.0829981746177));
#58759=CARTESIAN_POINT('Ctrl Pts',(-10.8506322134124,-13.5734082564495,
6.92599804726545));
#58760=CARTESIAN_POINT('Ctrl Pts',(-9.83465084917482,-10.517313638478,6.76899791991319));
#58761=CARTESIAN_POINT('Ctrl Pts',(-6.72516567143593,-9.67884238140407,
6.61199779256095));
#58762=CARTESIAN_POINT('Ctrl Pts',(-4.31048186840692,-11.8098594647285,
6.45499766520868));
#58763=CARTESIAN_POINT('Ctrl Pts',(-4.75586957505634,-14.999461896718,6.29799753785644));
#58764=CARTESIAN_POINT('Ctrl Pts',(-7.66194535538809,-16.3875016553343,
6.14099741050417));
#58765=CARTESIAN_POINT('Ctrl Pts',(-10.4228031904426,-14.7293119763608,
5.98399728315194));
#58766=CARTESIAN_POINT('Ctrl Pts',(-10.5627553478246,-11.5118039232893,
5.82699715579966));
#58767=CARTESIAN_POINT('Ctrl Pts',(-7.95630543474677,-9.62015474206144,
5.66999702844743));
#58768=CARTESIAN_POINT('Ctrl Pts',(-4.94068199678335,-10.7506108834838,
5.51299690109516));
#58769=CARTESIAN_POINT('Ctrl Pts',(-4.22002369044277,-13.8895079343495,
5.35599677374291));
#58770=CARTESIAN_POINT('Ctrl Pts',(-6.44055136262695,-16.2221150259203,
5.19899664639066));
#58771=CARTESIAN_POINT('Ctrl Pts',(-9.61109727113964,-15.6568623145209,
5.04199651903841));
#58772=CARTESIAN_POINT('Ctrl Pts',(-10.8886010657355,-12.7004190599517,
4.88499639168614));
#58773=CARTESIAN_POINT('Ctrl Pts',(-9.12751561079228,-10.0042443043008,
4.72799626433391));
#58774=CARTESIAN_POINT('Ctrl Pts',(-5.90701771024297,-9.98526445765287,
4.57099613698164));
#58775=CARTESIAN_POINT('Ctrl Pts',(-4.11496924804734,-12.6619852293197,
4.4139960096294));
#58776=CARTESIAN_POINT('Ctrl Pts',(-5.35829758700603,-15.631254150908,4.25699588227714));
#58777=CARTESIAN_POINT('Ctrl Pts',(-8.52212705303664,-16.2362247214587,
4.09999575492489));
#58778=CARTESIAN_POINT('Ctrl Pts',(-10.7694699922944,-13.9229064764016,
3.94299562757263));
#58779=CARTESIAN_POINT('Ctrl Pts',(-10.31234789899,-11.8353429831647,3.83832887600446));
#58780=CARTESIAN_POINT('Ctrl Pts',(-9.69519710401908,-11.1135176176878,
3.78599550022038));
#58781=CARTESIAN_POINT('Ctrl Pts',(-8.19806642616111,-15.6015132427052,
12.2140044997796));
#58782=CARTESIAN_POINT('Ctrl Pts',(-9.05665968914096,-15.3719748325695,
12.1616711239955));
#58783=CARTESIAN_POINT('Ctrl Pts',(-10.5158039562152,-14.0043225620313,
12.0570043724274));
#58784=CARTESIAN_POINT('Ctrl Pts',(-10.0088832947732,-11.0289458118043,
11.9000042450751));
#58785=CARTESIAN_POINT('Ctrl Pts',(-7.24818590221332,-9.81838695213045,
11.7430041177229));
#58786=CARTESIAN_POINT('Ctrl Pts',(-4.71531822093855,-11.4492651276319,
11.5860039903706));
#58787=CARTESIAN_POINT('Ctrl Pts',(-4.67846979899401,-14.4635565391549,
11.4290038630183));
#58788=CARTESIAN_POINT('Ctrl Pts',(-7.17224139716313,-16.1560823648925,
11.2720037356661));
#58789=CARTESIAN_POINT('Ctrl Pts',(-9.95964810902439,-15.0102791451622,
11.1150036083138));
#58790=CARTESIAN_POINT('Ctrl Pts',(-10.5416023048445,-12.0530168592103,
10.9580034809616));
#58791=CARTESIAN_POINT('Ctrl Pts',(-8.39605225285175,-9.93639874276315,
10.8010033536093));
#58792=CARTESIAN_POINT('Ctrl Pts',(-5.44703946231937,-10.5582644088895,
10.6440032262571));
#58793=CARTESIAN_POINT('Ctrl Pts',(-4.3389177300236,-13.3610586997827,10.4870030989048));
#58794=CARTESIAN_POINT('Ctrl Pts',(-6.06537817248458,-15.8314493561443,
10.3300029715526));
#58795=CARTESIAN_POINT('Ctrl Pts',(-9.07827297916059,-15.7542336780869,
10.1730028442003));
#58796=CARTESIAN_POINT('Ctrl Pts',(-10.6759177126423,-13.1986413310391,
10.0160027168481));
#58797=CARTESIAN_POINT('Ctrl Pts',(-9.42568531367393,-10.4563017907707,
9.85900258949582));
#58798=CARTESIAN_POINT('Ctrl Pts',(-6.44867305906919,-9.98629452313723,
9.70200246214357));
#58799=CARTESIAN_POINT('Ctrl Pts',(-4.41439543168378,-12.2100809381968,
9.54500233479132));
#58800=CARTESIAN_POINT('Ctrl Pts',(-5.14700918959101,-15.1335697162506,
9.38800220743905));
#58801=CARTESIAN_POINT('Ctrl Pts',(-7.98957229546242,-16.1352407847476,
9.23100208008682));
#58802=CARTESIAN_POINT('Ctrl Pts',(-10.3931312708367,-14.3168859022886,
9.07400195273454));
#58803=CARTESIAN_POINT('Ctrl Pts',(-10.2023916579342,-11.3090414308585,
8.91700182538231));
#58804=CARTESIAN_POINT('Ctrl Pts',(-7.58839153117158,-9.80887031570234,
8.76000169803004));
#58805=CARTESIAN_POINT('Ctrl Pts',(-4.89512986460196,-11.1615904124476,
8.6030015706778));
#58806=CARTESIAN_POINT('Ctrl Pts',(-4.53768024140768,-14.1542046202714,
8.44600144332553));
#58807=CARTESIAN_POINT('Ctrl Pts',(-6.83657116343421,-16.103207075751,8.28900131597329));
#58808=CARTESIAN_POINT('Ctrl Pts',(-9.730365088632,-15.2609085756139,8.13200118862103));
#58809=CARTESIAN_POINT('Ctrl Pts',(-10.6241692413057,-12.3826062677939,
7.97500106126879));
#58810=CARTESIAN_POINT('Ctrl Pts',(-8.71650086357571,-10.0493014429898,
7.81800093391652));
#58811=CARTESIAN_POINT('Ctrl Pts',(-5.7179844908027,-10.3532909248038,7.66100080656428));
#58812=CARTESIAN_POINT('Ctrl Pts',(-4.31741852104351,-13.0219844243168,
7.50400067921201));
#58813=CARTESIAN_POINT('Ctrl Pts',(-5.7707038957789,-15.6623388861897,7.34700055185977));
#58814=CARTESIAN_POINT('Ctrl Pts',(-8.77466567722613,-15.9067231186349,
7.19000042450751));
#58815=CARTESIAN_POINT('Ctrl Pts',(-10.635622517451,-13.5359954659799,7.03300029715527));
#58816=CARTESIAN_POINT('Ctrl Pts',(-9.68483656420267,-10.6760100992742,
6.87600016980299));
#58817=CARTESIAN_POINT('Ctrl Pts',(-6.77488670400349,-9.89134344938279,
6.71900004245076));
#58818=CARTESIAN_POINT('Ctrl Pts',(-4.51515289168187,-11.8856134038101,
6.56199991509849));
#58819=CARTESIAN_POINT('Ctrl Pts',(-4.93196011880019,-14.8705394029777,
6.40499978774625));
#58820=CARTESIAN_POINT('Ctrl Pts',(-7.65155333996934,-16.1695088048751,
6.24799966039398));
#58821=CARTESIAN_POINT('Ctrl Pts',(-10.2352472352362,-14.6177249729221,
6.09099953304175));
#58822=CARTESIAN_POINT('Ctrl Pts',(-10.366218678266,-11.6066840532695,5.93399940568948));
#58823=CARTESIAN_POINT('Ctrl Pts',(-7.92702436581964,-9.83642178932047,
5.77699927833724));
#58824=CARTESIAN_POINT('Ctrl Pts',(-5.10491314800829,-10.8943366860512,
5.61999915098497));
#58825=CARTESIAN_POINT('Ctrl Pts',(-4.43049940492298,-13.8318110627544,
5.46299902363273));
#58826=CARTESIAN_POINT('Ctrl Pts',(-6.50853606369215,-16.0147350170509,
5.30599889628046));
#58827=CARTESIAN_POINT('Ctrl Pts',(-9.47562839437195,-15.4857545091874,
5.14899876892823));
#58828=CARTESIAN_POINT('Ctrl Pts',(-10.6711549127493,-12.7190258889931,
4.99199864157595));
#58829=CARTESIAN_POINT('Ctrl Pts',(-9.02307811531067,-10.1958643671286,
4.83499851422372));
#58830=CARTESIAN_POINT('Ctrl Pts',(-6.00923920635987,-10.1781024551261,
4.67799838687145));
#58831=CARTESIAN_POINT('Ctrl Pts',(-4.33218629439574,-12.6830583529922,
4.52099825951921));
#58832=CARTESIAN_POINT('Ctrl Pts',(-5.49573039231789,-15.4617896185815,
4.36399813216695));
#58833=CARTESIAN_POINT('Ctrl Pts',(-8.45653727388165,-16.027939294998,4.2069980048147));
#58834=CARTESIAN_POINT('Ctrl Pts',(-10.5596684670228,-13.8630664240827,
4.04999787746245));
#58835=CARTESIAN_POINT('Ctrl Pts',(-10.1318798475343,-11.9094616477065,
3.94533112589428));
#58836=CARTESIAN_POINT('Ctrl Pts',(-9.55433155034205,-11.2339557355397,
3.89299775011019));
#58837=CARTESIAN_POINT('Ctrl Pts',(-8.15019999797519,-15.4224678588016,
12.3210067496694));
#58838=CARTESIAN_POINT('Ctrl Pts',(-8.94991950449986,-15.2086689018368,
12.2686733738853));
#58839=CARTESIAN_POINT('Ctrl Pts',(-10.3090102212882,-13.934796573633,12.1640066223172));
#58840=CARTESIAN_POINT('Ctrl Pts',(-9.83684911929144,-11.1634414640457,
12.0070064949649));
#58841=CARTESIAN_POINT('Ctrl Pts',(-7.26545279971217,-10.0358906485204,
11.8500063676127));
#58842=CARTESIAN_POINT('Ctrl Pts',(-4.90626390376006,-11.5549394763523,
11.6930062402604));
#58843=CARTESIAN_POINT('Ctrl Pts',(-4.87194217881263,-14.3625408681667,
11.5360061129082));
#58844=CARTESIAN_POINT('Ctrl Pts',(-7.19471581082501,-15.9390101656796,
11.3790059855559));
#58845=CARTESIAN_POINT('Ctrl Pts',(-9.7909899911706,-14.871774694629,11.2220058582037));
#58846=CARTESIAN_POINT('Ctrl Pts',(-10.3330395766588,-12.1172919401552,
11.0650057308514));
#58847=CARTESIAN_POINT('Ctrl Pts',(-8.334609932745,-10.1458103684135,10.9080056034992));
#58848=CARTESIAN_POINT('Ctrl Pts',(-5.587811005632,-10.7250346939262,10.7510054761469));
#58849=CARTESIAN_POINT('Ctrl Pts',(-4.55567320170231,-13.3356413267153,
10.5940053487946));
#58850=CARTESIAN_POINT('Ctrl Pts',(-6.16375021862117,-15.6366372485469,
10.4370052214424));
#58851=CARTESIAN_POINT('Ctrl Pts',(-8.97005077080969,-15.5647162510099,
10.2800050940901));
#58852=CARTESIAN_POINT('Ctrl Pts',(-10.4581449743764,-13.1843609200512,
10.1230049667379));
#58853=CARTESIAN_POINT('Ctrl Pts',(-9.29364103490441,-10.6300636544808,
9.96600483938564));
#58854=CARTESIAN_POINT('Ctrl Pts',(-6.52076256750571,-10.1922847941736,
9.80900471203337));
#58855=CARTESIAN_POINT('Ctrl Pts',(-4.62597539591685,-12.2635861322432,
9.65200458468114));
#58856=CARTESIAN_POINT('Ctrl Pts',(-5.30835381443992,-14.9866112289011,
9.49500445732886));
#58857=CARTESIAN_POINT('Ctrl Pts',(-7.95600231380402,-15.9195976930836,
9.33800432997663));
#58858=CARTESIAN_POINT('Ctrl Pts',(-10.1947492042911,-14.2259274396741,
9.18100420262435));
#58859=CARTESIAN_POINT('Ctrl Pts',(-10.0170886102914,-11.424330921147,9.02400407527213));
#58860=CARTESIAN_POINT('Ctrl Pts',(-7.58233052218947,-10.0270265680341,
8.86700394791983));
#58861=CARTESIAN_POINT('Ctrl Pts',(-5.07374585958023,-11.2869906218872,
8.71000382056763));
#58862=CARTESIAN_POINT('Ctrl Pts',(-4.7408065638813,-14.0744012162745,8.55300369321533));
#58863=CARTESIAN_POINT('Ctrl Pts',(-6.88206249143947,-15.8897605361253,
8.39600356586311));
#58864=CARTESIAN_POINT('Ctrl Pts',(-9.57742891186941,-15.1052184602437,
8.23900343851083));
#58865=CARTESIAN_POINT('Ctrl Pts',(-10.4099448967086,-12.4242813966918,
8.0820033111586));
#58866=CARTESIAN_POINT('Ctrl Pts',(-8.633085376106,-10.2509713283274,7.92500318380633));
#58867=CARTESIAN_POINT('Ctrl Pts',(-5.84017732833291,-10.5341162455624,
7.7680030564541));
#58868=CARTESIAN_POINT('Ctrl Pts',(-4.53564819389297,-13.0198173807997,
7.61100292910182));
#58869=CARTESIAN_POINT('Ctrl Pts',(-5.88928176270212,-15.4791226867497,
7.45400280174959));
#58870=CARTESIAN_POINT('Ctrl Pts',(-8.68726182737255,-15.7067494877046,
7.29700267439731));
#58871=CARTESIAN_POINT('Ctrl Pts',(-10.4206128214897,-13.4985826755103,
7.14000254704508));
#58872=CARTESIAN_POINT('Ctrl Pts',(-9.53502227923051,-10.8347065600703,
6.9830024196928));
#58873=CARTESIAN_POINT('Ctrl Pts',(-6.82460773657105,-10.1038445173615,
6.82600229234058));
#58874=CARTESIAN_POINT('Ctrl Pts',(-4.71982391495681,-11.9613673428918,
6.66900216498829));
#58875=CARTESIAN_POINT('Ctrl Pts',(-5.10805066254405,-14.7416169092374,
6.51200203763607));
#58876=CARTESIAN_POINT('Ctrl Pts',(-7.64116132455058,-15.9515159544159,
6.35500191028379));
#58877=CARTESIAN_POINT('Ctrl Pts',(-10.0476912800297,-14.5061379694834,
6.19800178293156));
#58878=CARTESIAN_POINT('Ctrl Pts',(-10.1696820087074,-11.7015641832497,
6.04100165557928));
#58879=CARTESIAN_POINT('Ctrl Pts',(-7.8977432968925,-10.0526888365795,5.88400152822706));
#58880=CARTESIAN_POINT('Ctrl Pts',(-5.26914429923322,-11.0380624886186,
5.72700140087478));
#58881=CARTESIAN_POINT('Ctrl Pts',(-4.6409751194032,-13.7741141911592,5.57000127352254));
#58882=CARTESIAN_POINT('Ctrl Pts',(-6.57652076475734,-15.8073550081814,
5.41300114617028));
#58883=CARTESIAN_POINT('Ctrl Pts',(-9.34015951760427,-15.314646703854,5.25600101881803));
#58884=CARTESIAN_POINT('Ctrl Pts',(-10.4537087597631,-12.7376327180345,
5.09900089146577));
#58885=CARTESIAN_POINT('Ctrl Pts',(-8.91864061982905,-10.3874844299563,
4.94200076411353));
#58886=CARTESIAN_POINT('Ctrl Pts',(-6.11146070247677,-10.3709404525994,
4.78500063676126));
#58887=CARTESIAN_POINT('Ctrl Pts',(-4.54940334074414,-12.7041314766647,
4.62800050940902));
#58888=CARTESIAN_POINT('Ctrl Pts',(-5.63316319762975,-15.2923250862551,
4.47100038205676));
#58889=CARTESIAN_POINT('Ctrl Pts',(-8.39094749472666,-15.8196538685372,
4.31400025470451));
#58890=CARTESIAN_POINT('Ctrl Pts',(-10.3498669417512,-13.8032263717638,
4.15700012735226));
#58891=CARTESIAN_POINT('Ctrl Pts',(-9.95141179607851,-11.9835803122483,
4.05233337578409));
#58892=CARTESIAN_POINT('Ctrl Pts',(-9.41346599666503,-11.3543938533916,
4.));
#58893=CARTESIAN_POINT('Ctrl Pts',(-10.0159021674261,-12.9883695445715,
11.112583302492));
#58894=CARTESIAN_POINT('Ctrl Pts',(-10.0178571377502,-12.737164469747,11.0967241119451));
#58895=CARTESIAN_POINT('Ctrl Pts',(-9.98318366513377,-12.4864861117061,
11.0808649213983));
#58896=CARTESIAN_POINT('Ctrl Pts',(-9.90962637175846,-12.2477921372772,
11.0650057308514));
#58897=CARTESIAN_POINT('Ctrl Pts',(-9.66689636202086,-11.4601314162413,
11.0126723550673));
#58898=CARTESIAN_POINT('Ctrl Pts',(-9.00075314738293,-10.8029708923274,
10.9603389792832));
#58899=CARTESIAN_POINT('Ctrl Pts',(-8.20988171887847,-10.5709280179559,
10.9080056034991));
#58900=CARTESIAN_POINT('Ctrl Pts',(-7.419010290374,-10.3388851435844,10.8556722277151));
#58901=CARTESIAN_POINT('Ctrl Pts',(-6.503410648003,-10.5319599187553,10.803338851931));
#58902=CARTESIAN_POINT('Ctrl Pts',(-5.87358785949589,-11.0635984118056,
10.7510054761469));
#58903=CARTESIAN_POINT('Ctrl Pts',(-5.24376507098877,-11.5952369048559,
10.6986721003628));
#58904=CARTESIAN_POINT('Ctrl Pts',(-4.89971913634554,-12.4654391157856,
10.6463387245787));
#58905=CARTESIAN_POINT('Ctrl Pts',(-4.99570900517707,-13.2840395415557,
10.5940053487946));
#58906=CARTESIAN_POINT('Ctrl Pts',(-5.0916988740086,-14.1026399673258,10.5416719730106));
#58907=CARTESIAN_POINT('Ctrl Pts',(-5.62772454631489,-14.8696386079364,
10.4893385972265));
#58908=CARTESIAN_POINT('Ctrl Pts',(-6.36345414116612,-15.2411510953188,
10.4370052214424));
#58909=CARTESIAN_POINT('Ctrl Pts',(-7.09918373601734,-15.6126635827012,
10.3846718456583));
#58910=CARTESIAN_POINT('Ctrl Pts',(-8.03461725341351,-15.5886899168556,
10.3323384698742));
#58911=CARTESIAN_POINT('Ctrl Pts',(-8.75034971270605,-15.1799771954396,
10.2800050940901));
#58912=CARTESIAN_POINT('Ctrl Pts',(-9.46608217199859,-14.7712644740237,
10.2276717183061));
#58913=CARTESIAN_POINT('Ctrl Pts',(-9.96211357318751,-13.9778126970374,
10.175338342522));
#58914=CARTESIAN_POINT('Ctrl Pts',(-10.01604528387,-13.1553705976159,10.1230049667379));
#58915=CARTESIAN_POINT('Ctrl Pts',(-10.0196252693796,-13.1007769130985,
10.1195310786559));
#58916=CARTESIAN_POINT('Ctrl Pts',(-10.0212572306508,-13.0460554884989,
10.1160571905739));
#58917=CARTESIAN_POINT('Ctrl Pts',(-10.0209920718673,-12.9913179799917,
10.112583302492));
#58918=CARTESIAN_POINT('Ctrl Pts',(-8.29379928253297,-15.9596040105122,
12.));
#58919=CARTESIAN_POINT('Ctrl Pts',(-8.38688146826619,-15.9255541311756,
12.));
#58920=CARTESIAN_POINT('Ctrl Pts',(-8.47790052796864,-15.8867414890058,
12.));
#58921=CARTESIAN_POINT('Ctrl Pts',(-8.56664663605253,-15.843492548424,12.));
#58922=CARTESIAN_POINT('Ctrl Pts',(-8.65733876929825,-15.7992952448277,
12.));
#58923=CARTESIAN_POINT('Ctrl Pts',(-8.74565784480789,-15.750464336337,12.));
#58924=CARTESIAN_POINT('Ctrl Pts',(-8.83135101694567,-15.6973027457218,
12.));
#58925=CARTESIAN_POINT('Ctrl Pts',(-8.91318960012018,-15.6465324317433,
12.));
#58926=CARTESIAN_POINT('Ctrl Pts',(-8.99263343720554,-15.5918113841942,
12.));
#58927=CARTESIAN_POINT('Ctrl Pts',(-9.069430157416,-15.533374159028,12.));
#58928=CARTESIAN_POINT('Ctrl Pts',(-9.13662728760015,-15.4822415870076,
12.));
#58929=CARTESIAN_POINT('Ctrl Pts',(-9.20179743619592,-15.4282631425356,
12.));
#58930=CARTESIAN_POINT('Ctrl Pts',(-9.26474763112753,-15.3715835638146,
12.));
#58931=CARTESIAN_POINT('Ctrl Pts',(-9.27985611388604,-15.3579800723751,
12.));
#58932=CARTESIAN_POINT('Ctrl Pts',(-9.29484029179697,-15.3442173582628,
12.));
#58933=CARTESIAN_POINT('Ctrl Pts',(-9.30967505138841,-15.3303185989115,
12.));
#58934=CARTESIAN_POINT('Ctrl Pts',(-9.38210503428163,-15.26245859108,12.));
#58935=CARTESIAN_POINT('Ctrl Pts',(-9.45106917065939,-15.1912779029607,
12.));
#58936=CARTESIAN_POINT('Ctrl Pts',(-9.51632647275336,-15.1170649381822,
12.));
#58937=CARTESIAN_POINT('Ctrl Pts',(-9.58121888012541,-15.0432669448824,
12.));
#58938=CARTESIAN_POINT('Ctrl Pts',(-9.64244627908667,-14.9664696982533,
12.));
#58939=CARTESIAN_POINT('Ctrl Pts',(-9.69972810245665,-14.8869300127004,
12.));
#58940=CARTESIAN_POINT('Ctrl Pts',(-9.75408287639578,-14.81145473323,12.));
#58941=CARTESIAN_POINT('Ctrl Pts',(-9.80488505097158,-14.7335093955071,
12.));
#58942=CARTESIAN_POINT('Ctrl Pts',(-9.85185230919616,-14.6533004074739,
12.));
#58943=CARTESIAN_POINT('Ctrl Pts',(-9.8892295724543,-14.5894688666365,12.));
#58944=CARTESIAN_POINT('Ctrl Pts',(-9.92417736747258,-14.5242033609892,
12.));
#58945=CARTESIAN_POINT('Ctrl Pts',(-9.95653206305223,-14.4576058296606,
12.));
#58946=CARTESIAN_POINT('Ctrl Pts',(-9.96243497650182,-14.4454555233034,
12.));
#58947=CARTESIAN_POINT('Ctrl Pts',(-9.9682498087257,-14.4332643188572,12.));
#58948=CARTESIAN_POINT('Ctrl Pts',(-9.97397236800321,-14.4210401757467,
12.));
#58949=CARTESIAN_POINT('Ctrl Pts',(-10.014548795905,-14.3343635617469,12.));
#58950=CARTESIAN_POINT('Ctrl Pts',(-10.0505434398104,-14.2459232997935,
12.));
#58951=CARTESIAN_POINT('Ctrl Pts',(-10.0816927676552,-14.1559630239742,
12.));
#58952=CARTESIAN_POINT('Ctrl Pts',(-10.1128420955,-14.0660027481548,12.));
#58953=CARTESIAN_POINT('Ctrl Pts',(-10.1391465733587,-13.9745217251954,
12.));
#58954=CARTESIAN_POINT('Ctrl Pts',(-10.1602864633442,-13.8817537764296,
12.));
#58955=CARTESIAN_POINT('Ctrl Pts',(-10.1814515048034,-13.7888754557256,
12.));
#58956=CARTESIAN_POINT('Ctrl Pts',(-10.1974388881398,-13.6947059611701,
12.));
#58957=CARTESIAN_POINT('Ctrl Pts',(-10.2083240537505,-13.5996534977197,
12.));
#58958=CARTESIAN_POINT('Ctrl Pts',(-10.2138911337605,-13.5510401198348,
12.));
#58959=CARTESIAN_POINT('Ctrl Pts',(-10.2181228103627,-13.5021959582282,
12.));
#58960=CARTESIAN_POINT('Ctrl Pts',(-10.221024235662,-13.4531774228974,12.));
#58961=CARTESIAN_POINT('Ctrl Pts',(-10.2218608104944,-13.4390437924411,
12.));
#58962=CARTESIAN_POINT('Ctrl Pts',(-10.2225867738812,-13.4248956759012,
12.));
#58963=CARTESIAN_POINT('Ctrl Pts',(-10.2232022007112,-13.410734453067,12.));
#58964=CARTESIAN_POINT('Ctrl Pts',(-10.2238234019696,-13.3964403582763,
12.));
#58965=CARTESIAN_POINT('Ctrl Pts',(-10.2243315800161,-13.3821418174545,
12.));
#58966=CARTESIAN_POINT('Ctrl Pts',(-10.2247271750585,-13.3678432915664,
12.));
#58967=CARTESIAN_POINT('Ctrl Pts',(-10.2273082491492,-13.2745520448321,
12.));
#58968=CARTESIAN_POINT('Ctrl Pts',(-10.2251029799825,-13.1812181718667,
12.));
#58969=CARTESIAN_POINT('Ctrl Pts',(-10.2182398910409,-13.0882187710056,
12.));
#58970=CARTESIAN_POINT('Ctrl Pts',(-10.2113725866781,-12.9951622483964,
12.));
#58971=CARTESIAN_POINT('Ctrl Pts',(-10.1998413619504,-12.902439631583,12.));
#58972=CARTESIAN_POINT('Ctrl Pts',(-10.1837244231874,-12.810441427736,12.));
#58973=CARTESIAN_POINT('Ctrl Pts',(-10.1678505565058,-12.7198307203121,
12.));
#58974=CARTESIAN_POINT('Ctrl Pts',(-10.1475277985646,-12.629921903999,12.));
#58975=CARTESIAN_POINT('Ctrl Pts',(-10.1227882064871,-12.5411137713789,
12.));
#58976=CARTESIAN_POINT('Ctrl Pts',(-10.1129089207081,-12.5056499319226,
12.));
#58977=CARTESIAN_POINT('Ctrl Pts',(-10.1023248586868,-12.4703619714101,
12.));
#58978=CARTESIAN_POINT('Ctrl Pts',(-10.0910363601597,-12.435276902831,12.));
#58979=CARTESIAN_POINT('Ctrl Pts',(-10.0850884600019,-12.4167906103951,
12.));
#58980=CARTESIAN_POINT('Ctrl Pts',(-10.0789449767355,-12.398360662607,12.));
#58981=CARTESIAN_POINT('Ctrl Pts',(-10.0726058589696,-12.3799911333697,
12.));
#58982=CARTESIAN_POINT('Ctrl Pts',(-10.0672510463096,-12.3644739287129,
12.));
#58983=CARTESIAN_POINT('Ctrl Pts',(-10.0617592067699,-12.349007385008,12.));
#58984=CARTESIAN_POINT('Ctrl Pts',(-10.0561325433239,-12.3335987119335,
12.));
#58985=CARTESIAN_POINT('Ctrl Pts',(-10.0253173441252,-12.2492109864665,
12.));
#58986=CARTESIAN_POINT('Ctrl Pts',(-9.99044488561477,-12.166508346864,12.));
#58987=CARTESIAN_POINT('Ctrl Pts',(-9.95156719631022,-12.0858609769308,
12.));
#58988=CARTESIAN_POINT('Ctrl Pts',(-9.92246136851044,-12.0254842286268,
12.));
#58989=CARTESIAN_POINT('Ctrl Pts',(-9.89110980665403,-11.9662598549223,
12.));
#58990=CARTESIAN_POINT('Ctrl Pts',(-9.85752076592995,-11.9083564676894,
12.));
#58991=CARTESIAN_POINT('Ctrl Pts',(-9.84460179101728,-11.8860857391751,
12.));
#58992=CARTESIAN_POINT('Ctrl Pts',(-9.83135170784992,-11.8640105638195,
12.));
#58993=CARTESIAN_POINT('Ctrl Pts',(-9.81777057146904,-11.8421410854707,
12.));
#58994=CARTESIAN_POINT('Ctrl Pts',(-9.80600924137691,-11.8232020109641,
12.));
#58995=CARTESIAN_POINT('Ctrl Pts',(-9.79399765022805,-11.8044144459084,
12.));
#58996=CARTESIAN_POINT('Ctrl Pts',(-9.78175006557354,-11.7858062660097,
12.));
#58997=CARTESIAN_POINT('Ctrl Pts',(-9.73447815410214,-11.7139844123438,
12.));
#58998=CARTESIAN_POINT('Ctrl Pts',(-9.68365479534874,-11.6447676019631,
12.));
#58999=CARTESIAN_POINT('Ctrl Pts',(-9.62930896131935,-11.578509745124,12.));
#59000=CARTESIAN_POINT('Ctrl Pts',(-9.58717521523442,-11.5271407346737,
12.));
#59001=CARTESIAN_POINT('Ctrl Pts',(-9.54292346973057,-11.477550842089,12.));
#59002=CARTESIAN_POINT('Ctrl Pts',(-9.49655480089338,-11.4299227460007,
12.));
#59003=CARTESIAN_POINT('Ctrl Pts',(-9.47068894114788,-11.4033543392671,
12.));
#59004=CARTESIAN_POINT('Ctrl Pts',(-9.44416412664311,-11.377396721654,12.));
#59005=CARTESIAN_POINT('Ctrl Pts',(-9.41700750114215,-11.3520617378123,
12.));
#59006=CARTESIAN_POINT('Origin',(-7.50000000000001,-12.9903810567666,7.5));
#59007=CARTESIAN_POINT('Origin',(-7.5,12.9903810567666,4.));
#59008=CARTESIAN_POINT('Ctrl Pts',(-9.41346599666504,14.6263682601415,4.));
#59009=CARTESIAN_POINT('Ctrl Pts',(-9.47563132777586,14.5679481137415,4.));
#59010=CARTESIAN_POINT('Ctrl Pts',(-9.53442555802215,14.506276247837,4.));
#59011=CARTESIAN_POINT('Ctrl Pts',(-9.58983471826803,14.4417285757633,4.));
#59012=CARTESIAN_POINT('Ctrl Pts',(-9.64659435921208,14.3756076911582,4.));
#59013=CARTESIAN_POINT('Ctrl Pts',(-9.69980238305237,14.3064686172689,4.));
#59014=CARTESIAN_POINT('Ctrl Pts',(-9.7494149473681,14.2346691598829,4.));
#59015=CARTESIAN_POINT('Ctrl Pts',(-9.76242041292079,14.2158476096845,4.));
#59016=CARTESIAN_POINT('Ctrl Pts',(-9.77517863474719,14.1968430256296,4.));
#59017=CARTESIAN_POINT('Ctrl Pts',(-9.78768844229491,14.177661413676,4.));
#59018=CARTESIAN_POINT('Ctrl Pts',(-9.79776816908292,14.1622059074975,4.));
#59019=CARTESIAN_POINT('Ctrl Pts',(-9.80768698071961,14.1466346904616,4.));
#59020=CARTESIAN_POINT('Ctrl Pts',(-9.81743563533852,14.1309651390747,4.));
#59021=CARTESIAN_POINT('Ctrl Pts',(-9.86491280549081,14.0546524593777,4.));
#59022=CARTESIAN_POINT('Ctrl Pts',(-9.90840772399799,13.9759343990068,4.));
#59023=CARTESIAN_POINT('Ctrl Pts',(-9.94788354450479,13.8952025688597,4.));
#59024=CARTESIAN_POINT('Ctrl Pts',(-9.97942538424941,13.8306964885275,4.));
#59025=CARTESIAN_POINT('Ctrl Pts',(-10.0084008056984,13.7649036744675,4.));
#59026=CARTESIAN_POINT('Ctrl Pts',(-10.0347744493784,13.6980066802042,4.));
#59027=CARTESIAN_POINT('Ctrl Pts',(-10.0434535064654,13.6759921705975,4.));
#59028=CARTESIAN_POINT('Ctrl Pts',(-10.0518506786378,13.6538579807081,4.));
#59029=CARTESIAN_POINT('Ctrl Pts',(-10.0599643178554,13.6316103344208,4.));
#59030=CARTESIAN_POINT('Ctrl Pts',(-10.0673321856527,13.6114075977388,4.));
#59031=CARTESIAN_POINT('Ctrl Pts',(-10.0744676826305,13.591106675655,4.));
#59032=CARTESIAN_POINT('Ctrl Pts',(-10.0813601244641,13.5707407736482,4.));
#59033=CARTESIAN_POINT('Ctrl Pts',(-10.110937889366,13.4833439009404,4.));
#59034=CARTESIAN_POINT('Ctrl Pts',(-10.1360768470728,13.3946653712955,4.));
#59035=CARTESIAN_POINT('Ctrl Pts',(-10.1567422986514,13.3051020151044,4.));
#59036=CARTESIAN_POINT('Ctrl Pts',(-10.1777244132853,13.2141662521254,4.));
#59037=CARTESIAN_POINT('Ctrl Pts',(-10.194095376586,13.1223175335281,4.));
#59038=CARTESIAN_POINT('Ctrl Pts',(-10.205777094777,13.0299380601523,4.));
#59039=CARTESIAN_POINT('Ctrl Pts',(-10.2173678863481,12.938277637958,4.));
#59040=CARTESIAN_POINT('Ctrl Pts',(-10.2243424959595,12.8460937642312,4.));
#59041=CARTESIAN_POINT('Ctrl Pts',(-10.2265776894176,12.7537405691803,4.));
#59042=CARTESIAN_POINT('Ctrl Pts',(-10.2276571919675,12.7091379379498,4.));
#59043=CARTESIAN_POINT('Ctrl Pts',(-10.2276305022847,12.6644956114825,4.));
#59044=CARTESIAN_POINT('Ctrl Pts',(-10.226479393828,12.619852841063,4.));
#59045=CARTESIAN_POINT('Ctrl Pts',(-10.2261091350259,12.6054933090796,4.));
#59046=CARTESIAN_POINT('Ctrl Pts',(-10.2256225193086,12.5911337303501,4.));
#59047=CARTESIAN_POINT('Ctrl Pts',(-10.225018873735,12.5767754108853,4.));
#59048=CARTESIAN_POINT('Ctrl Pts',(-10.2243878291515,12.5617653783061,4.));
#59049=CARTESIAN_POINT('Ctrl Pts',(-10.2236292144324,12.5467651944381,4.));
#59050=CARTESIAN_POINT('Ctrl Pts',(-10.2227430773117,12.5317818464922,4.));
#59051=CARTESIAN_POINT('Ctrl Pts',(-10.21709364836,12.436257849471,4.));
#59052=CARTESIAN_POINT('Ctrl Pts',(-10.2062620470353,12.3413497626712,4.));
#59053=CARTESIAN_POINT('Ctrl Pts',(-10.1901757223778,12.2474518873064,4.));
#59054=CARTESIAN_POINT('Ctrl Pts',(-10.1886872627285,12.2387635634276,4.));
#59055=CARTESIAN_POINT('Ctrl Pts',(-10.1871537792193,12.2300838755081,4.));
#59056=CARTESIAN_POINT('Ctrl Pts',(-10.1855751929644,12.2214131286805,4.));
#59057=CARTESIAN_POINT('Ctrl Pts',(-10.1691864185716,12.1313940289104,4.));
#59058=CARTESIAN_POINT('Ctrl Pts',(-10.1479406949308,12.0423388878924,4.));
#59059=CARTESIAN_POINT('Ctrl Pts',(-10.1221403086027,11.9544825435439,4.));
#59060=CARTESIAN_POINT('Ctrl Pts',(-10.095748827746,11.8646133842016,4.));
#59061=CARTESIAN_POINT('Ctrl Pts',(-10.0645913960745,11.7759978814463,4.));
#59062=CARTESIAN_POINT('Ctrl Pts',(-10.0289372513566,11.6888902934565,4.));
#59063=CARTESIAN_POINT('Ctrl Pts',(-10.0090455594271,11.6402923725491,4.));
#59064=CARTESIAN_POINT('Ctrl Pts',(-9.98775327367975,11.5921639163278,4.));
#59065=CARTESIAN_POINT('Ctrl Pts',(-9.96510045219232,11.5445507349067,4.));
#59066=CARTESIAN_POINT('Ctrl Pts',(-9.95876521331174,11.5312349155799,4.));
#59067=CARTESIAN_POINT('Ctrl Pts',(-9.95232326498233,11.517959024353,4.));
#59068=CARTESIAN_POINT('Ctrl Pts',(-9.94578250287666,11.504737914807,4.));
#59069=CARTESIAN_POINT('Ctrl Pts',(-9.90302508933715,11.4183106087567,4.));
#59070=CARTESIAN_POINT('Ctrl Pts',(-9.85598190542476,11.3340799660434,4.));
#59071=CARTESIAN_POINT('Ctrl Pts',(-9.80499298346813,11.2522993127725,4.));
#59072=CARTESIAN_POINT('Ctrl Pts',(-9.75299886407878,11.1689064327755,4.));
#59073=CARTESIAN_POINT('Ctrl Pts',(-9.69690158938222,11.0880603146916,4.));
#59074=CARTESIAN_POINT('Ctrl Pts',(-9.63700679973682,11.0100365149775,4.));
#59075=CARTESIAN_POINT('Ctrl Pts',(-9.57664072131881,10.9313987763712,4.));
#59076=CARTESIAN_POINT('Ctrl Pts',(-9.5124166745289,10.855627103721,4.00000000000001));
#59077=CARTESIAN_POINT('Ctrl Pts',(-9.44459833298039,10.7830228983692,4.00000000000001));
#59078=CARTESIAN_POINT('Ctrl Pts',(-9.40866399637306,10.7445527161936,4.00000000000001));
#59079=CARTESIAN_POINT('Ctrl Pts',(-9.37171976510391,10.706972211061,4.));
#59080=CARTESIAN_POINT('Ctrl Pts',(-9.33380001260192,10.67032964942,4.));
#59081=CARTESIAN_POINT('Ctrl Pts',(-9.31851279266197,10.655557324655,4.));
#59082=CARTESIAN_POINT('Ctrl Pts',(-9.30306698875868,10.6409374727743,4.00000000000001));
#59083=CARTESIAN_POINT('Ctrl Pts',(-9.28746471547238,10.6264733925429,4.00000000000001));
#59084=CARTESIAN_POINT('Ctrl Pts',(-9.27676484992977,10.616554087142,4.00000000000001));
#59085=CARTESIAN_POINT('Ctrl Pts',(-9.265998221379,10.6067143856922,4.00000000000001));
#59086=CARTESIAN_POINT('Ctrl Pts',(-9.25516722641356,10.5969563651344,4.00000000000001));
#59087=CARTESIAN_POINT('Ctrl Pts',(-9.17938034347013,10.5286773229844,4.));
#59088=CARTESIAN_POINT('Ctrl Pts',(-9.10042408605055,10.4643755397515,4.));
#59089=CARTESIAN_POINT('Ctrl Pts',(-9.01862125042457,10.4043372079866,4.));
#59090=CARTESIAN_POINT('Ctrl Pts',(-8.9367488325877,10.344247807089,4.));
#59091=CARTESIAN_POINT('Ctrl Pts',(-8.85202442117708,10.2884282704825,4.));
#59092=CARTESIAN_POINT('Ctrl Pts',(-8.76472673601652,10.2371917535793,4.00000000000001));
#59093=CARTESIAN_POINT('Ctrl Pts',(-8.67911981959232,10.1869475780055,4.00000000000001));
#59094=CARTESIAN_POINT('Ctrl Pts',(-8.59103768625539,10.1411099279233,4.));
#59095=CARTESIAN_POINT('Ctrl Pts',(-8.50070929346997,10.1000104724858,4.));
#59096=CARTESIAN_POINT('Ctrl Pts',(-8.47449841652962,10.0880845128227,4.));
#59097=CARTESIAN_POINT('Ctrl Pts',(-8.4480982164028,10.0765577851635,4.));
#59098=CARTESIAN_POINT('Ctrl Pts',(-8.42151385798486,10.0654391093543,4.));
#59099=CARTESIAN_POINT('Ctrl Pts',(-8.38003010456224,10.0480888916659,4.));
#59100=CARTESIAN_POINT('Ctrl Pts',(-8.33809795636191,10.0317321930114,4.));
#59101=CARTESIAN_POINT('Ctrl Pts',(-8.29574920379127,10.0163624306404,4.));
#59102=CARTESIAN_POINT('Ctrl Pts',(-6.70620071746715,10.0211581030209,4.));
#59103=CARTESIAN_POINT('Ctrl Pts',(-6.61134536198573,10.0558566157721,4.));
#59104=CARTESIAN_POINT('Ctrl Pts',(-6.51853047906358,10.0955386450798,4.));
#59105=CARTESIAN_POINT('Ctrl Pts',(-6.42799833026157,10.1398859077314,4.));
#59106=CARTESIAN_POINT('Ctrl Pts',(-6.33621672682966,10.1848452169695,4.));
#59107=CARTESIAN_POINT('Ctrl Pts',(-6.24678063208038,10.2346001195317,4.));
#59108=CARTESIAN_POINT('Ctrl Pts',(-6.15997649545542,10.288859611306,4.));
#59109=CARTESIAN_POINT('Ctrl Pts',(-6.13531542249315,10.3042747440124,4.));
#59110=CARTESIAN_POINT('Ctrl Pts',(-6.11086702515844,10.3200536672633,4.));
#59111=CARTESIAN_POINT('Ctrl Pts',(-6.0866384800126,10.3361901726906,4.));
#59112=CARTESIAN_POINT('Ctrl Pts',(-6.06744058816026,10.3489762019054,4.));
#59113=CARTESIAN_POINT('Ctrl Pts',(-6.04837875428141,10.3619882719582,4.));
#59114=CARTESIAN_POINT('Ctrl Pts',(-6.0294755109822,10.37520976247,4.));
#59115=CARTESIAN_POINT('Ctrl Pts',(-5.9467711696009,10.43305563831,4.));
#59116=CARTESIAN_POINT('Ctrl Pts',(-5.86702033335456,10.4949586291912,4.));
#59117=CARTESIAN_POINT('Ctrl Pts',(-5.79049045427403,10.5606238082624,4.));
#59118=CARTESIAN_POINT('Ctrl Pts',(-5.73202499106291,10.6107891183003,4.));
#59119=CARTESIAN_POINT('Ctrl Pts',(-5.67544001899664,10.6631510546145,4.));
#59120=CARTESIAN_POINT('Ctrl Pts',(-5.62087181378523,10.7175895430331,4.));
#59121=CARTESIAN_POINT('Ctrl Pts',(-5.59237441395403,10.7460192002787,4.));
#59122=CARTESIAN_POINT('Ctrl Pts',(-5.56442730562685,10.7750153331146,4.));
#59123=CARTESIAN_POINT('Ctrl Pts',(-5.53705172637329,10.8045615976092,4.));
#59124=CARTESIAN_POINT('Ctrl Pts',(-5.52590399611565,10.8165932621689,4.));
#59125=CARTESIAN_POINT('Ctrl Pts',(-5.51485083286264,10.828716515658,4.));
#59126=CARTESIAN_POINT('Ctrl Pts',(-5.50390377375039,10.8409187451704,4.));
#59127=CARTESIAN_POINT('Ctrl Pts',(-5.43813900242605,10.9142239886428,4.));
#59128=CARTESIAN_POINT('Ctrl Pts',(-5.37610793089156,10.9904753850308,4.));
#59129=CARTESIAN_POINT('Ctrl Pts',(-5.31805547404601,11.0693968127291,4.));
#59130=CARTESIAN_POINT('Ctrl Pts',(-5.26107067938322,11.14686677001,4.));
#59131=CARTESIAN_POINT('Ctrl Pts',(-5.20791915062963,11.2269102402285,4.));
#59132=CARTESIAN_POINT('Ctrl Pts',(-5.15887680160751,11.3092877421736,4.));
#59133=CARTESIAN_POINT('Ctrl Pts',(-5.11076852001942,11.390096270703,4.));
#59134=CARTESIAN_POINT('Ctrl Pts',(-5.0666140967032,11.4731514387505,4.));
#59135=CARTESIAN_POINT('Ctrl Pts',(-5.0267215928916,11.558237595229,4.));
#59136=CARTESIAN_POINT('Ctrl Pts',(-5.00642757575884,11.6015224169963,4.));
#59137=CARTESIAN_POINT('Ctrl Pts',(-4.98723731004213,11.6453329516309,4.));
#59138=CARTESIAN_POINT('Ctrl Pts',(-4.96919657902753,11.6896410472644,4.));
#59139=CARTESIAN_POINT('Ctrl Pts',(-4.96034359773442,11.7113839988919,4.));
#59140=CARTESIAN_POINT('Ctrl Pts',(-4.95176748954608,11.7332467663051,4.));
#59141=CARTESIAN_POINT('Ctrl Pts',(-4.94347399674913,11.7552260059165,4.));
#59142=CARTESIAN_POINT('Ctrl Pts',(-4.93874124380541,11.7677686479032,4.));
#59143=CARTESIAN_POINT('Ctrl Pts',(-4.93410183231377,11.780345881655,4.));
#59144=CARTESIAN_POINT('Ctrl Pts',(-4.92955939125163,11.7929492290495,4.));
#59145=CARTESIAN_POINT('Ctrl Pts',(-4.89805310423436,11.8803658129868,4.));
#59146=CARTESIAN_POINT('Ctrl Pts',(-4.87116553516298,11.9691490179121,4.));
#59147=CARTESIAN_POINT('Ctrl Pts',(-4.84914983533523,12.059077444786,4.));
#59148=CARTESIAN_POINT('Ctrl Pts',(-4.84589756836606,12.0723621123006,4.));
#59149=CARTESIAN_POINT('Ctrl Pts',(-4.84275170968814,12.0856717889067,4.));
#59150=CARTESIAN_POINT('Ctrl Pts',(-4.83971317200452,12.0990057760668,4.));
#59151=CARTESIAN_POINT('Ctrl Pts',(-4.81880138299547,12.1907727887468,4.));
#59152=CARTESIAN_POINT('Ctrl Pts',(-4.80296850182884,12.2836914928978,4.));
#59153=CARTESIAN_POINT('Ctrl Pts',(-4.792106149773,12.377370023065,4.));
#59154=CARTESIAN_POINT('Ctrl Pts',(-4.78082380016171,12.4746706742486,4.));
#59155=CARTESIAN_POINT('Ctrl Pts',(-4.77490383217972,12.5727922441963,4.));
#59156=CARTESIAN_POINT('Ctrl Pts',(-4.77428144864228,12.6712822681824,4.));
#59157=CARTESIAN_POINT('Ctrl Pts',(-4.77410039443767,12.6999334645636,4.));
#59158=CARTESIAN_POINT('Ctrl Pts',(-4.77436800145517,12.72861569198,4.));
#59159=CARTESIAN_POINT('Ctrl Pts',(-4.77508351480076,12.7573173782009,4.));
#59160=CARTESIAN_POINT('Ctrl Pts',(-4.77547910205812,12.7731857353794,4.));
#59161=CARTESIAN_POINT('Ctrl Pts',(-4.77601160613275,12.7890600363428,4.));
#59162=CARTESIAN_POINT('Ctrl Pts',(-4.77668094646708,12.8049382921795,4.));
#59163=CARTESIAN_POINT('Ctrl Pts',(-4.77726157393708,12.8187120796562,4.));
#59164=CARTESIAN_POINT('Ctrl Pts',(-4.77794517105296,12.8324874411773,4.));
#59165=CARTESIAN_POINT('Ctrl Pts',(-4.77873077105928,12.846250960695,4.));
#59166=CARTESIAN_POINT('Ctrl Pts',(-4.7840331030193,12.9391465167459,4.));
#59167=CARTESIAN_POINT('Ctrl Pts',(-4.79398369008647,13.0316542436184,4.));
#59168=CARTESIAN_POINT('Ctrl Pts',(-4.80846381204201,13.1234011743035,4.));
#59169=CARTESIAN_POINT('Ctrl Pts',(-4.82290319752883,13.2148899962528,4.));
#59170=CARTESIAN_POINT('Ctrl Pts',(-4.84184707271793,13.3056232412176,4.));
#59171=CARTESIAN_POINT('Ctrl Pts',(-4.86522626081521,13.3952139858104,4.));
#59172=CARTESIAN_POINT('Ctrl Pts',(-4.88820180858057,13.4832579513734,4.));
#59173=CARTESIAN_POINT('Ctrl Pts',(-4.91546130118121,13.5701993091168,4.));
#59174=CARTESIAN_POINT('Ctrl Pts',(-4.94697947428434,13.6556416339958,4.));
#59175=CARTESIAN_POINT('Ctrl Pts',(-4.9623719301486,13.6973689006853,4.));
#59176=CARTESIAN_POINT('Ctrl Pts',(-4.97878066818245,13.7387381251278,4.));
#59177=CARTESIAN_POINT('Ctrl Pts',(-4.99620585058615,13.779699693788,4.));
#59178=CARTESIAN_POINT('Ctrl Pts',(-5.00196797407456,13.7932447810892,4.));
#59179=CARTESIAN_POINT('Ctrl Pts',(-5.00784125922211,13.8067452713773,4.));
#59180=CARTESIAN_POINT('Ctrl Pts',(-5.01382575727085,13.8201993070928,4.));
#59181=CARTESIAN_POINT('Ctrl Pts',(-5.01951346999181,13.8329861255467,4.));
#59182=CARTESIAN_POINT('Ctrl Pts',(-5.02529821878992,13.8457232464252,4.));
#59183=CARTESIAN_POINT('Ctrl Pts',(-5.03117811610162,13.8584059204054,4.));
#59184=CARTESIAN_POINT('Ctrl Pts',(-5.06862984407309,13.9391876127847,4.));
#59185=CARTESIAN_POINT('Ctrl Pts',(-5.10995846184345,14.0178080548726,4.));
#59186=CARTESIAN_POINT('Ctrl Pts',(-5.15509821873846,14.0939187469392,4.));
#59187=CARTESIAN_POINT('Ctrl Pts',(-5.19948177774165,14.1687544045606,4.));
#59188=CARTESIAN_POINT('Ctrl Pts',(-5.24755030145435,14.2411643668113,4.));
#59189=CARTESIAN_POINT('Ctrl Pts',(-5.299277628138,14.3107831411822,4.));
#59190=CARTESIAN_POINT('Ctrl Pts',(-5.34947359960038,14.37834089519,4.));
#59191=CARTESIAN_POINT('Ctrl Pts',(-5.40311538240653,14.4432707274223,4.));
#59192=CARTESIAN_POINT('Ctrl Pts',(-5.46020707398797,14.5051981890779,4.));
#59193=CARTESIAN_POINT('Ctrl Pts',(-5.47440626361873,14.5206000758857,4.));
#59194=CARTESIAN_POINT('Ctrl Pts',(-5.48881897228929,14.5358160294758,4.));
#59195=CARTESIAN_POINT('Ctrl Pts',(-5.50344549658044,14.5508398362218,4.));
#59196=CARTESIAN_POINT('Ctrl Pts',(-5.52930175835117,14.5773984001217,4.));
#59197=CARTESIAN_POINT('Ctrl Pts',(-5.55582619547196,14.603356583853,4.));
#59198=CARTESIAN_POINT('Ctrl Pts',(-5.58299280741585,14.6287008947316,4.));
#59199=CARTESIAN_POINT('Origin',(-7.5,12.9903810567666,14.2084234471775));
#59200=CARTESIAN_POINT('Ctrl Pts',(-10.5771718362758,12.9919049495641,11.7084234471775));
#59201=CARTESIAN_POINT('Ctrl Pts',(-10.5778105116372,13.0907937922778,11.7032843782051));
#59202=CARTESIAN_POINT('Ctrl Pts',(-10.5289894981275,14.1961054493059,11.6458119334487));
#59203=CARTESIAN_POINT('Ctrl Pts',(-9.19520332408216,16.188335839362,11.5360061129082));
#59204=CARTESIAN_POINT('Ctrl Pts',(-5.76804722455709,16.1681372027015,11.3790059855559));
#59205=CARTESIAN_POINT('Ctrl Pts',(-3.89395310615829,13.2989500353867,11.2220058582037));
#59206=CARTESIAN_POINT('Ctrl Pts',(-5.25343413560966,10.1527921984098,11.0650057308514));
#59207=CARTESIAN_POINT('Ctrl Pts',(-8.62743319586002,9.55126751773617,10.9080056034992));
#59208=CARTESIAN_POINT('Ctrl Pts',(-10.416413733365,11.4305453719444,10.7891448422745));
#59209=CARTESIAN_POINT('Ctrl Pts',(-10.5747253393417,12.713490324996,10.7226174568339));
#59210=CARTESIAN_POINT('Ctrl Pts',(-10.5724150045772,12.9877735244422,10.7084234471775));
#59211=CARTESIAN_POINT('Ctrl Pts',(-10.5702206634037,12.9870745539208,11.7915765528226));
#59212=CARTESIAN_POINT('Ctrl Pts',(-10.5655505963514,13.6681072977096,11.7563842836469));
#59213=CARTESIAN_POINT('Ctrl Pts',(-10.0102057878341,15.3711021382601,11.6688586386871));
#59214=CARTESIAN_POINT('Ctrl Pts',(-7.21365218567195,16.5973810760335,11.5289996179432));
#59215=CARTESIAN_POINT('Ctrl Pts',(-4.33342713054201,14.7428462583649,11.371999490591));
#59216=CARTESIAN_POINT('Ctrl Pts',(-4.29152522806557,11.3151739482887,11.2149993632387));
#59217=CARTESIAN_POINT('Ctrl Pts',(-7.12729264284838,9.39053585671186,11.0579992358865));
#59218=CARTESIAN_POINT('Ctrl Pts',(-9.97678331927841,10.5618592714599,10.9168582990811));
#59219=CARTESIAN_POINT('Ctrl Pts',(-10.5660598502819,12.2874997426315,10.8280507380598));
#59220=CARTESIAN_POINT('Ctrl Pts',(-10.5715490487462,12.9928368154298,10.7915765528225));
#59221=CARTESIAN_POINT('Ctrl Pts',(-5.58653400333492,14.6263682601415,12.));
#59222=CARTESIAN_POINT('Ctrl Pts',(-5.04858820392146,13.9971818012847,11.9476666242159));
#59223=CARTESIAN_POINT('Ctrl Pts',(-4.6501298356162,12.1775391083675,11.8429998726477));
#59224=CARTESIAN_POINT('Ctrl Pts',(-6.60905434274384,10.1611067275626,11.6859997452955));
#59225=CARTESIAN_POINT('Ctrl Pts',(-9.36683572422696,10.6884384302024,11.5289996179432));
#59226=CARTESIAN_POINT('Ctrl Pts',(-10.4505967777648,13.2766298839747,11.371999490591));
#59227=CARTESIAN_POINT('Ctrl Pts',(-8.88853891927017,15.609821813293,11.2149993632387));
#59228=CARTESIAN_POINT('Ctrl Pts',(-6.0813596511542,15.5932771353061,11.0579992358865));
#59229=CARTESIAN_POINT('Ctrl Pts',(-4.5462915063457,13.2431295206274,10.9009991085342));
#59230=CARTESIAN_POINT('Ctrl Pts',(-5.65984071462414,10.666115577374,10.743998981182));
#59231=CARTESIAN_POINT('Ctrl Pts',(-8.42347911845702,10.1734074649302,10.5869988538297));
#59232=CARTESIAN_POINT('Ctrl Pts',(-10.3590245740303,12.2066479805288,10.4299987264775));
#59233=CARTESIAN_POINT('Ctrl Pts',(-9.73085545152254,14.9426994258741,10.2729985991252));
#59234=CARTESIAN_POINT('Ctrl Pts',(-7.10225674886102,15.9280729453192,10.115998471773));
#59235=CARTESIAN_POINT('Ctrl Pts',(-4.8303182837872,14.2791977933351,9.9589983444207));
#59236=CARTESIAN_POINT('Ctrl Pts',(-4.95230900060974,11.4746243081013,9.80199821706846));
#59237=CARTESIAN_POINT('Ctrl Pts',(-7.35883869070172,10.0292464861065,9.64499808971619));
#59238=CARTESIAN_POINT('Ctrl Pts',(-9.89194907460283,11.2391453960705,9.48799796236395));
#59239=CARTESIAN_POINT('Ctrl Pts',(-10.2801757792987,14.0193946579201,9.33099783501168));
#59240=CARTESIAN_POINT('Ctrl Pts',(-8.17539218920641,15.8769172785782,9.17399770765945));
#59241=CARTESIAN_POINT('Ctrl Pts',(-5.46497794449781,15.1460553165716,9.01699758030717));
#59242=CARTESIAN_POINT('Ctrl Pts',(-4.57938749963505,12.4821794938336,8.85999745295494));
#59243=CARTESIAN_POINT('Ctrl Pts',(-6.31273830315983,10.2740129245224,8.70299732560267));
#59244=CARTESIAN_POINT('Ctrl Pts',(-9.11071806020523,10.501639700397,8.54599719825042));
#59245=CARTESIAN_POINT('Ctrl Pts',(-10.4643514801813,12.96094473598,8.38899707089817));
#59246=CARTESIAN_POINT('Ctrl Pts',(-9.15982248917363,15.4466455979041,8.23199694354592));
#59247=CARTESIAN_POINT('Ctrl Pts',(-6.36691474847379,15.7297904840163,8.07499681619367));
#59248=CARTESIAN_POINT('Ctrl Pts',(-4.59005542323444,13.5564806545976,7.91799668884141));
#59249=CARTESIAN_POINT('Ctrl Pts',(-5.42257131653894,10.8755438858135,7.76099656148916));
#59250=CARTESIAN_POINT('Ctrl Pts',(-8.11793744062105,10.0910018961859,7.6039964341369));
#59251=CARTESIAN_POINT('Ctrl Pts',(-10.2591931327486,11.9063610164495,7.44699630678465));
#59252=CARTESIAN_POINT('Ctrl Pts',(-9.92625387366264,14.6937713043528,7.2899961794324));
#59253=CARTESIAN_POINT('Ctrl Pts',(-7.41766948685395,15.953735219701,7.13299605208014));
#59254=CARTESIAN_POINT('Ctrl Pts',(-4.98291166647307,14.5564310201707,6.97599592472789));
#59255=CARTESIAN_POINT('Ctrl Pts',(-4.80525109196198,11.7548348097635,6.81899579737564));
#59256=CARTESIAN_POINT('Ctrl Pts',(-7.04399773638617,10.061164742401,6.66199567002339));
#59257=CARTESIAN_POINT('Ctrl Pts',(-9.69164594449512,10.9941511043189,6.50499554267113));
#59258=CARTESIAN_POINT('Ctrl Pts',(-10.3740242882686,13.7171759009976,6.34799541531889));
#59259=CARTESIAN_POINT('Ctrl Pts',(-8.47923732450549,15.7884770124268,6.19099528796661));
#59260=CARTESIAN_POINT('Ctrl Pts',(-5.70635916288519,15.3506981982192,6.03399516061438));
#59261=CARTESIAN_POINT('Ctrl Pts',(-4.54185534982472,12.7964012172524,5.87699503326211));
#59262=CARTESIAN_POINT('Ctrl Pts',(-6.02994939266268,10.4160461410637,5.71999490590986));
#59263=CARTESIAN_POINT('Ctrl Pts',(-8.83624963123305,10.3441251642037,5.56299477855761));
#59264=CARTESIAN_POINT('Ctrl Pts',(-10.4443264801503,12.6451208096654,5.40599465120535));
#59265=CARTESIAN_POINT('Ctrl Pts',(-9.41218877466708,15.2557271980297,5.24899452385311));
#59266=CARTESIAN_POINT('Ctrl Pts',(-6.66539017469168,15.834951382638,5.09199439650085));
#59267=CARTESIAN_POINT('Ctrl Pts',(-4.66696070971034,13.863470166724,4.9349942691486));
#59268=CARTESIAN_POINT('Ctrl Pts',(-5.20901029900842,11.1089874665202,4.77799414179634));
#59269=CARTESIAN_POINT('Ctrl Pts',(-7.8052841019297,10.0417525531808,4.62099401444409));
#59270=CARTESIAN_POINT('Ctrl Pts',(-10.128057595771,11.6182209055488,4.46399388709184));
#59271=CARTESIAN_POINT('Ctrl Pts',(-10.093735767433,14.4258233247707,4.30699375973958));
#59272=CARTESIAN_POINT('Ctrl Pts',(-7.73454710646218,15.9448696981551,4.14999363238733));
#59273=CARTESIAN_POINT('Ctrl Pts',(-5.16315153543426,14.8173229408266,3.99299350503507));
#59274=CARTESIAN_POINT('Ctrl Pts',(-4.69098902991507,12.045960940047,3.83599337768282));
#59275=CARTESIAN_POINT('Ctrl Pts',(-6.05008049550023,10.7720932116963,3.73132662611465));
#59276=CARTESIAN_POINT('Ctrl Pts',(-6.84980000202491,10.5582942547315,3.67899325033057));
#59277=CARTESIAN_POINT('Ctrl Pts',(-5.44566844965789,14.7468063779934,12.1070022498898));
#59278=CARTESIAN_POINT('Ctrl Pts',(-4.86812015246569,14.0713004658265,12.0546688741057));
#59279=CARTESIAN_POINT('Ctrl Pts',(-4.44032807310083,12.1176993038908,11.9500021225376));
#59280=CARTESIAN_POINT('Ctrl Pts',(-6.54346469885977,9.95282118939152,11.7930019951853));
#59281=CARTESIAN_POINT('Ctrl Pts',(-9.50426845016806,10.5189740011564,11.6360018678331));
#59282=CARTESIAN_POINT('Ctrl Pts',(-10.6678138328376,13.2977029522207,11.4790017404808));
#59283=CARTESIAN_POINT('Ctrl Pts',(-8.99076038754082,15.8026598219827,11.3220016131285));
#59284=CARTESIAN_POINT('Ctrl Pts',(-5.97692217562184,15.7848971577712,11.1650014857763));
#59285=CARTESIAN_POINT('Ctrl Pts',(-4.32884537294989,13.2617363588805,11.008001358424));
#59286=CARTESIAN_POINT('Ctrl Pts',(-5.52437185495265,10.4950077843859,10.8510012310718));
#59287=CARTESIAN_POINT('Ctrl Pts',(-8.49146381092469,9.96602748253219,10.6940011037195));
#59288=CARTESIAN_POINT('Ctrl Pts',(-10.5695002659417,12.1489511132149,10.5370009763673));
#59289=CARTESIAN_POINT('Ctrl Pts',(-9.89508658439861,15.0864252137885,10.380000849015));
#59290=CARTESIAN_POINT('Ctrl Pts',(-7.07297568330216,16.144339968164,10.2230007216628));
#59291=CARTESIAN_POINT('Ctrl Pts',(-4.63378163576147,14.3740779132334,10.0660005943105));
#59292=CARTESIAN_POINT('Ctrl Pts',(-4.76475306606344,11.3630373167398,9.90900046695826));
#59293=CARTESIAN_POINT('Ctrl Pts',(-7.34844667640581,9.81125365971957,9.75200033960601));
#59294=CARTESIAN_POINT('Ctrl Pts',(-10.068039598996,11.1102229164483,9.59500021225375));
#59295=CARTESIAN_POINT('Ctrl Pts',(-10.4848467800654,14.0951485887035,9.43800008490151));
#59296=CARTESIAN_POINT('Ctrl Pts',(-8.22511321630987,16.0894183231763,9.28099995754925));
#59297=CARTESIAN_POINT('Ctrl Pts',(-5.31516367599608,15.3047517599283,9.12399983019699));
#59298=CARTESIAN_POINT('Ctrl Pts',(-4.36437782731425,12.4447667074727,8.96699970284474));
#59299=CARTESIAN_POINT('Ctrl Pts',(-6.22533446291578,10.0740393155813,8.80999957549249));
#59300=CARTESIAN_POINT('Ctrl Pts',(-9.22929591409124,10.3184235210999,8.65299944814023));
#59301=CARTESIAN_POINT('Ctrl Pts',(-10.6825811290368,12.9587776927019,8.49599932078798));
#59302=CARTESIAN_POINT('Ctrl Pts',(-9.28201531326903,15.6274708987809,8.33899919343573));
#59303=CARTESIAN_POINT('Ctrl Pts',(-6.2834992701754,15.9314603471809,8.18199906608347));
#59304=CARTESIAN_POINT('Ctrl Pts',(-4.37583110219086,13.5981557789132,8.02499893873123));
#59305=CARTESIAN_POINT('Ctrl Pts',(-5.26963515659132,10.7198537875612,7.86799881137897));
#59306=CARTESIAN_POINT('Ctrl Pts',(-8.16342876362473,9.87755538002796,7.71099868402671));
#59307=CARTESIAN_POINT('Ctrl Pts',(-10.4623194328887,11.8265576212272,7.55399855667447));
#59308=CARTESIAN_POINT('Ctrl Pts',(-10.1048698490028,14.8191715000043,7.39699842932221));
#59309=CARTESIAN_POINT('Ctrl Pts',(-7.4116084785376,16.1718914480481,7.23999830196995));
#59310=CARTESIAN_POINT('Ctrl Pts',(-4.79760863920515,14.6717204977811,7.0829981746177));
#59311=CARTESIAN_POINT('Ctrl Pts',(-4.60686904722592,11.6638763571539,6.92599804726545));
#59312=CARTESIAN_POINT('Ctrl Pts',(-7.01042775842265,9.84552167443846,6.7689979199132));
#59313=CARTESIAN_POINT('Ctrl Pts',(-9.85299055159733,10.8471926331423,6.61199779256093));
#59314=CARTESIAN_POINT('Ctrl Pts',(-10.585604229252,13.770681089133,6.4549976652087));
#59315=CARTESIAN_POINT('Ctrl Pts',(-8.55132682499211,15.9944672608673,6.29799753785643));
#59316=CARTESIAN_POINT('Ctrl Pts',(-5.57431489867653,15.5244600427274,6.14099741050419));
#59317=CARTESIAN_POINT('Ctrl Pts',(-4.32408263542585,12.7821208080144,5.98399728315193));
#59318=CARTESIAN_POINT('Ctrl Pts',(-5.92172719634629,10.2265287344922,5.82699715579967));
#59319=CARTESIAN_POINT('Ctrl Pts',(-8.93462166631621,10.149313078634,5.66999702844742));
#59320=CARTESIAN_POINT('Ctrl Pts',(-10.6610819284076,12.61970343828,5.51299690109516));
#59321=CARTESIAN_POINT('Ctrl Pts',(-9.55296030180576,15.4224974667542,5.35599677374291));
#59322=CARTESIAN_POINT('Ctrl Pts',(-6.60394786249421,16.0443629816032,5.19899664639066));
#59323=CARTESIAN_POINT('Ctrl Pts',(-4.45839800260659,13.927745247179,5.04199651903841));
#59324=CARTESIAN_POINT('Ctrl Pts',(-5.04035220251703,10.9704830194925,4.88499639168615));
#59325=CARTESIAN_POINT('Ctrl Pts',(-7.82775850916875,9.82468039853088,4.7279962643339));
#59326=CARTESIAN_POINT('Ctrl Pts',(-10.3215299589949,11.5172052095439,4.57099613698165));
#59327=CARTESIAN_POINT('Ctrl Pts',(-10.2846814260484,14.53149772411,4.41399600962939));
#59328=CARTESIAN_POINT('Ctrl Pts',(-7.75181399705376,16.1623732644724,4.25699588227714));
#59329=CARTESIAN_POINT('Ctrl Pts',(-4.99111740815211,14.9518187617518,4.09999575492489));
#59330=CARTESIAN_POINT('Ctrl Pts',(-4.48419523986314,11.9764346130167,3.94299562757263));
#59331=CARTESIAN_POINT('Ctrl Pts',(-5.94334031085913,10.6087872809636,3.83832887600446));
#59332=CARTESIAN_POINT('Ctrl Pts',(-6.80193357383899,10.379248870828,3.78599550022038));
#59333=CARTESIAN_POINT('Ctrl Pts',(-5.30480289598085,14.8672444958453,12.2140044997796));
#59334=CARTESIAN_POINT('Ctrl Pts',(-4.68765210100993,14.1454191303684,12.1616711239955));
#59335=CARTESIAN_POINT('Ctrl Pts',(-4.23052631058544,12.0578594994142,12.0570043724274));
#59336=CARTESIAN_POINT('Ctrl Pts',(-6.47787505497571,9.74453565122039,11.9000042450751));
#59337=CARTESIAN_POINT('Ctrl Pts',(-9.64170117610916,10.3495095721105,11.7430041177229));
#59338=CARTESIAN_POINT('Ctrl Pts',(-10.8850308879103,13.3187760204667,11.5860039903706));
#59339=CARTESIAN_POINT('Ctrl Pts',(-9.09298185581149,15.9954978306723,11.4290038630184));
#59340=CARTESIAN_POINT('Ctrl Pts',(-5.87248470008946,15.9765171802363,11.2720037356661));
#59341=CARTESIAN_POINT('Ctrl Pts',(-4.11139923955409,13.2803431971336,11.1150036083138));
#59342=CARTESIAN_POINT('Ctrl Pts',(-5.38890299528115,10.3238999913978,10.9580034809616));
#59343=CARTESIAN_POINT('Ctrl Pts',(-8.55944850339236,9.75864750013418,10.8010033536093));
#59344=CARTESIAN_POINT('Ctrl Pts',(-10.7799759578531,12.091254245901,10.6440032262571));
#59345=CARTESIAN_POINT('Ctrl Pts',(-10.0593177172747,15.230151001703,10.4870030989048));
#59346=CARTESIAN_POINT('Ctrl Pts',(-7.04369461774331,16.3606069910088,10.3300029715526));
#59347=CARTESIAN_POINT('Ctrl Pts',(-4.43724498773573,14.4689580331317,10.1730028442003));
#59348=CARTESIAN_POINT('Ctrl Pts',(-4.57719713151714,11.2514503253782,10.0160027168481));
#59349=CARTESIAN_POINT('Ctrl Pts',(-7.33805466210989,9.59326083333269,9.85900258949581));
#59350=CARTESIAN_POINT('Ctrl Pts',(-10.2441301233891,10.9813004368261,9.70200246214358));
#59351=CARTESIAN_POINT('Ctrl Pts',(-10.689517780832,14.1709025194869,9.5450023347913));
#59352=CARTESIAN_POINT('Ctrl Pts',(-8.27483424341331,16.3019193677744,9.38800220743907));
#59353=CARTESIAN_POINT('Ctrl Pts',(-5.16534940749437,15.463448203285,9.2310020800868));
#59354=CARTESIAN_POINT('Ctrl Pts',(-4.14936815499344,12.4073539211118,9.07400195273456));
#59355=CARTESIAN_POINT('Ctrl Pts',(-6.13793062267174,9.87406570664018,8.9170018253823));
#59356=CARTESIAN_POINT('Ctrl Pts',(-9.34787376797726,10.1352073418028,8.76000169803005));
#59357=CARTESIAN_POINT('Ctrl Pts',(-10.9008107778922,12.9566106494239,8.6030015706778));
#59358=CARTESIAN_POINT('Ctrl Pts',(-9.40420813736444,15.8082961996578,8.44600144332554));
#59359=CARTESIAN_POINT('Ctrl Pts',(-6.20008379187702,16.1331302103455,8.28900131597328));
#59360=CARTESIAN_POINT('Ctrl Pts',(-4.16160678114728,13.6398309032289,8.13200118862104));
#59361=CARTESIAN_POINT('Ctrl Pts',(-5.1166989966437,10.564163689309,7.97500106126877));
#59362=CARTESIAN_POINT('Ctrl Pts',(-8.20892008662842,9.66410886387002,7.81800093391653));
#59363=CARTESIAN_POINT('Ctrl Pts',(-10.6654457330288,11.7467542260049,7.66100080656427));
#59364=CARTESIAN_POINT('Ctrl Pts',(-10.2834858243429,14.9445716956558,7.50400067921202));
#59365=CARTESIAN_POINT('Ctrl Pts',(-7.40554747022126,16.3900476763952,7.34700055185976));
#59366=CARTESIAN_POINT('Ctrl Pts',(-4.61230561193723,14.7870099753915,7.19000042450751));
#59367=CARTESIAN_POINT('Ctrl Pts',(-4.40848700248986,11.5729179045444,7.03300029715526));
#59368=CARTESIAN_POINT('Ctrl Pts',(-6.97685778045915,9.6298786064759,6.876000169803));
#59369=CARTESIAN_POINT('Ctrl Pts',(-10.0143351586995,10.7002341619658,6.71900004245076));
#59370=CARTESIAN_POINT('Ctrl Pts',(-10.7971841702354,13.8241862772684,6.5619999150985));
#59371=CARTESIAN_POINT('Ctrl Pts',(-8.62341632547871,16.2004575093079,6.40499978774625));
#59372=CARTESIAN_POINT('Ctrl Pts',(-5.44227063446788,15.6982218872355,6.24799966039399));
#59373=CARTESIAN_POINT('Ctrl Pts',(-4.10630992102698,12.7678403987764,6.09099953304174));
#59374=CARTESIAN_POINT('Ctrl Pts',(-5.81350500002991,10.0370113279208,5.93399940568948));
#59375=CARTESIAN_POINT('Ctrl Pts',(-9.03299370139936,9.95450099306433,5.77699927833723));
#59376=CARTESIAN_POINT('Ctrl Pts',(-10.877837376665,12.5942860668946,5.61999915098498));
#59377=CARTESIAN_POINT('Ctrl Pts',(-9.69373182894443,15.5892677354788,5.46299902363273));
#59378=CARTESIAN_POINT('Ctrl Pts',(-6.54250555029675,16.2537745805684,5.30599889628047));
#59379=CARTESIAN_POINT('Ctrl Pts',(-4.24983529550283,13.9920203276339,5.14899876892821));
#59380=CARTESIAN_POINT('Ctrl Pts',(-4.87169410602564,10.8319785724647,4.99199864157597));
#59381=CARTESIAN_POINT('Ctrl Pts',(-7.85023291640778,9.60760824388092,4.83499851422371));
#59382=CARTESIAN_POINT('Ctrl Pts',(-10.5150023222189,11.416189513539,4.67799838687146));
#59383=CARTESIAN_POINT('Ctrl Pts',(-10.4756270846638,14.6371721234493,4.52099825951921));
#59384=CARTESIAN_POINT('Ctrl Pts',(-7.76908088764536,16.3798768307898,4.36399813216695));
#59385=CARTESIAN_POINT('Ctrl Pts',(-4.81908328086994,15.086314582677,4.2069980048147));
#59386=CARTESIAN_POINT('Ctrl Pts',(-4.27740144981121,11.9069082859864,4.04999787746244));
#59387=CARTESIAN_POINT('Ctrl Pts',(-5.83660012621804,10.4454813502308,3.94533112589427));
#59388=CARTESIAN_POINT('Ctrl Pts',(-6.75406714565307,10.2002034869244,3.89299775011019));
#59389=CARTESIAN_POINT('Ctrl Pts',(-5.16393734230382,14.9876826136972,12.3210067496694));
#59390=CARTESIAN_POINT('Ctrl Pts',(-4.50718404955416,14.2195377949102,12.2686733738853));
#59391=CARTESIAN_POINT('Ctrl Pts',(-4.02072454807007,11.9980196949375,12.1640066223172));
#59392=CARTESIAN_POINT('Ctrl Pts',(-6.41228541109164,9.53625011304927,12.0070064949649));
#59393=CARTESIAN_POINT('Ctrl Pts',(-9.77913390205027,10.1800451430645,11.8500063676127));
#59394=CARTESIAN_POINT('Ctrl Pts',(-11.1022479429831,13.3398490887126,11.6930062402604));
#59395=CARTESIAN_POINT('Ctrl Pts',(-9.19520332408216,16.188335839362,11.5360061129082));
#59396=CARTESIAN_POINT('Ctrl Pts',(-5.76804722455709,16.1681372027015,11.3790059855559));
#59397=CARTESIAN_POINT('Ctrl Pts',(-3.89395310615829,13.2989500353867,11.2220058582037));
#59398=CARTESIAN_POINT('Ctrl Pts',(-5.25343413560966,10.1527921984098,11.0650057308514));
#59399=CARTESIAN_POINT('Ctrl Pts',(-8.62743319586002,9.55126751773617,10.9080056034992));
#59400=CARTESIAN_POINT('Ctrl Pts',(-10.9904516497645,12.0335573785871,10.7510054761469));
#59401=CARTESIAN_POINT('Ctrl Pts',(-10.2235488501508,15.3738767896174,10.5940053487946));
#59402=CARTESIAN_POINT('Ctrl Pts',(-7.01441355218445,16.5768740138536,10.4370052214424));
#59403=CARTESIAN_POINT('Ctrl Pts',(-4.24070833971001,14.56383815303,10.2800050940901));
#59404=CARTESIAN_POINT('Ctrl Pts',(-4.38964119697082,11.1398633340167,10.1230049667379));
#59405=CARTESIAN_POINT('Ctrl Pts',(-7.32766264781398,9.3752680069458,9.96600483938563));
#59406=CARTESIAN_POINT('Ctrl Pts',(-10.4202206477823,10.8523779572038,9.80900471203337));
#59407=CARTESIAN_POINT('Ctrl Pts',(-10.8941887815987,14.2466564502702,9.65200458468113));
#59408=CARTESIAN_POINT('Ctrl Pts',(-8.32455527051676,16.5144204123725,9.49500445732887));
#59409=CARTESIAN_POINT('Ctrl Pts',(-5.01553513899265,15.6221446466417,9.33800432997661));
#59410=CARTESIAN_POINT('Ctrl Pts',(-3.93435848267263,12.3699411347509,9.18100420262437));
#59411=CARTESIAN_POINT('Ctrl Pts',(-6.0505267824277,9.67409209769908,9.02400407527211));
#59412=CARTESIAN_POINT('Ctrl Pts',(-9.46645162186327,9.95199116250562,8.86700394791985));
#59413=CARTESIAN_POINT('Ctrl Pts',(-11.1190404267477,12.9544436061459,8.71000382056761));
#59414=CARTESIAN_POINT('Ctrl Pts',(-9.52640096145984,15.9891215005347,8.55300369321535));
#59415=CARTESIAN_POINT('Ctrl Pts',(-6.11666831357863,16.3348000735102,8.3960035658631));
#59416=CARTESIAN_POINT('Ctrl Pts',(-3.9473824601037,13.6815060275445,8.23900343851085));
#59417=CARTESIAN_POINT('Ctrl Pts',(-4.9637628366961,10.4084735910568,8.08200331115859));
#59418=CARTESIAN_POINT('Ctrl Pts',(-8.25441140963209,9.45066234771208,7.92500318380633));
#59419=CARTESIAN_POINT('Ctrl Pts',(-10.8685720331689,11.6669508307826,7.76800305645408));
#59420=CARTESIAN_POINT('Ctrl Pts',(-10.4621017996831,15.0699718913073,7.61100292910183));
#59421=CARTESIAN_POINT('Ctrl Pts',(-7.39948646190492,16.6082039047423,7.45400280174958));
#59422=CARTESIAN_POINT('Ctrl Pts',(-4.42700258466931,14.902299453002,7.29700267439732));
#59423=CARTESIAN_POINT('Ctrl Pts',(-4.21010495775379,11.4819594519348,7.14000254704507));
#59424=CARTESIAN_POINT('Ctrl Pts',(-6.94328780249567,9.41423553851335,6.98300241969282));
#59425=CARTESIAN_POINT('Ctrl Pts',(-10.1756797658017,10.5532756907892,6.82600229234056));
#59426=CARTESIAN_POINT('Ctrl Pts',(-11.0087641112188,13.8776914654038,6.66900216498831));
#59427=CARTESIAN_POINT('Ctrl Pts',(-8.69550582596531,16.4064477577484,6.51200203763606));
#59428=CARTESIAN_POINT('Ctrl Pts',(-5.31022637025923,15.8719837317436,6.3550019102838));
#59429=CARTESIAN_POINT('Ctrl Pts',(-3.88853720662811,12.7535599895385,6.19800178293155));
#59430=CARTESIAN_POINT('Ctrl Pts',(-5.70528280371351,9.84749392134933,6.04100165557929));
#59431=CARTESIAN_POINT('Ctrl Pts',(-9.13136573648253,9.75968890749465,5.88400152822705));
#59432=CARTESIAN_POINT('Ctrl Pts',(-11.0945928249223,12.5688686955092,5.72700140087479));
#59433=CARTESIAN_POINT('Ctrl Pts',(-9.83450335608313,15.7560380042034,5.57000127352253));
#59434=CARTESIAN_POINT('Ctrl Pts',(-6.48106323809927,16.4631861795336,5.41300114617029));
#59435=CARTESIAN_POINT('Ctrl Pts',(-4.04127258839909,14.0562954080889,5.25600101881802));
#59436=CARTESIAN_POINT('Ctrl Pts',(-4.70303600953422,10.693474125437,5.09900089146578));
#59437=CARTESIAN_POINT('Ctrl Pts',(-7.87270732364685,9.390536089231,4.94200076411351));
#59438=CARTESIAN_POINT('Ctrl Pts',(-10.7084746854428,11.3151738175341,4.78500063676127));
#59439=CARTESIAN_POINT('Ctrl Pts',(-10.6665727432792,14.7428465227886,4.62800050940901));
#59440=CARTESIAN_POINT('Ctrl Pts',(-7.78634777823694,16.5973803971072,4.47100038205676));
#59441=CARTESIAN_POINT('Ctrl Pts',(-4.64704915358778,15.2208104036021,4.31400025470451));
#59442=CARTESIAN_POINT('Ctrl Pts',(-4.07060765975928,11.8373819589561,4.15700012735225));
#59443=CARTESIAN_POINT('Ctrl Pts',(-5.72985994157694,10.2821754194981,4.05233337578409));
#59444=CARTESIAN_POINT('Ctrl Pts',(-6.70620071746715,10.0211581030209,4.));
#59445=CARTESIAN_POINT('Ctrl Pts',(-5.58653400333492,14.6263682601415,12.));
#59446=CARTESIAN_POINT('Ctrl Pts',(-5.52489667247578,14.5684443043264,12.));
#59447=CARTESIAN_POINT('Ctrl Pts',(-5.46662450511892,14.5073716307993,12.));
#59448=CARTESIAN_POINT('Ctrl Pts',(-5.41171706416437,14.4435345397783,12.));
#59449=CARTESIAN_POINT('Ctrl Pts',(-5.35535922399003,14.3780111697138,12.));
#59450=CARTESIAN_POINT('Ctrl Pts',(-5.30254577876706,14.3095749751578,12.));
#59451=CARTESIAN_POINT('Ctrl Pts',(-5.25330168675279,14.2385929714213,12.));
#59452=CARTESIAN_POINT('Ctrl Pts',(-5.20312907342738,14.1662725674732,12.));
#59453=CARTESIAN_POINT('Ctrl Pts',(-5.15666120991867,14.0913088475707,12.));
#59454=CARTESIAN_POINT('Ctrl Pts',(-5.1139575408143,14.0140482152174,12.));
#59455=CARTESIAN_POINT('Ctrl Pts',(-5.09461512222896,13.9790533887192,12.));
#59456=CARTESIAN_POINT('Ctrl Pts',(-5.07604545116087,13.9435868239722,12.));
#59457=CARTESIAN_POINT('Ctrl Pts',(-5.05825663128179,13.9076784991748,12.));
#59458=CARTESIAN_POINT('Ctrl Pts',(-5.04815176560046,13.887280923541,12.));
#59459=CARTESIAN_POINT('Ctrl Pts',(-5.03829889260597,13.8667407800149,12.));
#59460=CARTESIAN_POINT('Ctrl Pts',(-5.02869974914025,13.846063404379,12.));
#59461=CARTESIAN_POINT('Ctrl Pts',(-5.02048275827117,13.8283633035935,12.));
#59462=CARTESIAN_POINT('Ctrl Pts',(-5.0124495628302,13.8105575032607,12.));
#59463=CARTESIAN_POINT('Ctrl Pts',(-5.00461403680565,13.7926790499403,12.));
#59464=CARTESIAN_POINT('Ctrl Pts',(-4.96800796729637,13.7091543570335,12.));
#59465=CARTESIAN_POINT('Ctrl Pts',(-4.93566374876766,13.6239462866792,12.));
#59466=CARTESIAN_POINT('Ctrl Pts',(-4.90760852459924,13.5374526993157,12.));
#59467=CARTESIAN_POINT('Ctrl Pts',(-4.87909391214457,13.449542828816,12.));
#59468=CARTESIAN_POINT('Ctrl Pts',(-4.85500940725962,13.3603042433618,12.));
#59469=CARTESIAN_POINT('Ctrl Pts',(-4.83542253240114,13.2701175707646,12.));
#59470=CARTESIAN_POINT('Ctrl Pts',(-4.81671792757447,13.1839932613098,12.));
#59471=CARTESIAN_POINT('Ctrl Pts',(-4.80211484736484,13.0970034290495,12.));
#59472=CARTESIAN_POINT('Ctrl Pts',(-4.79171068325589,13.0094587764721,12.));
#59473=CARTESIAN_POINT('Ctrl Pts',(-4.78712088419529,12.9708384356209,12.));
#59474=CARTESIAN_POINT('Ctrl Pts',(-4.78334877386587,12.9321099201028,12.));
#59475=CARTESIAN_POINT('Ctrl Pts',(-4.78040530851934,12.893299212279,12.));
#59476=CARTESIAN_POINT('Ctrl Pts',(-4.77903296806464,12.8752043824944,12.));
#59477=CARTESIAN_POINT('Ctrl Pts',(-4.77784077628839,12.8570916824141,12.));
#59478=CARTESIAN_POINT('Ctrl Pts',(-4.77682996946529,12.8389637304098,12.));
#59479=CARTESIAN_POINT('Ctrl Pts',(-4.77585594563052,12.8214954497015,12.));
#59480=CARTESIAN_POINT('Ctrl Pts',(-4.7750503477527,12.8040101811658,12.));
#59481=CARTESIAN_POINT('Ctrl Pts',(-4.77441493543858,12.7865348449805,12.));
#59482=CARTESIAN_POINT('Ctrl Pts',(-4.77095144017316,12.6912805623749,12.));
#59483=CARTESIAN_POINT('Ctrl Pts',(-4.77253057533756,12.5961742600887,12.));
#59484=CARTESIAN_POINT('Ctrl Pts',(-4.77921451714525,12.501614579937,12.));
#59485=CARTESIAN_POINT('Ctrl Pts',(-4.78586350142022,12.4075494542275,12.));
#59486=CARTESIAN_POINT('Ctrl Pts',(-4.7975636844451,12.3140242926481,12.));
#59487=CARTESIAN_POINT('Ctrl Pts',(-4.81442425859455,12.2214137249389,12.));
#59488=CARTESIAN_POINT('Ctrl Pts',(-4.83092299201404,12.1307906503674,12.));
#59489=CARTESIAN_POINT('Ctrl Pts',(-4.85236265681916,12.0410424028911,12.));
#59490=CARTESIAN_POINT('Ctrl Pts',(-4.87846866601438,11.9524107169388,12.));
#59491=CARTESIAN_POINT('Ctrl Pts',(-4.89379308908251,11.9003832529699,12.));
#59492=CARTESIAN_POINT('Ctrl Pts',(-4.91072644984389,11.8487405476717,12.));
#59493=CARTESIAN_POINT('Ctrl Pts',(-4.92922132646561,11.7975326456,12.));
#59494=CARTESIAN_POINT('Ctrl Pts',(-4.93398223972469,11.7843508123318,12.));
#59495=CARTESIAN_POINT('Ctrl Pts',(-4.93884748217419,11.7711956209025,12.));
#59496=CARTESIAN_POINT('Ctrl Pts',(-4.94381359460063,11.7580750750315,12.));
#59497=CARTESIAN_POINT('Ctrl Pts',(-4.97686200318078,11.6707606682067,12.));
#59498=CARTESIAN_POINT('Ctrl Pts',(-5.01429316281797,11.5851876670551,12.));
#59499=CARTESIAN_POINT('Ctrl Pts',(-5.05577609967284,11.5015918684293,12.));
#59500=CARTESIAN_POINT('Ctrl Pts',(-5.09882544403038,11.414839468654,12.));
#59501=CARTESIAN_POINT('Ctrl Pts',(-5.14623844362019,11.330215691903,12.));
#59502=CARTESIAN_POINT('Ctrl Pts',(-5.19770129474244,11.2479859989681,12.));
#59503=CARTESIAN_POINT('Ctrl Pts',(-5.2497890294851,11.1647578384569,12.));
#59504=CARTESIAN_POINT('Ctrl Pts',(-5.30602595623937,11.0839814330439,12.));
#59505=CARTESIAN_POINT('Ctrl Pts',(-5.36613892032226,11.0059457826021,12.));
#59506=CARTESIAN_POINT('Ctrl Pts',(-5.4056128756235,10.9547026635106,12.));
#59507=CARTESIAN_POINT('Ctrl Pts',(-5.44675926231209,10.9046416780186,12.));
#59508=CARTESIAN_POINT('Ctrl Pts',(-5.48951145353165,10.8558504805206,12.));
#59509=CARTESIAN_POINT('Ctrl Pts',(-5.50097088386534,10.8427723361571,12.));
#59510=CARTESIAN_POINT('Ctrl Pts',(-5.5125457300662,10.8297854541688,12.));
#59511=CARTESIAN_POINT('Ctrl Pts',(-5.52423480193837,10.8168915966514,12.));
#59512=CARTESIAN_POINT('Ctrl Pts',(-5.53538763239833,10.8045892506277,12.));
#59513=CARTESIAN_POINT('Ctrl Pts',(-5.54663877351141,10.7923778862678,12.));
#59514=CARTESIAN_POINT('Ctrl Pts',(-5.55798379608792,10.7802620173577,12.));
#59515=CARTESIAN_POINT('Ctrl Pts',(-5.62980564817047,10.7035601739863,12.));
#59516=CARTESIAN_POINT('Ctrl Pts',(-5.70542329107336,10.630641847274,12.));
#59517=CARTESIAN_POINT('Ctrl Pts',(-5.78449319659024,10.5618401471187,12.));
#59518=CARTESIAN_POINT('Ctrl Pts',(-5.84379562572791,10.5102388720023,12.));
#59519=CARTESIAN_POINT('Ctrl Pts',(-5.90504126576837,10.4609534569649,12.));
#59520=CARTESIAN_POINT('Ctrl Pts',(-5.96810424452339,10.4141359861561,12.));
#59521=CARTESIAN_POINT('Ctrl Pts',(-5.99074689198795,10.39732625868,12.));
#59522=CARTESIAN_POINT('Ctrl Pts',(-6.01362396161954,10.3808348014861,12.));
#59523=CARTESIAN_POINT('Ctrl Pts',(-6.03673007192386,10.3646690702049,12.));
#59524=CARTESIAN_POINT('Ctrl Pts',(-6.05604446520068,10.351156138454,12.));
#59525=CARTESIAN_POINT('Ctrl Pts',(-6.07552143283976,10.3378692705033,12.));
#59526=CARTESIAN_POINT('Ctrl Pts',(-6.09513718668148,10.3248263089414,12.));
#59527=CARTESIAN_POINT('Ctrl Pts',(-6.18010809783264,10.2683272145418,12.));
#59528=CARTESIAN_POINT('Ctrl Pts',(-6.26775573276173,10.2163476819429,12.));
#59529=CARTESIAN_POINT('Ctrl Pts',(-6.35779277794461,10.1691997545039,12.));
#59530=CARTESIAN_POINT('Ctrl Pts',(-6.4298686728608,10.131457189133,12.));
#59531=CARTESIAN_POINT('Ctrl Pts',(-6.50347672461637,10.0968111469865,12.));
#59532=CARTESIAN_POINT('Ctrl Pts',(-6.57848633664494,10.0654390261441,12.));
#59533=CARTESIAN_POINT('Ctrl Pts',(-6.61998971216275,10.0480805986452,12.));
#59534=CARTESIAN_POINT('Ctrl Pts',(-6.6619224176942,10.0317247798523,12.));
#59535=CARTESIAN_POINT('Ctrl Pts',(-6.70425100699966,10.0163623331919,12.));
#59536=CARTESIAN_POINT('Ctrl Pts',(-10.0166112816083,12.988245230306,10.387416697508));
#59537=CARTESIAN_POINT('Ctrl Pts',(-10.0185036739199,12.7635802052187,10.4016107071645));
#59538=CARTESIAN_POINT('Ctrl Pts',(-9.99083720988162,12.539373330507,10.415804716821));
#59539=CARTESIAN_POINT('Ctrl Pts',(-9.93173881101679,12.3237831354866,10.4299987264775));
#59540=CARTESIAN_POINT('Ctrl Pts',(-9.71384275550587,11.5289011419959,10.4823321022615));
#59541=CARTESIAN_POINT('Ctrl Pts',(-9.06866093698144,10.8511543034631,10.5346654780456));
#59542=CARTESIAN_POINT('Ctrl Pts',(-8.28546362708042,10.5943989029373,10.5869988538297));
#59543=CARTESIAN_POINT('Ctrl Pts',(-7.50226631717939,10.3376435024115,10.6393322296138));
#59544=CARTESIAN_POINT('Ctrl Pts',(-6.58105351590176,10.5018795398927,10.6916656053979));
#59545=CARTESIAN_POINT('Ctrl Pts',(-5.93485558054988,11.0134998825089,10.743998981182));
#59546=CARTESIAN_POINT('Ctrl Pts',(-5.28865764519799,11.5251202251251,10.796332356966));
#59547=CARTESIAN_POINT('Ctrl Pts',(-4.91747457577184,12.3841248728762,10.8486657327501));
#59548=CARTESIAN_POINT('Ctrl Pts',(-4.98772773186019,13.2053184658649,10.9009991085342));
#59549=CARTESIAN_POINT('Ctrl Pts',(-5.05798088794854,14.0265120588536,10.9533324843183));
#59550=CARTESIAN_POINT('Ctrl Pts',(-5.56967026955137,14.8098945970798,11.0056658601024));
#59551=CARTESIAN_POINT('Ctrl Pts',(-6.29337817170545,15.2043433125241,11.0579992358865));
#59552=CARTESIAN_POINT('Ctrl Pts',(-7.01708607385953,15.5987920279684,11.1103326116706));
#59553=CARTESIAN_POINT('Ctrl Pts',(-7.95281249656485,15.6043069206307,11.1626659874546));
#59554=CARTESIAN_POINT('Ctrl Pts',(-8.68101868433327,15.2181990454088,11.2149993632387));
#59555=CARTESIAN_POINT('Ctrl Pts',(-9.4092248721017,14.8320911701869,11.2673327390228));
#59556=CARTESIAN_POINT('Ctrl Pts',(-9.92991082493323,14.0543605270808,11.3196661148069));
#59557=CARTESIAN_POINT('Ctrl Pts',(-10.0096269590927,13.2341299632324,11.371999490591));
#59558=CARTESIAN_POINT('Ctrl Pts',(-10.0174549790803,13.1535843959402,11.3771385595633));
#59559=CARTESIAN_POINT('Ctrl Pts',(-10.0210307346825,13.0726290026425,11.3822776285357));
#59560=CARTESIAN_POINT('Ctrl Pts',(-10.020507596494,12.9916292754481,11.387416697508));
#59561=CARTESIAN_POINT('Ctrl Pts',(-8.29379928253292,10.0211581030209,12.));
#59562=CARTESIAN_POINT('Ctrl Pts',(-9.27014005842312,10.2821754194981,11.9476666242159));
#59563=CARTESIAN_POINT('Ctrl Pts',(-10.9293920526294,11.8373837255142,11.8429998726477));
#59564=CARTESIAN_POINT('Ctrl Pts',(-10.3529510979028,15.2208095229378,11.6859997452955));
#59565=CARTESIAN_POINT('Ctrl Pts',(-7.21365218567195,16.5973810760335,11.5289996179432));
#59566=CARTESIAN_POINT('Ctrl Pts',(-4.33342713054201,14.7428462583649,11.371999490591));
#59567=CARTESIAN_POINT('Ctrl Pts',(-4.29152522806557,11.3151739482887,11.2149993632387));
#59568=CARTESIAN_POINT('Ctrl Pts',(-7.12729264284838,9.39053585671186,11.0579992358865));
#59569=CARTESIAN_POINT('Ctrl Pts',(-10.2969641018483,10.6934741072896,10.9009991085342));
#59570=CARTESIAN_POINT('Ctrl Pts',(-10.9587275214881,14.0562954105675,10.743998981182));
#59571=CARTESIAN_POINT('Ctrl Pts',(-8.5189368031419,16.4631863186891,10.5869988538297));
#59572=CARTESIAN_POINT('Ctrl Pts',(-5.16549655959477,15.7560380892136,10.4299987264775));
#59573=CARTESIAN_POINT('Ctrl Pts',(-3.90540705298465,12.5688686867556,10.2729985991252));
#59574=CARTESIAN_POINT('Ctrl Pts',(-5.86863420589283,9.75968879265402,10.115998471773));
#59575=CARTESIAN_POINT('Ctrl Pts',(-9.29471725902464,9.84749381445728,9.9589983444207));
#59576=CARTESIAN_POINT('Ctrl Pts',(-11.1114629177913,12.7535599804133,9.80199821706845));
#59577=CARTESIAN_POINT('Ctrl Pts',(-9.68977370564798,15.8719838318464,9.64499808971619));
#59578=CARTESIAN_POINT('Ctrl Pts',(-6.30449413259093,16.4064478755407,9.48799796236394));
#59579=CARTESIAN_POINT('Ctrl Pts',(-3.99123576757957,13.8776914962184,9.3309978350117));
#59580=CARTESIAN_POINT('Ctrl Pts',(-4.82432014168349,10.5532756064786,9.17399770765943));
#59581=CARTESIAN_POINT('Ctrl Pts',(-8.05671221676616,9.41423541495656,9.0169975803072));
#59582=CARTESIAN_POINT('Ctrl Pts',(-10.7898951559407,11.481959399778,8.85999745295492));
#59583=CARTESIAN_POINT('Ctrl Pts',(-10.572997521546,14.902299519094,8.70299732560269));
#59584=CARTESIAN_POINT('Ctrl Pts',(-7.60051354156566,16.6082040297755,8.54599719825042));
#59585=CARTESIAN_POINT('Ctrl Pts',(-4.53789809794217,15.0699719631857,8.38899707089818));
#59586=CARTESIAN_POINT('Ctrl Pts',(-4.1314278504052,11.6669507850401,8.23199694354592));
#59587=CARTESIAN_POINT('Ctrl Pts',(-6.74558856429446,9.45066222537301,8.07499681619367));
#59588=CARTESIAN_POINT('Ctrl Pts',(-10.0362372509614,10.4084735018199,7.91799668884141));
#59589=CARTESIAN_POINT('Ctrl Pts',(-11.0526176626825,13.6815060514322,7.76099656148917));
#59590=CARTESIAN_POINT('Ctrl Pts',(-8.88333173423194,16.3348001890992,7.6039964341369));
#59591=CARTESIAN_POINT('Ctrl Pts',(-5.47359896850368,15.9891216041795,7.44699630678466));
#59592=CARTESIAN_POINT('Ctrl Pts',(-3.88095944817013,12.9544436048999,7.28999617943239));
#59593=CARTESIAN_POINT('Ctrl Pts',(-5.53354831017302,9.95199105749957,7.13299605208015));
#59594=CARTESIAN_POINT('Ctrl Pts',(-8.9494732676674,9.67409198306777,6.97599592472789));
#59595=CARTESIAN_POINT('Ctrl Pts',(-11.0656416405671,12.3699411133323,6.81899579737564));
#59596=CARTESIAN_POINT('Ctrl Pts',(-9.98446494686864,15.6221447375545,6.66199567002338));
#59597=CARTESIAN_POINT('Ctrl Pts',(-6.67544470099851,16.5144205342573,6.50499554267113));
#59598=CARTESIAN_POINT('Ctrl Pts',(-4.10581110106408,14.2466564935293,6.34799541531888));
#59599=CARTESIAN_POINT('Ctrl Pts',(-4.57977925134152,10.8523778836063,6.19099528796662));
#59600=CARTESIAN_POINT('Ctrl Pts',(-7.67233735803906,9.3752678814539,6.03399516061438));
#59601=CARTESIAN_POINT('Ctrl Pts',(-10.6103589107324,11.1398632710606,5.87699503326211));
#59602=CARTESIAN_POINT('Ctrl Pts',(-10.7592917725406,14.5638382055826,5.71999490590987));
#59603=CARTESIAN_POINT('Ctrl Pts',(-7.98558646537732,16.576874141135,5.56299477855761));
#59604=CARTESIAN_POINT('Ctrl Pts',(-4.77645105419042,15.3738768659897,5.40599465120536));
#59605=CARTESIAN_POINT('Ctrl Pts',(-4.00954823259222,12.0335573562934,5.24899452385311));
#59606=CARTESIAN_POINT('Ctrl Pts',(-6.37256675930357,9.55126737969704,5.09199439650085));
#59607=CARTESIAN_POINT('Ctrl Pts',(-9.74656595354479,10.1527921341227,4.9349942691486));
#59608=CARTESIAN_POINT('Ctrl Pts',(-11.1060469959117,13.2989499872504,4.77799414179634));
#59609=CARTESIAN_POINT('Ctrl Pts',(-9.2319528795399,16.1681374132995,4.62099401444409));
#59610=CARTESIAN_POINT('Ctrl Pts',(-5.80479653057489,16.1883357805992,4.46399388709183));
#59611=CARTESIAN_POINT('Ctrl Pts',(-3.89775210281319,13.3398493780975,4.30699375973959));
#59612=CARTESIAN_POINT('Ctrl Pts',(-5.22086568363505,10.1800446040033,4.14999363238733));
#59613=CARTESIAN_POINT('Ctrl Pts',(-8.58771529500726,9.53625069635182,3.99299350503508));
#59614=CARTESIAN_POINT('Ctrl Pts',(-10.9792742142571,11.9980184020288,3.83599337768282));
#59615=CARTESIAN_POINT('Ctrl Pts',(-10.4928159504458,14.2195377949103,3.73132662611465));
#59616=CARTESIAN_POINT('Ctrl Pts',(-9.83606265769613,14.9876826136973,3.67899325033057));
#59617=CARTESIAN_POINT('Ctrl Pts',(-8.245932854347,10.2002034869244,12.1070022498898));
#59618=CARTESIAN_POINT('Ctrl Pts',(-9.16339987378202,10.4454813502309,12.0546688741057));
#59619=CARTESIAN_POINT('Ctrl Pts',(-10.7225982799205,11.9069099460203,11.9500021225376));
#59620=CARTESIAN_POINT('Ctrl Pts',(-10.1809169554557,15.086313755117,11.7930019951853));
#59621=CARTESIAN_POINT('Ctrl Pts',(-7.23091907843985,16.3798774687766,11.636001867833));
#59622=CARTESIAN_POINT('Ctrl Pts',(-4.52437279676603,14.6371718749705,11.4790017404808));
#59623=CARTESIAN_POINT('Ctrl Pts',(-4.48499759650499,11.4161896364091,11.3220016131285));
#59624=CARTESIAN_POINT('Ctrl Pts',(-7.14976705210776,9.60760802538281,11.1650014857763));
#59625=CARTESIAN_POINT('Ctrl Pts',(-10.1283059986405,10.8319785554116,11.008001358424));
#59626=CARTESIAN_POINT('Ctrl Pts',(-10.7501648077581,13.992020329963,10.8510012310718));
#59627=CARTESIAN_POINT('Ctrl Pts',(-8.45749448845756,16.2537747113328,10.6940011037195));
#59628=CARTESIAN_POINT('Ctrl Pts',(-5.30626809181812,15.5892678153629,10.5370009763673));
#59629=CARTESIAN_POINT('Ctrl Pts',(-4.12216250860425,12.5942860586688,10.380000849015));
#59630=CARTESIAN_POINT('Ctrl Pts',(-5.96700624445078,9.95450088514863,10.2230007216628));
#59631=CARTESIAN_POINT('Ctrl Pts',(-9.18649505892511,10.0370112274744,10.0660005943105));
#59632=CARTESIAN_POINT('Ctrl Pts',(-10.8936901958899,12.7678403902015,9.90900046695827));
#59633=CARTESIAN_POINT('Ctrl Pts',(-9.5577294368621,15.6982219813021,9.752000339606));
#59634=CARTESIAN_POINT('Ctrl Pts',(-6.3765836355766,16.2004576199972,9.59500021225376));
#59635=CARTESIAN_POINT('Ctrl Pts',(-4.20281571587151,13.8241863062249,9.4380000849015));
#59636=CARTESIAN_POINT('Ctrl Pts',(-4.98566475436435,10.7002340827391,9.28099995754925));
#59637=CARTESIAN_POINT('Ctrl Pts',(-8.02314223764118,9.62987849036962,9.123999830197));
#59638=CARTESIAN_POINT('Ctrl Pts',(-10.5915131043488,11.5729178555327,8.96699970284474));
#59639=CARTESIAN_POINT('Ctrl Pts',(-10.3876944878733,14.7870100374982,8.80999957549249));
#59640=CARTESIAN_POINT('Ctrl Pts',(-7.59445253304005,16.3900477938888,8.65299944814024));
#59641=CARTESIAN_POINT('Ctrl Pts',(-4.71651407945554,14.9445717631999,8.49599932078798));
#59642=CARTESIAN_POINT('Ctrl Pts',(-4.33455415756585,11.7467541830206,8.33899919343573));
#59643=CARTESIAN_POINT('Ctrl Pts',(-6.79107988887037,9.66410874890807,8.18199906608347));
#59644=CARTESIAN_POINT('Ctrl Pts',(-9.88330108572798,10.5641636054531,8.02499893873122));
#59645=CARTESIAN_POINT('Ctrl Pts',(-10.8383933342348,13.6398309256761,7.86799881137897));
#59646=CARTESIAN_POINT('Ctrl Pts',(-8.79991625305057,16.1331303189645,7.71099868402671));
#59647=CARTESIAN_POINT('Ctrl Pts',(-5.59579179682231,15.8082962970528,7.55399855667447));
#59648=CARTESIAN_POINT('Ctrl Pts',(-4.09918910456809,12.956610648253,7.39699842932221));
#59649=CARTESIAN_POINT('Ctrl Pts',(-5.65212616815729,10.1352072431286,7.23999830196996));
#59650=CARTESIAN_POINT('Ctrl Pts',(-8.86206942440258,9.8740655989212,7.0829981746177));
#59651=CARTESIAN_POINT('Ctrl Pts',(-10.8506319608149,12.4073539009847,6.92599804726545));
#59652=CARTESIAN_POINT('Ctrl Pts',(-9.83465067318943,15.4634482887157,6.76899791991319));
#59653=CARTESIAN_POINT('Ctrl Pts',(-6.72516572981961,16.3019194823095,6.61199779256095));
#59654=CARTESIAN_POINT('Ctrl Pts',(-4.3104821089062,14.1709025601374,6.45499766520868));
#59655=CARTESIAN_POINT('Ctrl Pts',(-4.75586978181755,10.9813003676665,6.29799753785644));
#59656=CARTESIAN_POINT('Ctrl Pts',(-7.6619453433902,9.59326071540802,6.14099741050417));
#59657=CARTESIAN_POINT('Ctrl Pts',(-10.4228029696916,11.2514502662184,5.98399728315193));
#59658=CARTESIAN_POINT('Ctrl Pts',(-10.5627551177461,14.4689580825154,5.82699715579967));
#59659=CARTESIAN_POINT('Ctrl Pts',(-7.95630539875948,16.360607110615,5.66999702844743));
#59660=CARTESIAN_POINT('Ctrl Pts',(-4.94068219283476,15.23015107347,5.51299690109516));
#59661=CARTESIAN_POINT('Ctrl Pts',(-4.22002393159755,12.0912542249516,5.35599677374292));
#59662=CARTESIAN_POINT('Ctrl Pts',(-6.44055145447491,9.75864737041887,5.19899664639066));
#59663=CARTESIAN_POINT('Ctrl Pts',(-9.61109708849724,10.3238999309873,5.04199651903841));
#59664=CARTESIAN_POINT('Ctrl Pts',(-10.8886008563611,13.2803431519,4.88499639168615));
#59665=CARTESIAN_POINT('Ctrl Pts',(-9.12751539773043,15.9765173781352,4.72799626433391));
#59666=CARTESIAN_POINT('Ctrl Pts',(-5.9070180076098,15.995497775453,4.57099613698164));
#59667=CARTESIAN_POINT('Ctrl Pts',(-4.11496915512444,13.3187762924015,4.4139960096294));
#59668=CARTESIAN_POINT('Ctrl Pts',(-5.35829843455949,10.3495090655549,4.25699588227714));
#59669=CARTESIAN_POINT('Ctrl Pts',(-8.52212560854514,9.74453619934955,4.09999575492489));
#59670=CARTESIAN_POINT('Ctrl Pts',(-10.7694725263739,12.0578582844684,3.94299562757263));
#59671=CARTESIAN_POINT('Ctrl Pts',(-10.31234789899,14.1454191303684,3.83832887600446));
#59672=CARTESIAN_POINT('Ctrl Pts',(-9.6951971040191,14.8672444958454,3.78599550022038));
#59673=CARTESIAN_POINT('Ctrl Pts',(-8.19806642616107,10.379248870828,12.2140044997796));
#59674=CARTESIAN_POINT('Ctrl Pts',(-9.05665968914092,10.6087872809636,12.1616711239955));
#59675=CARTESIAN_POINT('Ctrl Pts',(-10.5158045072117,11.9764361665263,12.0570043724274));
#59676=CARTESIAN_POINT('Ctrl Pts',(-10.0088828130085,14.9518179872963,11.9000042450751));
#59677=CARTESIAN_POINT('Ctrl Pts',(-7.24818597120775,16.1623738615197,11.7430041177229));
#59678=CARTESIAN_POINT('Ctrl Pts',(-4.71531846299006,14.531497491576,11.5860039903706));
#59679=CARTESIAN_POINT('Ctrl Pts',(-4.67846996494438,11.5172053245294,11.4290038630183));
#59680=CARTESIAN_POINT('Ctrl Pts',(-7.17224146136718,9.82468019405374,11.2720037356661));
#59681=CARTESIAN_POINT('Ctrl Pts',(-9.9596478954327,10.9704830035337,11.1150036083138));
#59682=CARTESIAN_POINT('Ctrl Pts',(-10.5416020940281,13.9277452493586,10.9580034809616));
#59683=CARTESIAN_POINT('Ctrl Pts',(-8.39605217377323,16.0443631039765,10.8010033536093));
#59684=CARTESIAN_POINT('Ctrl Pts',(-5.44703962404145,15.4224975415121,10.6440032262571));
#59685=CARTESIAN_POINT('Ctrl Pts',(-4.33891796422385,12.6197034305821,10.4870030989048));
#59686=CARTESIAN_POINT('Ctrl Pts',(-6.06537828300873,10.1493129776432,10.3300029715526));
#59687=CARTESIAN_POINT('Ctrl Pts',(-9.07827285882558,10.2265286404914,10.1730028442003));
#59688=CARTESIAN_POINT('Ctrl Pts',(-10.6759174739885,12.7821207999897,10.0160027168481));
#59689=CARTESIAN_POINT('Ctrl Pts',(-9.4256851680762,15.5244601307577,9.85900258949583));
#59690=CARTESIAN_POINT('Ctrl Pts',(-6.4486731385623,15.9944673644538,9.70200246214356));
#59691=CARTESIAN_POINT('Ctrl Pts',(-4.41439566416342,13.7706811162314,9.54500233479132));
#59692=CARTESIAN_POINT('Ctrl Pts',(-5.14700936704523,10.8471925589996,9.38800220743905));
#59693=CARTESIAN_POINT('Ctrl Pts',(-7.98957225851618,9.84552156578271,9.23100208008681));
#59694=CARTESIAN_POINT('Ctrl Pts',(-10.393131052757,11.6638763112873,9.07400195273455));
#59695=CARTESIAN_POINT('Ctrl Pts',(-10.2023914542005,14.6717205559024,8.9170018253823));
#59696=CARTESIAN_POINT('Ctrl Pts',(-7.58839152451442,16.1718915580022,8.76000169803004));
#59697=CARTESIAN_POINT('Ctrl Pts',(-4.89513006096893,14.8191715632141,8.6030015706778));
#59698=CARTESIAN_POINT('Ctrl Pts',(-4.53768046472649,11.8265575810012,8.44600144332554));
#59699=CARTESIAN_POINT('Ctrl Pts',(-6.83657121344629,9.87755527244308,8.28900131597329));
#59700=CARTESIAN_POINT('Ctrl Pts',(-9.73036492049458,10.7198537090864,8.13200118862103));
#59701=CARTESIAN_POINT('Ctrl Pts',(-10.6241690057872,13.59815579992,7.97500106126879));
#59702=CARTESIAN_POINT('Ctrl Pts',(-8.71650077186918,15.9314604488298,7.81800093391652));
#59703=CARTESIAN_POINT('Ctrl Pts',(-5.71798462514094,15.6274709899262,7.66100080656428));
#59704=CARTESIAN_POINT('Ctrl Pts',(-4.31741876096606,12.9587776916062,7.50400067921201));
#59705=CARTESIAN_POINT('Ctrl Pts',(-5.77070402614152,10.3184234287576,7.34700055185978));
#59706=CARTESIAN_POINT('Ctrl Pts',(-8.7746655811378,10.0740392147746,7.19000042450751));
#59707=CARTESIAN_POINT('Ctrl Pts',(-10.6356222810626,12.4447666886372,7.03300029715527));
#59708=CARTESIAN_POINT('Ctrl Pts',(-9.68483639951025,15.304751839877,6.876000169803));
#59709=CARTESIAN_POINT('Ctrl Pts',(-6.77488675864068,16.0894184303616,6.71900004245076));
#59710=CARTESIAN_POINT('Ctrl Pts',(-4.51515311674835,14.0951486267455,6.56199991509849));
#59711=CARTESIAN_POINT('Ctrl Pts',(-4.93196031229355,11.1102228517267,6.40499978774625));
#59712=CARTESIAN_POINT('Ctrl Pts',(-7.65155332874137,9.81125354936211,6.24799966039399));
#59713=CARTESIAN_POINT('Ctrl Pts',(-10.2352470286507,11.3630372613762,6.09099953304174));
#59714=CARTESIAN_POINT('Ctrl Pts',(-10.3662184629517,14.3740779594481,5.93399940568949));
#59715=CARTESIAN_POINT('Ctrl Pts',(-7.92702433214164,16.1443400800951,5.77699927833723));
#59716=CARTESIAN_POINT('Ctrl Pts',(-5.10491333147909,15.0864252809503,5.61999915098498));
#59717=CARTESIAN_POINT('Ctrl Pts',(-4.4304996306029,12.1489510936098,5.46299902363272));
#59718=CARTESIAN_POINT('Ctrl Pts',(-6.50853614964623,9.96602736114071,5.30599889628047));
#59719=CARTESIAN_POINT('Ctrl Pts',(-9.47562822344969,10.4950077278519,5.14899876892822));
#59720=CARTESIAN_POINT('Ctrl Pts',(-10.6711547168104,13.2617363165495,4.99199864157597));
#59721=CARTESIAN_POINT('Ctrl Pts',(-9.02307791592096,15.7848973429709,4.83499851422371));
#59722=CARTESIAN_POINT('Ctrl Pts',(-6.0092394846447,15.8026597703067,4.67799838687145));
#59723=CARTESIAN_POINT('Ctrl Pts',(-4.33218620743569,13.2977032067055,4.52099825951921));
#59724=CARTESIAN_POINT('Ctrl Pts',(-5.49573118548395,10.5189735271065,4.36399813216694));
#59725=CARTESIAN_POINT('Ctrl Pts',(-8.45653592208301,9.95282170234728,4.20699800481471));
#59726=CARTESIAN_POINT('Ctrl Pts',(-10.5596708384907,12.117698166908,4.04999787746244));
#59727=CARTESIAN_POINT('Ctrl Pts',(-10.1318798475343,14.0713004658266,3.94533112589427));
#59728=CARTESIAN_POINT('Ctrl Pts',(-9.55433155034207,14.7468063779934,3.89299775011019));
#59729=CARTESIAN_POINT('Ctrl Pts',(-8.15019999797515,10.5582942547315,12.3210067496694));
#59730=CARTESIAN_POINT('Ctrl Pts',(-8.94991950449982,10.7720932116964,12.2686733738853));
#59731=CARTESIAN_POINT('Ctrl Pts',(-10.3090107345028,12.0459623870324,12.1640066223172));
#59732=CARTESIAN_POINT('Ctrl Pts',(-9.83684867056136,14.8173222194755,12.0070064949649));
#59733=CARTESIAN_POINT('Ctrl Pts',(-7.26545286397565,15.9448702542628,11.8500063676127));
#59734=CARTESIAN_POINT('Ctrl Pts',(-4.90626412921408,14.4258231081815,11.6930062402604));
#59735=CARTESIAN_POINT('Ctrl Pts',(-4.87194233338379,11.6182210126498,11.5360061129081));
#59736=CARTESIAN_POINT('Ctrl Pts',(-7.19471587062657,10.0417523627247,11.3790059855559));
#59737=CARTESIAN_POINT('Ctrl Pts',(-9.79098979222489,11.1089874516557,11.2220058582036));
#59738=CARTESIAN_POINT('Ctrl Pts',(-10.3330393802981,13.8634701687541,11.0650057308514));
#59739=CARTESIAN_POINT('Ctrl Pts',(-8.33460985908889,15.8349514966202,10.9080056034991));
#59740=CARTESIAN_POINT('Ctrl Pts',(-5.5878111562648,15.2557272676614,10.7510054761469));
#59741=CARTESIAN_POINT('Ctrl Pts',(-4.55567341984345,12.6451208024954,10.5940053487946));
#59742=CARTESIAN_POINT('Ctrl Pts',(-6.16375032156668,10.3441250701379,10.4370052214424));
#59743=CARTESIAN_POINT('Ctrl Pts',(-8.97005065872605,10.4160460535085,10.2800050940901));
#59744=CARTESIAN_POINT('Ctrl Pts',(-10.4581447520871,12.796401209778,10.1230049667379));
#59745=CARTESIAN_POINT('Ctrl Pts',(-9.29364089929031,15.3506982802133,9.96600483938563));
#59746=CARTESIAN_POINT('Ctrl Pts',(-6.52076264154797,15.7884771089103,9.80900471203338));
#59747=CARTESIAN_POINT('Ctrl Pts',(-4.62597561245536,13.7171759262378,9.65200458468112));
#59748=CARTESIAN_POINT('Ctrl Pts',(-5.3083539797261,10.9941510352601,9.49500445732887));
#59749=CARTESIAN_POINT('Ctrl Pts',(-7.95600227939119,10.0611646411958,9.33800432997662));
#59750=CARTESIAN_POINT('Ctrl Pts',(-10.1947490011651,11.7548347670419,9.18100420262436));
#59751=CARTESIAN_POINT('Ctrl Pts',(-10.0170884205278,14.5564310743066,9.02400407527211));
#59752=CARTESIAN_POINT('Ctrl Pts',(-7.5823305159888,15.9537353221155,8.86700394791986));
#59753=CARTESIAN_POINT('Ctrl Pts',(-5.07374604248231,14.6937713632283,8.71000382056761));
#59754=CARTESIAN_POINT('Ctrl Pts',(-4.74080677188713,11.9063609789818,8.55300369321535));
#59755=CARTESIAN_POINT('Ctrl Pts',(-6.88206253802222,10.0910017959781,8.3960035658631));
#59756=CARTESIAN_POINT('Ctrl Pts',(-9.57742875526118,10.8755438127196,8.23900343851084));
#59757=CARTESIAN_POINT('Ctrl Pts',(-10.4099446773395,13.5564806741639,8.0820033111586));
#59758=CARTESIAN_POINT('Ctrl Pts',(-8.63308529068779,15.7297905786951,7.92500318380633));
#59759=CARTESIAN_POINT('Ctrl Pts',(-5.84017745345957,15.4466456827995,7.7680030564541));
#59760=CARTESIAN_POINT('Ctrl Pts',(-4.53564841736402,12.9609447349594,7.61100292910181));
#59761=CARTESIAN_POINT('Ctrl Pts',(-5.88928188412577,10.5016396143867,7.45400280174959));
#59762=CARTESIAN_POINT('Ctrl Pts',(-8.687261737873,10.2740128306281,7.29700267439731));
#59763=CARTESIAN_POINT('Ctrl Pts',(-10.4206126013104,12.4821794762896,7.14000254704508));
#59764=CARTESIAN_POINT('Ctrl Pts',(-9.53502212583107,15.1460553910382,6.98300241969281));
#59765=CARTESIAN_POINT('Ctrl Pts',(-6.82460778746177,15.8769173784138,6.82600229234057));
#59766=CARTESIAN_POINT('Ctrl Pts',(-4.71982412459047,14.0193946933536,6.66900216498831));
#59767=CARTESIAN_POINT('Ctrl Pts',(-5.10805084276957,11.2391453357869,6.51200203763605));
#59768=CARTESIAN_POINT('Ctrl Pts',(-7.64116131409251,10.0292463833162,6.35500191028381));
#59769=CARTESIAN_POINT('Ctrl Pts',(-10.0476910876099,11.474624256534,6.19800178293155));
#59770=CARTESIAN_POINT('Ctrl Pts',(-10.1696818081572,14.2791978363808,6.0410016555793));
#59771=CARTESIAN_POINT('Ctrl Pts',(-7.89774326552381,15.9280730495752,5.88400152822705));
#59772=CARTESIAN_POINT('Ctrl Pts',(-5.26914447012342,14.9426994884306,5.72700140087479));
#59773=CARTESIAN_POINT('Ctrl Pts',(-4.64097532960824,12.206647962268,5.57000127352254));
#59774=CARTESIAN_POINT('Ctrl Pts',(-6.57652084481755,10.1734073518625,5.41300114617028));
#59775=CARTESIAN_POINT('Ctrl Pts',(-9.34015935840215,10.6661155247165,5.25600101881803));
#59776=CARTESIAN_POINT('Ctrl Pts',(-10.4537085772597,13.243129481199,5.09900089146578));
#59777=CARTESIAN_POINT('Ctrl Pts',(-8.91864043411149,15.5932773078066,4.94200076411352));
#59778=CARTESIAN_POINT('Ctrl Pts',(-6.11146096167962,15.6098217651605,4.78500063676127));
#59779=CARTESIAN_POINT('Ctrl Pts',(-4.54940325974693,13.2766301210095,4.62800050940902));
#59780=CARTESIAN_POINT('Ctrl Pts',(-5.63316393640839,10.6884379886581,4.47100038205676));
#59781=CARTESIAN_POINT('Ctrl Pts',(-8.39094623562089,10.161107205345,4.31400025470451));
#59782=CARTESIAN_POINT('Ctrl Pts',(-10.3498691506075,12.1775380493476,4.15700012735225));
#59783=CARTESIAN_POINT('Ctrl Pts',(-9.95141179607851,13.9971818012848,4.05233337578409));
#59784=CARTESIAN_POINT('Ctrl Pts',(-9.41346599666504,14.6263682601415,4.));
#59785=CARTESIAN_POINT('Ctrl Pts',(-10.0159019782719,12.9923925656114,11.112583302492));
#59786=CARTESIAN_POINT('Ctrl Pts',(-10.017856950592,13.2435976299952,11.0967241119451));
#59787=CARTESIAN_POINT('Ctrl Pts',(-9.98318348246503,13.4942759769916,11.0808649213983));
#59788=CARTESIAN_POINT('Ctrl Pts',(-9.90962619541772,13.7329699372154,11.0650057308514));
#59789=CARTESIAN_POINT('Ctrl Pts',(-9.66689620656173,14.5206306113761,11.0126723550673));
#59790=CARTESIAN_POINT('Ctrl Pts',(-9.00075303282531,15.1777910539982,10.9603389792832));
#59791=CARTESIAN_POINT('Ctrl Pts',(-8.20988166215309,15.409833903816,10.9080056034991));
#59792=CARTESIAN_POINT('Ctrl Pts',(-7.41901029148087,15.6418767536339,10.8556722277151));
#59793=CARTESIAN_POINT('Ctrl Pts',(-6.50341072387283,15.4488020106477,10.803338851931));
#59794=CARTESIAN_POINT('Ctrl Pts',(-5.87358798399859,14.9171635616269,10.7510054761469));
#59795=CARTESIAN_POINT('Ctrl Pts',(-5.24376524412435,14.3855251126061,10.6986721003628));
#59796=CARTESIAN_POINT('Ctrl Pts',(-4.8997193319839,13.5153229575507,10.6463387245787));
#59797=CARTESIAN_POINT('Ctrl Pts',(-4.99570919286755,12.6967225912968,10.5940053487946));
#59798=CARTESIAN_POINT('Ctrl Pts',(-5.09169905375119,11.8781222250429,10.5416719730106));
#59799=CARTESIAN_POINT('Ctrl Pts',(-5.62772468765894,11.1111236475904,10.4893385972265));
#59800=CARTESIAN_POINT('Ctrl Pts',(-6.3634542274727,10.7396111894259,10.4370052214424));
#59801=CARTESIAN_POINT('Ctrl Pts',(-7.09918376728647,10.3680987312614,10.3846718456583));
#59802=CARTESIAN_POINT('Ctrl Pts',(-8.03461721300627,10.392072392385,10.3323384698742));
#59803=CARTESIAN_POINT('Ctrl Pts',(-8.750349618093,10.800785082325,10.2800050940901));
#59804=CARTESIAN_POINT('Ctrl Pts',(-9.46608202317973,11.209497772265,10.227671718306));
#59805=CARTESIAN_POINT('Ctrl Pts',(-9.9621133876334,12.0029494910215,10.175338342522));
#59806=CARTESIAN_POINT('Ctrl Pts',(-10.0160450943941,12.8253915288056,10.1230049667379));
#59807=CARTESIAN_POINT('Ctrl Pts',(-10.0196250796435,12.8799852092316,10.1195310786559));
#59808=CARTESIAN_POINT('Ctrl Pts',(-10.0212570407989,12.9347066297247,10.116057190574));
#59809=CARTESIAN_POINT('Ctrl Pts',(-10.0209918820407,12.9894441341194,10.112583302492));
#59810=CARTESIAN_POINT('Ctrl Pts',(-8.29379928253292,10.0211581030209,12.));
#59811=CARTESIAN_POINT('Ctrl Pts',(-8.38688154479599,10.0552080103525,12.));
#59812=CARTESIAN_POINT('Ctrl Pts',(-8.4779006806254,10.0940206699959,12.));
#59813=CARTESIAN_POINT('Ctrl Pts',(-8.56664686325615,10.1372696205127,12.));
#59814=CARTESIAN_POINT('Ctrl Pts',(-8.65733903335545,10.1814669150961,12.));
#59815=CARTESIAN_POINT('Ctrl Pts',(-8.74565814612796,10.2302978026812,12.));
#59816=CARTESIAN_POINT('Ctrl Pts',(-8.83135135493958,10.2834593640583,12.));
#59817=CARTESIAN_POINT('Ctrl Pts',(-8.91318992856164,10.3342296224599,12.));
#59818=CARTESIAN_POINT('Ctrl Pts',(-8.99263375816446,10.3889506025256,12.));
#59819=CARTESIAN_POINT('Ctrl Pts',(-9.06943047246088,10.4473877517771,12.));
#59820=CARTESIAN_POINT('Ctrl Pts',(-9.13662759747024,10.4985202573722,12.));
#59821=CARTESIAN_POINT('Ctrl Pts',(-9.20179774209257,10.5524986289602,12.));
#59822=CARTESIAN_POINT('Ctrl Pts',(-9.26474793392036,10.6091781306825,12.));
#59823=CARTESIAN_POINT('Ctrl Pts',(-9.27985634938565,10.6227815437226,12.));
#59824=CARTESIAN_POINT('Ctrl Pts',(-9.29484046111391,10.636544177759,12.));
#59825=CARTESIAN_POINT('Ctrl Pts',(-9.30967515586603,10.6504428556362,12.));
#59826=CARTESIAN_POINT('Ctrl Pts',(-9.38210515214773,10.718302774818,12.));
#59827=CARTESIAN_POINT('Ctrl Pts',(-9.45106930229927,10.7894833711807,12.));
#59828=CARTESIAN_POINT('Ctrl Pts',(-9.51632661790574,10.8636962448604,12.));
#59829=CARTESIAN_POINT('Ctrl Pts',(-9.58121902341258,10.9374941301685,12.));
#59830=CARTESIAN_POINT('Ctrl Pts',(-9.64244642197802,11.0142912680357,12.));
#59831=CARTESIAN_POINT('Ctrl Pts',(-9.69972824598415,11.0938308479656,12.));
#59832=CARTESIAN_POINT('Ctrl Pts',(-9.75408303717497,11.169306050327,12.));
#59833=CARTESIAN_POINT('Ctrl Pts',(-9.80488522775839,11.2472513152745,12.));
#59834=CARTESIAN_POINT('Ctrl Pts',(-9.85185250012922,11.3274602381139,12.));
#59835=CARTESIAN_POINT('Ctrl Pts',(-9.88922975528545,11.3912916940074,12.));
#59836=CARTESIAN_POINT('Ctrl Pts',(-9.92417754353756,11.4565571180282,12.));
#59837=CARTESIAN_POINT('Ctrl Pts',(-9.95653223361561,11.5231545729247,12.));
#59838=CARTESIAN_POINT('Ctrl Pts',(-9.96243512991986,11.5353048321122,12.));
#59839=CARTESIAN_POINT('Ctrl Pts',(-9.96824994557655,11.5474959894548,12.));
#59840=CARTESIAN_POINT('Ctrl Pts',(-9.97397248881904,11.5597200854486,12.));
#59841=CARTESIAN_POINT('Ctrl Pts',(-10.0145489524258,11.6463966845059,12.));
#59842=CARTESIAN_POINT('Ctrl Pts',(-10.0505436256048,11.7348369448931,12.));
#59843=CARTESIAN_POINT('Ctrl Pts',(-10.0816929753162,11.8247972357439,12.));
#59844=CARTESIAN_POINT('Ctrl Pts',(-10.1128423250276,11.9147575265948,12.));
#59845=CARTESIAN_POINT('Ctrl Pts',(-10.1391468173479,12.0062385811789,12.));
#59846=CARTESIAN_POINT('Ctrl Pts',(-10.1602867132728,12.0990065815937,12.));
#59847=CARTESIAN_POINT('Ctrl Pts',(-10.1814517508012,12.1918849106638,12.));
#59848=CARTESIAN_POINT('Ctrl Pts',(-10.197439126489,12.286054432468,12.));
#59849=CARTESIAN_POINT('Ctrl Pts',(-10.2083242813819,12.381106938598,12.));
#59850=CARTESIAN_POINT('Ctrl Pts',(-10.2138913557349,12.4297203367777,12.));
#59851=CARTESIAN_POINT('Ctrl Pts',(-10.2181230259612,12.4785645227018,12.));
#59852=CARTESIAN_POINT('Ctrl Pts',(-10.2210244442513,12.527583085919,12.));
#59853=CARTESIAN_POINT('Ctrl Pts',(-10.2218610165225,12.5417167152898,12.));
#59854=CARTESIAN_POINT('Ctrl Pts',(-10.2225869774383,12.5558648310221,12.));
#59855=CARTESIAN_POINT('Ctrl Pts',(-10.2232024018895,12.5700260533185,12.));
#59856=CARTESIAN_POINT('Ctrl Pts',(-10.2238236012139,12.5843201583174,12.));
#59857=CARTESIAN_POINT('Ctrl Pts',(-10.2243317772527,12.598618709654,12.));
#59858=CARTESIAN_POINT('Ctrl Pts',(-10.2247273702154,12.6129172463203,12.));
#59859=CARTESIAN_POINT('Ctrl Pts',(-10.227308430526,12.7062085557579,12.));
#59860=CARTESIAN_POINT('Ctrl Pts',(-10.2251031453087,12.7995425030326,12.));
#59861=CARTESIAN_POINT('Ctrl Pts',(-10.2182400386914,12.8925419864032,12.));
#59862=CARTESIAN_POINT('Ctrl Pts',(-10.2113727169558,12.985598587323,12.));
#59863=CARTESIAN_POINT('Ctrl Pts',(-10.1998414736524,13.0783212906945,12.));
#59864=CARTESIAN_POINT('Ctrl Pts',(-10.1837245157332,13.1703195860503,12.));
#59865=CARTESIAN_POINT('Ctrl Pts',(-10.167850633777,13.2609303630954,12.));
#59866=CARTESIAN_POINT('Ctrl Pts',(-10.1475278620093,13.3508392541549,12.));
#59867=CARTESIAN_POINT('Ctrl Pts',(-10.1227882581427,13.4396474637383,12.));
#59868=CARTESIAN_POINT('Ctrl Pts',(-10.1129089853156,13.4751112705354,12.));
#59869=CARTESIAN_POINT('Ctrl Pts',(-10.102324939091,13.5103991993701,12.));
#59870=CARTESIAN_POINT('Ctrl Pts',(-10.0910364592447,13.5454842372103,12.));
#59871=CARTESIAN_POINT('Ctrl Pts',(-10.0850885997417,13.5639704176856,12.));
#59872=CARTESIAN_POINT('Ctrl Pts',(-10.0789451599571,13.5824002543575,12.));
#59873=CARTESIAN_POINT('Ctrl Pts',(-10.0726060885077,13.6007696733809,12.));
#59874=CARTESIAN_POINT('Ctrl Pts',(-10.0672512100823,13.6162870888888,12.));
#59875=CARTESIAN_POINT('Ctrl Pts',(-10.0617593012071,13.6317538427315,12.));
#59876=CARTESIAN_POINT('Ctrl Pts',(-10.05613256518,13.6471627242414,12.));
#59877=CARTESIAN_POINT('Ctrl Pts',(-10.0253173594462,13.7315505205696,12.));
#59878=CARTESIAN_POINT('Ctrl Pts',(-9.99044489732798,13.8142532308756,12.));
#59879=CARTESIAN_POINT('Ctrl Pts',(-9.95156720789968,13.8949006686344,12.));
#59880=CARTESIAN_POINT('Ctrl Pts',(-9.92246136322671,13.9552775025255,12.));
#59881=CARTESIAN_POINT('Ctrl Pts',(-9.89110978386257,14.0145019588769,12.));
#59882=CARTESIAN_POINT('Ctrl Pts',(-9.85752072526523,14.0724054243587,12.));
#59883=CARTESIAN_POINT('Ctrl Pts',(-9.84460176992236,14.0946761373823,12.));
#59884=CARTESIAN_POINT('Ctrl Pts',(-9.83135170762611,14.1167512973966,12.));
#59885=CARTESIAN_POINT('Ctrl Pts',(-9.81777059343282,14.1386207605303,12.));
#59886=CARTESIAN_POINT('Ctrl Pts',(-9.80600921691784,14.1575599275555,12.));
#59887=CARTESIAN_POINT('Ctrl Pts',(-9.79399757751539,14.1763475835755,12.));
#59888=CARTESIAN_POINT('Ctrl Pts',(-9.78174994291027,14.194955852553,12.));
#59889=CARTESIAN_POINT('Ctrl Pts',(-9.73447804437696,14.2667777374594,12.));
#59890=CARTESIAN_POINT('Ctrl Pts',(-9.68365470418875,14.3359945738428,12.));
#59891=CARTESIAN_POINT('Ctrl Pts',(-9.62930889486242,14.4022524491644,12.));
#59892=CARTESIAN_POINT('Ctrl Pts',(-9.58717510546268,14.453621550103,12.));
#59893=CARTESIAN_POINT('Ctrl Pts',(-9.54292331405751,14.5032115233845,12.));
#59894=CARTESIAN_POINT('Ctrl Pts',(-9.49655459700825,14.5508396884611,12.));
#59895=CARTESIAN_POINT('Ctrl Pts',(-9.47068873424204,14.5774081091567,12.));
#59896=CARTESIAN_POINT('Ctrl Pts',(-9.44416391721335,14.6033657382126,12.));
#59897=CARTESIAN_POINT('Ctrl Pts',(-9.41700728965907,14.6287007311509,12.));
#59898=CARTESIAN_POINT('Origin',(-7.5,12.9903810567666,7.5));
#59899=CARTESIAN_POINT('Origin',(15.,1.36827403442078E-16,4.));
#59900=CARTESIAN_POINT('Ctrl Pts',(13.086534003335,1.63598720337497,4.));
#59901=CARTESIAN_POINT('Ctrl Pts',(13.0243671614557,1.57756563722365,4.));
#59902=CARTESIAN_POINT('Ctrl Pts',(12.9655713261624,1.51589246301216,4.));
#59903=CARTESIAN_POINT('Ctrl Pts',(12.9101605215997,1.45134356594541,4.));
#59904=CARTESIAN_POINT('Ctrl Pts',(12.8533994594265,1.38522173305508,4.));
#59905=CARTESIAN_POINT('Ctrl Pts',(12.8001899401135,1.31608182626898,4.));
#59906=CARTESIAN_POINT('Ctrl Pts',(12.7505758639603,1.24428161564212,4.));
#59907=CARTESIAN_POINT('Ctrl Pts',(12.737567030614,1.22545556774005,4.));
#59908=CARTESIAN_POINT('Ctrl Pts',(12.7248055528518,1.20644640781821,4.));
#59909=CARTESIAN_POINT('Ctrl Pts',(12.7122926030956,1.18726014528907,4.));
#59910=CARTESIAN_POINT('Ctrl Pts',(12.7022174307361,1.17181175736453,4.));
#59911=CARTESIAN_POINT('Ctrl Pts',(12.6923030248513,1.15624777849328,4.));
#59912=CARTESIAN_POINT('Ctrl Pts',(12.6825586157748,1.14058556199816,4.));
#59913=CARTESIAN_POINT('Ctrl Pts',(12.6350797654636,1.06427267050556,4.));
#59914=CARTESIAN_POINT('Ctrl Pts',(12.5915831545383,0.985554475328281,4.00000000000001));
#59915=CARTESIAN_POINT('Ctrl Pts',(12.5521056896097,0.904822546167765,4.00000000000001));
#59916=CARTESIAN_POINT('Ctrl Pts',(12.5205631790518,0.840317701884819,4.));
#59917=CARTESIAN_POINT('Ctrl Pts',(12.4915870127793,0.774526199173173,4.));
#59918=CARTESIAN_POINT('Ctrl Pts',(12.4652125787776,0.707630559635218,4.));
#59919=CARTESIAN_POINT('Ctrl Pts',(12.4565302425272,0.685608838292681,4.));
#59920=CARTESIAN_POINT('Ctrl Pts',(12.4481299823828,0.663467358107674,4.));
#59921=CARTESIAN_POINT('Ctrl Pts',(12.4400134491405,0.641212348322469,4.));
#59922=CARTESIAN_POINT('Ctrl Pts',(12.4326491678695,0.6210199648435,4.));
#59923=CARTESIAN_POINT('Ctrl Pts',(12.4255170259942,0.600729502784082,4.));
#59924=CARTESIAN_POINT('Ctrl Pts',(12.41862769741,0.580374130450127,4.));
#59925=CARTESIAN_POINT('Ctrl Pts',(12.3890480800735,0.492977497088245,4.));
#59926=CARTESIAN_POINT('Ctrl Pts',(12.363907391977,0.404299179172776,4.00000000000001));
#59927=CARTESIAN_POINT('Ctrl Pts',(12.3432403919349,0.314735964380019,4.00000000000001));
#59928=CARTESIAN_POINT('Ctrl Pts',(12.322257026321,0.223801736977766,4.00000000000001));
#59929=CARTESIAN_POINT('Ctrl Pts',(12.3058848583804,0.131954509394712,4.));
#59930=CARTESIAN_POINT('Ctrl Pts',(12.2942020415478,0.039576420273935,4.));
#59931=CARTESIAN_POINT('Ctrl Pts',(12.2826102453471,-0.0520819526881022,
4.));
#59932=CARTESIAN_POINT('Ctrl Pts',(12.2756346673422,-0.14426387445687,4.));
#59933=CARTESIAN_POINT('Ctrl Pts',(12.2733985971608,-0.236615283315844,
4.));
#59934=CARTESIAN_POINT('Ctrl Pts',(12.2723186623648,-0.28121741642928,4.));
#59935=CARTESIAN_POINT('Ctrl Pts',(12.2723449592516,-0.325859284098739,
4.));
#59936=CARTESIAN_POINT('Ctrl Pts',(12.2734957210626,-0.370501641907857,
4.));
#59937=CARTESIAN_POINT('Ctrl Pts',(12.2738658684163,-0.384861043177254,
4.));
#59938=CARTESIAN_POINT('Ctrl Pts',(12.2743523774935,-0.399220495972395,
4.));
#59939=CARTESIAN_POINT('Ctrl Pts',(12.2749559214615,-0.413578694513598,
4.));
#59940=CARTESIAN_POINT('Ctrl Pts',(12.2755868612803,-0.428588635239398,
4.));
#59941=CARTESIAN_POINT('Ctrl Pts',(12.2763453773817,-0.443588732674977,
4.));
#59942=CARTESIAN_POINT('Ctrl Pts',(12.2772314223084,-0.458571999977678,
4.));
#59943=CARTESIAN_POINT('Ctrl Pts',(12.2828802428556,-0.554095133908471,
4.));
#59944=CARTESIAN_POINT('Ctrl Pts',(12.2937114584574,-0.649002595692518,
4.));
#59945=CARTESIAN_POINT('Ctrl Pts',(12.3097976800713,-0.742900147453328,
4.));
#59946=CARTESIAN_POINT('Ctrl Pts',(12.3112861449746,-0.75158852771142,4.));
#59947=CARTESIAN_POINT('Ctrl Pts',(12.3128196370525,-0.760268274419424,
4.));
#59948=CARTESIAN_POINT('Ctrl Pts',(12.3143982352413,-0.768939082485976,
4.));
#59949=CARTESIAN_POINT('Ctrl Pts',(12.3307867311623,-0.858956607935255,
4.));
#59950=CARTESIAN_POINT('Ctrl Pts',(12.3520323002905,-0.948010485772638,
4.));
#59951=CARTESIAN_POINT('Ctrl Pts',(12.3778326203319,-1.03586583972401,4.));
#59952=CARTESIAN_POINT('Ctrl Pts',(12.4042241967268,-1.12573454219727,4.));
#59953=CARTESIAN_POINT('Ctrl Pts',(12.435381875245,-1.21434985801567,4.));
#59954=CARTESIAN_POINT('Ctrl Pts',(12.4710363747919,-1.30145748669412,4.));
#59955=CARTESIAN_POINT('Ctrl Pts',(12.4909273060557,-1.35005308827618,4.));
#59956=CARTESIAN_POINT('Ctrl Pts',(12.5122187298043,-1.39817934130794,4.));
#59957=CARTESIAN_POINT('Ctrl Pts',(12.534870586159,-1.44579043537726,4.));
#59958=CARTESIAN_POINT('Ctrl Pts',(12.5412077066689,-1.45911019319316,4.));
#59959=CARTESIAN_POINT('Ctrl Pts',(12.5476516035311,-1.47239000998161,4.));
#59960=CARTESIAN_POINT('Ctrl Pts',(12.5541943737652,-1.48561501829369,4.));
#59961=CARTESIAN_POINT('Ctrl Pts',(12.5969523561364,-1.57204242626194,4.));
#59962=CARTESIAN_POINT('Ctrl Pts',(12.6439961654632,-1.65627338500264,4.));
#59963=CARTESIAN_POINT('Ctrl Pts',(12.6949857265575,-1.73805452373085,4.));
#59964=CARTESIAN_POINT('Ctrl Pts',(12.7469808269627,-1.82144842687817,4.));
#59965=CARTESIAN_POINT('Ctrl Pts',(12.8030791489228,-1.90229571208266,4.));
#59966=CARTESIAN_POINT('Ctrl Pts',(12.8629750013787,-1.98032077373009,4.));
#59967=CARTESIAN_POINT('Ctrl Pts',(12.9233424571313,-2.05896018302908,4.));
#59968=CARTESIAN_POINT('Ctrl Pts',(12.9875679362272,-2.13473359370643,4.));
#59969=CARTESIAN_POINT('Ctrl Pts',(13.0553877098439,-2.20733955177719,4.));
#59970=CARTESIAN_POINT('Ctrl Pts',(13.0913230991629,-2.24581097730712,4.));
#59971=CARTESIAN_POINT('Ctrl Pts',(13.1282683996108,-2.28339271539353,4.));
#59972=CARTESIAN_POINT('Ctrl Pts',(13.1661892287502,-2.32003649064048,4.));
#59973=CARTESIAN_POINT('Ctrl Pts',(13.1814900570711,-2.33482203533466,4.));
#59974=CARTESIAN_POINT('Ctrl Pts',(13.196949744001,-2.34945484110134,4.));
#59975=CARTESIAN_POINT('Ctrl Pts',(13.2125661689314,-2.36393160001069,4.));
#59976=CARTESIAN_POINT('Ctrl Pts',(13.2232570858249,-2.37384230794012,4.));
#59977=CARTESIAN_POINT('Ctrl Pts',(13.2340146157559,-2.3836735202466,4.));
#59978=CARTESIAN_POINT('Ctrl Pts',(13.2448364129784,-2.39342320679516,4.));
#59979=CARTESIAN_POINT('Ctrl Pts',(13.320625051765,-2.46170349859172,4.));
#59980=CARTESIAN_POINT('Ctrl Pts',(13.3995829817648,-2.52600647852482,4.));
#59981=CARTESIAN_POINT('Ctrl Pts',(13.4813873531473,-2.58604589859231,4.));
#59982=CARTESIAN_POINT('Ctrl Pts',(13.5632614554873,-2.64613649693043,4.));
#59983=CARTESIAN_POINT('Ctrl Pts',(13.6479874247046,-2.70195710712452,4.));
#59984=CARTESIAN_POINT('Ctrl Pts',(13.7352864859208,-2.75319451696124,4.));
#59985=CARTESIAN_POINT('Ctrl Pts',(13.8208945029142,-2.80343942212848,4.));
#59986=CARTESIAN_POINT('Ctrl Pts',(13.9089775477651,-2.84927765377448,4.));
#59987=CARTESIAN_POINT('Ctrl Pts',(13.9993066119595,-2.89037749094858,4.));
#59988=CARTESIAN_POINT('Ctrl Pts',(14.025515470362,-2.90230255429857,4.));
#59989=CARTESIAN_POINT('Ctrl Pts',(14.0519135997525,-2.91382843622988,4.));
#59990=CARTESIAN_POINT('Ctrl Pts',(14.0784958352494,-2.92494631785187,4.));
#59991=CARTESIAN_POINT('Ctrl Pts',(14.1199798960696,-2.94229681034347,4.));
#59992=CARTESIAN_POINT('Ctrl Pts',(14.1619123028466,-2.95865373590191,4.));
#59993=CARTESIAN_POINT('Ctrl Pts',(14.204261268307,-2.97402368063354,4.));
#59994=CARTESIAN_POINT('Ctrl Pts',(15.7937992825329,-2.9692229537457,4.));
#59995=CARTESIAN_POINT('Ctrl Pts',(15.8886556608518,-2.93452406683594,4.));
#59996=CARTESIAN_POINT('Ctrl Pts',(15.9814715788842,-2.89484190048077,4.));
#59997=CARTESIAN_POINT('Ctrl Pts',(16.0720047548823,-2.85049467748599,4.));
#59998=CARTESIAN_POINT('Ctrl Pts',(16.1637866430073,-2.80553577910774,4.));
#59999=CARTESIAN_POINT('Ctrl Pts',(16.2532230529932,-2.75578154813471,4.));
#60000=CARTESIAN_POINT('Ctrl Pts',(16.3400275203182,-2.70152291880737,4.));
#60001=CARTESIAN_POINT('Ctrl Pts',(16.3646888442304,-2.686107932988,4.));
#60002=CARTESIAN_POINT('Ctrl Pts',(16.389137491053,-2.67032916740001,4.));
#60003=CARTESIAN_POINT('Ctrl Pts',(16.4133662837328,-2.65419282892726,4.));
#60004=CARTESIAN_POINT('Ctrl Pts',(16.4325631402962,-2.64140775212984,4.));
#60005=CARTESIAN_POINT('Ctrl Pts',(16.4516239542716,-2.62839666993241,4.));
#60006=CARTESIAN_POINT('Ctrl Pts',(16.4705261961219,-2.61517619923621,4.));
#60007=CARTESIAN_POINT('Ctrl Pts',(16.5532306656362,-2.55733163115156,4.));
#60008=CARTESIAN_POINT('Ctrl Pts',(16.6329816584356,-2.49543011909309,4.));
#60009=CARTESIAN_POINT('Ctrl Pts',(16.7095117106738,-2.42976651841151,4.));
#60010=CARTESIAN_POINT('Ctrl Pts',(16.7679773228431,-2.37960239988795,4.));
#60011=CARTESIAN_POINT('Ctrl Pts',(16.8245624524955,-2.32724171199687,4.));
#60012=CARTESIAN_POINT('Ctrl Pts',(16.8791308185435,-2.27280449707864,4.));
#60013=CARTESIAN_POINT('Ctrl Pts',(16.9076285190194,-2.2443752887693,4.));
#60014=CARTESIAN_POINT('Ctrl Pts',(16.9355759205114,-2.21537960309138,4.));
#60015=CARTESIAN_POINT('Ctrl Pts',(16.9629517841853,-2.18583377975445,4.));
#60016=CARTESIAN_POINT('Ctrl Pts',(16.9740993314633,-2.17380261732463,4.));
#60017=CARTESIAN_POINT('Ctrl Pts',(16.9851523150081,-2.16167987026619,4.));
#60018=CARTESIAN_POINT('Ctrl Pts',(16.9960991984116,-2.14947815004889,4.));
#60019=CARTESIAN_POINT('Ctrl Pts',(17.061864093391,-2.07617465177648,4.));
#60020=CARTESIAN_POINT('Ctrl Pts',(17.1238952962526,-1.9999250033291,4.));
#60021=CARTESIAN_POINT('Ctrl Pts',(17.1819478816723,-1.92100525783345,4.));
#60022=CARTESIAN_POINT('Ctrl Pts',(17.2389325987962,-1.84353722880334,4.));
#60023=CARTESIAN_POINT('Ctrl Pts',(17.2920840747574,-1.76349564200828,4.));
#60024=CARTESIAN_POINT('Ctrl Pts',(17.3411263889919,-1.681119910375,4.));
#60025=CARTESIAN_POINT('Ctrl Pts',(17.3892346863819,-1.6003130345782,4.));
#60026=CARTESIAN_POINT('Ctrl Pts',(17.4333891346359,-1.51725940586905,4.));
#60027=CARTESIAN_POINT('Ctrl Pts',(17.473281665729,-1.43217460910322,4.));
#60028=CARTESIAN_POINT('Ctrl Pts',(17.4935758753293,-1.38889009814213,4.));
#60029=CARTESIAN_POINT('Ctrl Pts',(17.5127663147042,-1.34507981852401,4.));
#60030=CARTESIAN_POINT('Ctrl Pts',(17.5308071984732,-1.30077191375233,4.));
#60031=CARTESIAN_POINT('Ctrl Pts',(17.5396600651807,-1.27902952130341,4.));
#60032=CARTESIAN_POINT('Ctrl Pts',(17.548236065603,-1.25716730274661,4.));
#60033=CARTESIAN_POINT('Ctrl Pts',(17.5565294575664,-1.23518860043795,4.));
#60034=CARTESIAN_POINT('Ctrl Pts',(17.5612619499656,-1.22264680305532,4.));
#60035=CARTESIAN_POINT('Ctrl Pts',(17.5659011120686,-1.21007041067208,4.));
#60036=CARTESIAN_POINT('Ctrl Pts',(17.5704433141742,-1.19746790314509,4.));
#60037=CARTESIAN_POINT('Ctrl Pts',(17.601949668132,-1.11005236027246,4.));
#60038=CARTESIAN_POINT('Ctrl Pts',(17.6288373085193,-1.02126995392761,4.));
#60039=CARTESIAN_POINT('Ctrl Pts',(17.6508530784154,-0.931342019285625,
4.));
#60040=CARTESIAN_POINT('Ctrl Pts',(17.6541059208438,-0.918055116184408,
4.));
#60041=CARTESIAN_POINT('Ctrl Pts',(17.6572523179739,-0.90474318860678,4.));
#60042=CARTESIAN_POINT('Ctrl Pts',(17.6602913566075,-0.891406935242469,
4.));
#60043=CARTESIAN_POINT('Ctrl Pts',(17.6812030503878,-0.79963987330047,4.));
#60044=CARTESIAN_POINT('Ctrl Pts',(17.6970357825963,-0.706720788882977,
4.));
#60045=CARTESIAN_POINT('Ctrl Pts',(17.7078979433461,-0.613041608366267,
4.));
#60046=CARTESIAN_POINT('Ctrl Pts',(17.71918010274,-0.515740208504458,4.));
#60047=CARTESIAN_POINT('Ctrl Pts',(17.7250998267343,-0.417617597139405,
4.));
#60048=CARTESIAN_POINT('Ctrl Pts',(17.7257219253175,-0.319126306900475,
4.));
#60049=CARTESIAN_POINT('Ctrl Pts',(17.7259028938113,-0.290475188042702,
4.));
#60050=CARTESIAN_POINT('Ctrl Pts',(17.7256352115795,-0.261793020088843,
4.));
#60051=CARTESIAN_POINT('Ctrl Pts',(17.7249196338,-0.233091376404626,4.));
#60052=CARTESIAN_POINT('Ctrl Pts',(17.7245239501318,-0.217220604586536,
4.));
#60053=CARTESIAN_POINT('Ctrl Pts',(17.7239913108662,-0.201343881980789,
4.));
#60054=CARTESIAN_POINT('Ctrl Pts',(17.7233217966467,-0.185463198608965,
4.));
#60055=CARTESIAN_POINT('Ctrl Pts',(17.7227411089474,-0.171689454568016,
4.));
#60056=CARTESIAN_POINT('Ctrl Pts',(17.7220574547657,-0.157914135821034,
4.));
#60057=CARTESIAN_POINT('Ctrl Pts',(17.7212718008001,-0.144150654953,4.));
#60058=CARTESIAN_POINT('Ctrl Pts',(17.7159690064325,-0.0512536391956395,
4.));
#60059=CARTESIAN_POINT('Ctrl Pts',(17.7060179260155,0.0412556969053557,
4.));
#60060=CARTESIAN_POINT('Ctrl Pts',(17.691537290537,0.133004324856137,4.));
#60061=CARTESIAN_POINT('Ctrl Pts',(17.6770974224585,0.224494652470098,4.));
#60062=CARTESIAN_POINT('Ctrl Pts',(17.6581530629752,0.315229493843254,4.));
#60063=CARTESIAN_POINT('Ctrl Pts',(17.6347733990709,0.404821867293602,4.));
#60064=CARTESIAN_POINT('Ctrl Pts',(17.6117974920603,0.492867018399034,4.));
#60065=CARTESIAN_POINT('Ctrl Pts',(17.5845376887683,0.579809603493695,4.));
#60066=CARTESIAN_POINT('Ctrl Pts',(17.5530192634714,0.665253146715262,4.));
#60067=CARTESIAN_POINT('Ctrl Pts',(17.5376266260196,0.706981166786664,4.));
#60068=CARTESIAN_POINT('Ctrl Pts',(17.521217712657,0.748351139728866,4.));
#60069=CARTESIAN_POINT('Ctrl Pts',(17.5037923624592,0.789313445373718,4.));
#60070=CARTESIAN_POINT('Ctrl Pts',(17.4980299458858,0.802859334911291,4.));
#60071=CARTESIAN_POINT('Ctrl Pts',(17.4921563593103,0.816360622497498,4.));
#60072=CARTESIAN_POINT('Ctrl Pts',(17.4861715515314,0.829815450098292,4.));
#60073=CARTESIAN_POINT('Ctrl Pts',(17.4804842577731,0.842601417477522,4.));
#60074=CARTESIAN_POINT('Ctrl Pts',(17.4746999465266,0.855337690933622,4.));
#60075=CARTESIAN_POINT('Ctrl Pts',(17.4688205030047,0.868019526422757,4.));
#60076=CARTESIAN_POINT('Ctrl Pts',(17.4313685751689,0.948802543693164,4.));
#60077=CARTESIAN_POINT('Ctrl Pts',(17.3900398049897,1.02742425086957,4.));
#60078=CARTESIAN_POINT('Ctrl Pts',(17.3448999527151,1.10353609749938,4.));
#60079=CARTESIAN_POINT('Ctrl Pts',(17.3005164856713,1.17837257715787,4.));
#60080=CARTESIAN_POINT('Ctrl Pts',(17.2524481398624,1.25078327494736,4.));
#60081=CARTESIAN_POINT('Ctrl Pts',(17.2007210868077,1.32040265351989,4.));
#60082=CARTESIAN_POINT('Ctrl Pts',(17.1505256542607,1.38796062589101,4.));
#60083=CARTESIAN_POINT('Ctrl Pts',(17.0968845380256,1.45289058144554,4.));
#60084=CARTESIAN_POINT('Ctrl Pts',(17.0397936511852,1.5148180351349,4.));
#60085=CARTESIAN_POINT('Ctrl Pts',(17.0255930287153,1.53022169128796,4.));
#60086=CARTESIAN_POINT('Ctrl Pts',(17.0111788466503,1.54543936332989,4.));
#60087=CARTESIAN_POINT('Ctrl Pts',(16.9965508084827,1.56046483491105,4.));
#60088=CARTESIAN_POINT('Ctrl Pts',(16.9706944922369,1.58702364891564,4.));
#60089=CARTESIAN_POINT('Ctrl Pts',(16.9441700096348,1.61298203696882,4.));
#60090=CARTESIAN_POINT('Ctrl Pts',(16.9170033607454,1.6383265094434,4.));
#60091=CARTESIAN_POINT('Origin',(15.,0.,14.2084234471775));
#60092=CARTESIAN_POINT('Ctrl Pts',(11.9228311771842,0.0015213020298664,
11.7084234471775));
#60093=CARTESIAN_POINT('Ctrl Pts',(11.9221922557771,0.100409703179003,11.7032843782051));
#60094=CARTESIAN_POINT('Ctrl Pts',(11.9710108327432,1.20571704782255,11.6458119334487));
#60095=CARTESIAN_POINT('Ctrl Pts',(13.3048024582519,3.19795728077006,11.5360061129082));
#60096=CARTESIAN_POINT('Ctrl Pts',(16.7319486542021,3.17774782202826,11.3790059855559));
#60097=CARTESIAN_POINT('Ctrl Pts',(18.606042966971,0.308570934784431,11.2220058582037));
#60098=CARTESIAN_POINT('Ctrl Pts',(17.246562375271,-2.83758641060089,11.0650057308514));
#60099=CARTESIAN_POINT('Ctrl Pts',(13.8725685599584,-3.4391081414099,10.9080056034992));
#60100=CARTESIAN_POINT('Ctrl Pts',(12.0835901505745,-1.55983373126709,10.7891448422745));
#60101=CARTESIAN_POINT('Ctrl Pts',(11.9252787513183,-0.276890505982443,
10.7226174568339));
#60102=CARTESIAN_POINT('Ctrl Pts',(11.9275890856804,-0.00260766251225678,
10.7084234471775));
#60103=CARTESIAN_POINT('Ctrl Pts',(11.9297760945785,-0.00333806817183434,
11.7915765528225));
#60104=CARTESIAN_POINT('Ctrl Pts',(11.9344491671038,0.677708095250012,11.7563842836469));
#60105=CARTESIAN_POINT('Ctrl Pts',(12.4898049314569,2.38075616290146,11.6688586386871));
#60106=CARTESIAN_POINT('Ctrl Pts',(15.2863460006058,3.60696666543133,11.5289996179432));
#60107=CARTESIAN_POINT('Ctrl Pts',(18.1665668486981,1.75247841941832,11.371999490591));
#60108=CARTESIAN_POINT('Ctrl Pts',(18.2084706556688,-1.6752137223659,11.2149993632387));
#60109=CARTESIAN_POINT('Ctrl Pts',(15.3727057323674,-3.59983386165072,11.0579992358865));
#60110=CARTESIAN_POINT('Ctrl Pts',(12.5232213208654,-2.42851998200457,10.9168582990811));
#60111=CARTESIAN_POINT('Ctrl Pts',(11.9339453360424,-0.702880789277512,
10.8280507380598));
#60112=CARTESIAN_POINT('Ctrl Pts',(11.9284560106028,0.0024556673498264,
10.7915765528226));
#60113=CARTESIAN_POINT('Ctrl Pts',(16.9134659966651,1.63598720337493,12.));
#60114=CARTESIAN_POINT('Ctrl Pts',(17.4514117960785,1.00680074451815,11.9476666242159));
#60115=CARTESIAN_POINT('Ctrl Pts',(17.8499101160228,-0.812800245940048,
11.8429998726477));
#60116=CARTESIAN_POINT('Ctrl Pts',(15.8909226224913,-2.8292934693942,11.6859997452955));
#60117=CARTESIAN_POINT('Ctrl Pts',(13.1331777991764,-2.30192506894816,11.5289996179432));
#60118=CARTESIAN_POINT('Ctrl Pts',(12.0494015740803,0.286239346000545,11.371999490591));
#60119=CARTESIAN_POINT('Ctrl Pts',(13.6114658170324,2.61944280277814,11.2149993632387));
#60120=CARTESIAN_POINT('Ctrl Pts',(16.4186369731426,2.60288926043798,11.0579992358865));
#60121=CARTESIAN_POINT('Ctrl Pts',(17.9537052771594,0.252750066152531,10.9009991085342));
#60122=CARTESIAN_POINT('Ctrl Pts',(16.8401564274426,-2.32426347443882,10.743998981182));
#60123=CARTESIAN_POINT('Ctrl Pts',(14.0765223197317,-2.81696917065216,10.5869988538297));
#60124=CARTESIAN_POINT('Ctrl Pts',(12.1409791666289,-0.783732381279285,
10.4299987264775));
#60125=CARTESIAN_POINT('Ctrl Pts',(12.7691475978345,1.95231594579313,10.2729985991252));
#60126=CARTESIAN_POINT('Ctrl Pts',(15.3977426901935,2.93768783020276,10.1159984717729));
#60127=CARTESIAN_POINT('Ctrl Pts',(17.6696781425075,1.28881506595247,9.95899834442072));
#60128=CARTESIAN_POINT('Ctrl Pts',(17.5476875690895,-1.51575474549275,9.80199821706844));
#60129=CARTESIAN_POINT('Ctrl Pts',(15.1411611231766,-2.96113057342894,9.6449980897162));
#60130=CARTESIAN_POINT('Ctrl Pts',(12.6080541376564,-1.75123331751949,9.48799796236395));
#60131=CARTESIAN_POINT('Ctrl Pts',(12.2198279573789,1.02901222386683,9.33099783501168));
#60132=CARTESIAN_POINT('Ctrl Pts',(14.3246087178457,2.88653234022692,9.17399770765945));
#60133=CARTESIAN_POINT('Ctrl Pts',(17.0350193212714,2.15567136478361,9.01699758030717));
#60134=CARTESIAN_POINT('Ctrl Pts',(17.920608575789,-0.508200880905659,8.85999745295495));
#60135=CARTESIAN_POINT('Ctrl Pts',(16.1872601015714,-2.71636448178362,8.70299732560267));
#60136=CARTESIAN_POINT('Ctrl Pts',(13.3892841040964,-2.48873801247178,8.54599719825043));
#60137=CARTESIAN_POINT('Ctrl Pts',(12.0356525030592,-0.0294362811014349,
8.38899707089817));
#60138=CARTESIAN_POINT('Ctrl Pts',(13.3401797411332,2.45626124056312,8.23199694354592));
#60139=CARTESIAN_POINT('Ctrl Pts',(16.1330837289975,2.73940574632503,8.07499681619367));
#60140=CARTESIAN_POINT('Ctrl Pts',(17.9099406666424,0.566098837129481,7.91799668884141));
#60141=CARTESIAN_POINT('Ctrl Pts',(17.0774258920138,-2.11483432920145,7.76099656148916));
#60142=CARTESIAN_POINT('Ctrl Pts',(14.3820633896886,-2.89937526470001,7.6039964341369));
#60143=CARTESIAN_POINT('Ctrl Pts',(12.240810574834,-1.08401858364571,7.44699630678465));
#60144=CARTESIAN_POINT('Ctrl Pts',(12.5737493864543,1.70338795860876,7.28999617943239));
#60145=CARTESIAN_POINT('Ctrl Pts',(15.0823304026287,2.96335018127148,7.13299605208015));
#60146=CARTESIAN_POINT('Ctrl Pts',(17.5170849510905,1.56604785867891,6.97599592472789));
#60147=CARTESIAN_POINT('Ctrl Pts',(17.6947452874587,-1.23554458602037,6.81899579737564));
#60148=CARTESIAN_POINT('Ctrl Pts',(15.4560016501892,-2.92921237979097,6.66199567002338));
#60149=CARTESIAN_POINT('Ctrl Pts',(12.8083570016989,-1.99622726741817,6.50499554267113));
#60150=CARTESIAN_POINT('Ctrl Pts',(12.1259795712872,0.726793862646375,6.34799541531888));
#60151=CARTESIAN_POINT('Ctrl Pts',(14.0207639954511,2.79809220508692,6.19099528796662));
#60152=CARTESIAN_POINT('Ctrl Pts',(16.793638419534,2.3603139527537,6.03399516061437));
#60153=CARTESIAN_POINT('Ctrl Pts',(17.9581406885776,-0.193979547267846,
5.87699503326211));
#60154=CARTESIAN_POINT('Ctrl Pts',(16.4700486085461,-2.57433151465002,5.71999490590987));
#60155=CARTESIAN_POINT('Ctrl Pts',(13.6637522053085,-2.64625223032612,5.56299477855761));
#60156=CARTESIAN_POINT('Ctrl Pts',(12.0556774054966,-0.345259977325435,
5.40599465120536));
#60157=CARTESIAN_POINT('Ctrl Pts',(13.0878139143641,2.26534344968177,5.2489945238531));
#60158=CARTESIAN_POINT('Ctrl Pts',(15.8346085061802,2.84456586771516,5.09199439650085));
#60159=CARTESIAN_POINT('Ctrl Pts',(17.8330357993722,0.87308907652308,4.9349942691486));
#60160=CARTESIAN_POINT('Ctrl Pts',(17.2909861426673,-1.8813930887419,4.77799414179634));
#60161=CARTESIAN_POINT('Ctrl Pts',(14.6947169782024,-2.94862097263666,4.62099401444409));
#60162=CARTESIAN_POINT('Ctrl Pts',(12.3719451483433,-1.37216452037615,4.46399388709184));
#60163=CARTESIAN_POINT('Ctrl Pts',(12.4062682448688,1.4354510150691,4.30699375973958));
#60164=CARTESIAN_POINT('Ctrl Pts',(14.7654540928384,2.95446651190592,4.14999363238733));
#60165=CARTESIAN_POINT('Ctrl Pts',(17.3368403233694,1.82697070537499,3.99299350503508));
#60166=CARTESIAN_POINT('Ctrl Pts',(17.8090202723047,-0.94447711406392,3.83599337768282));
#60167=CARTESIAN_POINT('Ctrl Pts',(16.4499195044998,-2.21828784507026,3.73132662611465));
#60168=CARTESIAN_POINT('Ctrl Pts',(15.6501999979751,-2.43208680203507,3.67899325033057));
#60169=CARTESIAN_POINT('Ctrl Pts',(17.0543315503421,1.75642532122682,12.1070022498898));
#60170=CARTESIAN_POINT('Ctrl Pts',(17.6318798475343,1.08091940905997,12.0546688741057));
#60171=CARTESIAN_POINT('Ctrl Pts',(18.0597148196982,-0.872636980364766,
11.9500021225376));
#60172=CARTESIAN_POINT('Ctrl Pts',(15.9565105706019,-3.03758041662798,11.7930019951853));
#60173=CARTESIAN_POINT('Ctrl Pts',(12.9957460688013,-2.47138820543743,11.6360018678331));
#60174=CARTESIAN_POINT('Ctrl Pts',(11.8321843976736,0.307311716258913,11.4790017404808));
#60175=CARTESIAN_POINT('Ctrl Pts',(13.5092446974389,2.81228096210878,11.3220016131285));
#60176=CARTESIAN_POINT('Ctrl Pts',(16.5230742001624,2.79450878096808,11.1650014857763));
#60177=CARTESIAN_POINT('Ctrl Pts',(18.1711511737633,0.271357022363162,11.008001358424));
#60178=CARTESIAN_POINT('Ctrl Pts',(16.9756250767187,-2.49537111982618,10.8510012310718));
#60179=CARTESIAN_POINT('Ctrl Pts',(14.0085377331406,-3.02434882757141,10.6940011037195));
#60180=CARTESIAN_POINT('Ctrl Pts',(11.9305037500974,-0.841429197431721,
10.5370009763673));
#60181=CARTESIAN_POINT('Ctrl Pts',(12.604916689446,2.09604155530799,10.380000849015));
#60182=CARTESIAN_POINT('Ctrl Pts',(15.4270237144567,3.15395455427992,10.2230007216628));
#60183=CARTESIAN_POINT('Ctrl Pts',(17.8662145274442,1.38369506286337,10.0660005943105));
#60184=CARTESIAN_POINT('Ctrl Pts',(17.7352432511039,-1.62734158938471,9.90900046695827));
#60185=CARTESIAN_POINT('Ctrl Pts',(15.1515531237706,-3.17912310554764,9.752000339606));
#60186=CARTESIAN_POINT('Ctrl Pts',(12.4319638497434,-1.88015562464175,9.59500021225376));
#60187=CARTESIAN_POINT('Ctrl Pts',(12.0151572316991,1.10476605325709,9.4380000849015));
#60188=CARTESIAN_POINT('Ctrl Pts',(14.2748877575176,3.09903309907051,9.28099995754925));
#60189=CARTESIAN_POINT('Ctrl Pts',(17.1848333884845,2.31436759501462,9.123999830197));
#60190=CARTESIAN_POINT('Ctrl Pts',(18.1356179591903,-0.54561361705707,8.96699970284474));
#60191=CARTESIAN_POINT('Ctrl Pts',(16.274663824375,-2.9163378219851,8.80999957549249));
#60192=CARTESIAN_POINT('Ctrl Pts',(13.2707064095419,-2.67195394559781,8.65299944814023));
#60193=CARTESIAN_POINT('Ctrl Pts',(11.817423147442,-0.0316033214579261,
8.49599932078798));
#60194=CARTESIAN_POINT('Ctrl Pts',(13.2179870812285,2.63708629845826,8.33899919343572));
#60195=CARTESIAN_POINT('Ctrl Pts',(16.2164990952103,2.94107533850731,8.18199906608348));
#60196=CARTESIAN_POINT('Ctrl Pts',(18.1241646998305,0.607773905443812,8.02499893873121));
#60197=CARTESIAN_POINT('Ctrl Pts',(17.2303618464606,-2.27052421824958,7.86799881137898));
#60198=CARTESIAN_POINT('Ctrl Pts',(14.3365721278107,-3.11282149405098,7.71099868402671));
#60199=CARTESIAN_POINT('Ctrl Pts',(12.0376845476387,-1.16382187163074,7.55399855667447));
#60200=CARTESIAN_POINT('Ctrl Pts',(12.3951336511175,1.8287879857503,7.39699842932221));
#60201=CARTESIAN_POINT('Ctrl Pts',(15.088391402809,3.1815061164965,7.23999830196995));
#60202=CARTESIAN_POINT('Ctrl Pts',(17.7023877293502,1.68133718134365,7.0829981746177));
#60203=CARTESIAN_POINT('Ctrl Pts',(17.893127065655,-1.3265029163517,6.92599804726544));
#60204=CARTESIAN_POINT('Ctrl Pts',(15.4895715829936,-3.14485515809799,6.7689979199132));
#60205=CARTESIAN_POINT('Ctrl Pts',(12.6470126114897,-2.1431855409282,6.61199779256094));
#60206=CARTESIAN_POINT('Ctrl Pts',(11.9143999144365,0.780298978519449,6.45499766520869));
#60207=CARTESIAN_POINT('Ctrl Pts',(13.9486745921371,3.00408217741771,6.29799753785644));
#60208=CARTESIAN_POINT('Ctrl Pts',(16.9256825057651,2.53407556251617,6.14099741050418));
#60209=CARTESIAN_POINT('Ctrl Pts',(18.1759131113316,-0.208259934991238,
5.98399728315193));
#60210=CARTESIAN_POINT('Ctrl Pts',(16.5782706577155,-2.76384867084273,5.82699715579967));
#60211=CARTESIAN_POINT('Ctrl Pts',(13.5653803054279,-2.84106404628923,5.66999702844742));
#60212=CARTESIAN_POINT('Ctrl Pts',(11.8389222432929,-0.370677328850485,
5.51299690109516));
#60213=CARTESIAN_POINT('Ctrl Pts',(12.9470425851866,2.43211352025748,5.35599677374291));
#60214=CARTESIAN_POINT('Ctrl Pts',(15.8960507212661,3.05397713847976,5.19899664639066));
#60215=CARTESIAN_POINT('Ctrl Pts',(18.0415982494816,0.937364154516702,5.04199651903841));
#60216=CARTESIAN_POINT('Ctrl Pts',(17.459643977202,-2.01989749884988,4.88499639168616));
#60217=CARTESIAN_POINT('Ctrl Pts',(14.6722426504805,-3.16569257287314,4.7279962643339));
#60218=CARTESIAN_POINT('Ctrl Pts',(12.1784729871356,-1.4731805380298,4.57099613698165));
#60219=CARTESIAN_POINT('Ctrl Pts',(12.215322881631,1.54112605834992,4.41399600962939));
#60220=CARTESIAN_POINT('Ctrl Pts',(14.7481872905369,3.17196844909489,4.25699588227714));
#60221=CARTESIAN_POINT('Ctrl Pts',(17.5088738513129,1.96146864806794,4.09999575492489));
#60222=CARTESIAN_POINT('Ctrl Pts',(18.0158147471675,-1.0140076371251,3.94299562757263));
#60223=CARTESIAN_POINT('Ctrl Pts',(16.5566596891409,-2.38159377580301,3.83832887600446));
#60224=CARTESIAN_POINT('Ctrl Pts',(15.698066426161,-2.61113218593862,3.78599550022038));
#60225=CARTESIAN_POINT('Ctrl Pts',(17.1951971040191,1.87686343907872,12.2140044997796));
#60226=CARTESIAN_POINT('Ctrl Pts',(17.8123478989901,1.15503807360179,12.1616711239955));
#60227=CARTESIAN_POINT('Ctrl Pts',(18.2695195233736,-0.932473714789483,
12.0570043724274));
#60228=CARTESIAN_POINT('Ctrl Pts',(16.0220985187125,-3.24586736386177,11.9000042450751));
#60229=CARTESIAN_POINT('Ctrl Pts',(12.8583143384262,-2.6408513419267,11.7430041177229));
#60230=CARTESIAN_POINT('Ctrl Pts',(11.6149672212669,0.328384086517278,11.5860039903706));
#60231=CARTESIAN_POINT('Ctrl Pts',(13.4070235778454,3.00511912143942,11.4290038630183));
#60232=CARTESIAN_POINT('Ctrl Pts',(16.6275114271823,2.98612830149817,11.2720037356661));
#60233=CARTESIAN_POINT('Ctrl Pts',(18.3885970703671,0.289963978573797,11.1150036083139));
#60234=CARTESIAN_POINT('Ctrl Pts',(17.1110937259949,-2.66647876521353,10.9580034809616));
#60235=CARTESIAN_POINT('Ctrl Pts',(13.9405531465495,-3.23172848449065,10.8010033536093));
#60236=CARTESIAN_POINT('Ctrl Pts',(11.7200283335659,-0.899126013584159,
10.6440032262571));
#60237=CARTESIAN_POINT('Ctrl Pts',(12.4406857810575,2.23976716482285,10.4870030989048));
#60238=CARTESIAN_POINT('Ctrl Pts',(15.4563047387199,3.37022127835708,10.3300029715526));
#60239=CARTESIAN_POINT('Ctrl Pts',(18.0627509123809,1.47857505977427,10.1730028442003));
#60240=CARTESIAN_POINT('Ctrl Pts',(17.9227989331183,-1.73892843327666,10.0160027168481));
#60241=CARTESIAN_POINT('Ctrl Pts',(15.1619451243646,-3.39711563766634,9.85900258949583));
#60242=CARTESIAN_POINT('Ctrl Pts',(12.2558735618304,-2.00907793176401,9.70200246214356));
#60243=CARTESIAN_POINT('Ctrl Pts',(11.8104865060192,1.18051988264736,9.54500233479131));
#60244=CARTESIAN_POINT('Ctrl Pts',(14.2251667971895,3.31153385791409,9.38800220743906));
#60245=CARTESIAN_POINT('Ctrl Pts',(17.3346474556976,2.47306382524563,9.2310020800868));
#60246=CARTESIAN_POINT('Ctrl Pts',(18.3506273425917,-0.583026353208485,
9.07400195273456));
#60247=CARTESIAN_POINT('Ctrl Pts',(16.3620675471785,-3.11631116218659,8.91700182538229));
#60248=CARTESIAN_POINT('Ctrl Pts',(13.1521287149875,-2.85516987872383,8.76000169803006));
#60249=CARTESIAN_POINT('Ctrl Pts',(11.5991937918248,-0.0337703618144171,
8.60300157067778));
#60250=CARTESIAN_POINT('Ctrl Pts',(13.0957944213239,2.81791135635341,8.44600144332555));
#60251=CARTESIAN_POINT('Ctrl Pts',(16.2999144614232,3.1427449306896,8.28900131597327));
#60252=CARTESIAN_POINT('Ctrl Pts',(18.3383887330186,0.649448973758145,8.13200118862104));
#60253=CARTESIAN_POINT('Ctrl Pts',(17.3832978009075,-2.42621410729771,7.97500106126878));
#60254=CARTESIAN_POINT('Ctrl Pts',(14.2910808659327,-3.32626772340195,7.81800093391653));
#60255=CARTESIAN_POINT('Ctrl Pts',(11.8345585204434,-1.24362515961579,7.66100080656427));
#60256=CARTESIAN_POINT('Ctrl Pts',(12.2165179157807,1.95418801289184,7.50400067921202));
#60257=CARTESIAN_POINT('Ctrl Pts',(15.0944524029892,3.39966205172151,7.34700055185976));
#60258=CARTESIAN_POINT('Ctrl Pts',(17.8876905076099,1.7966265040084,7.19000042450751));
#60259=CARTESIAN_POINT('Ctrl Pts',(18.0915088438512,-1.41746124668302,7.03300029715526));
#60260=CARTESIAN_POINT('Ctrl Pts',(15.523141515798,-3.36049793640501,6.87600016980301));
#60261=CARTESIAN_POINT('Ctrl Pts',(12.4856682212804,-2.29014381443823,6.71900004245075));
#60262=CARTESIAN_POINT('Ctrl Pts',(11.7028202575859,0.833804094392522,6.5619999150985));
#60263=CARTESIAN_POINT('Ctrl Pts',(13.8765851888231,3.21007214974851,6.40499978774624));
#60264=CARTESIAN_POINT('Ctrl Pts',(17.0577265919963,2.70783717227864,6.247999660394));
#60265=CARTESIAN_POINT('Ctrl Pts',(18.3936855340856,-0.22254032271463,6.09099953304174));
#60266=CARTESIAN_POINT('Ctrl Pts',(16.6864927068848,-2.95336582703543,5.93399940568949));
#60267=CARTESIAN_POINT('Ctrl Pts',(13.4670084055473,-3.03587586225233,5.77699927833723));
#60268=CARTESIAN_POINT('Ctrl Pts',(11.6221670810891,-0.396094680375534,
5.61999915098498));
#60269=CARTESIAN_POINT('Ctrl Pts',(12.806271256009,2.59888359083319,5.46299902363272));
#60270=CARTESIAN_POINT('Ctrl Pts',(15.957492936352,3.26338840924436,5.30599889628048));
#60271=CARTESIAN_POINT('Ctrl Pts',(18.250160699591,1.00163923251032,5.14899876892821));
#60272=CARTESIAN_POINT('Ctrl Pts',(17.6283018117366,-2.15840190895786,4.99199864157597));
#60273=CARTESIAN_POINT('Ctrl Pts',(14.6497683227587,-3.38276417310961,4.8349985142237));
#60274=CARTESIAN_POINT('Ctrl Pts',(11.9850008259279,-1.57419655568344,4.67799838687146));
#60275=CARTESIAN_POINT('Ctrl Pts',(12.0243775183933,1.64680110163074,4.5209982595192));
#60276=CARTESIAN_POINT('Ctrl Pts',(14.7309204882355,3.38947038628386,4.36399813216696));
#60277=CARTESIAN_POINT('Ctrl Pts',(17.6809073792564,2.09596659076089,4.20699800481469));
#60278=CARTESIAN_POINT('Ctrl Pts',(18.2226092220303,-1.08353816018628,4.04999787746244));
#60279=CARTESIAN_POINT('Ctrl Pts',(16.663399873782,-2.54489970653575,3.94533112589427));
#60280=CARTESIAN_POINT('Ctrl Pts',(15.7459328543469,-2.79017756984216,3.89299775011019));
#60281=CARTESIAN_POINT('Ctrl Pts',(17.3360626576962,1.99730155693062,12.3210067496694));
#60282=CARTESIAN_POINT('Ctrl Pts',(17.9928159504458,1.22915673814361,12.2686733738853));
#60283=CARTESIAN_POINT('Ctrl Pts',(18.4793242270491,-0.9923104492142,12.1640066223172));
#60284=CARTESIAN_POINT('Ctrl Pts',(16.087686466823,-3.45415431109555,12.0070064949649));
#60285=CARTESIAN_POINT('Ctrl Pts',(12.7208826080511,-2.81031447841596,11.8500063676127));
#60286=CARTESIAN_POINT('Ctrl Pts',(11.3977500448602,0.349456456775644,11.6930062402604));
#60287=CARTESIAN_POINT('Ctrl Pts',(13.3048024582519,3.19795728077006,11.5360061129082));
#60288=CARTESIAN_POINT('Ctrl Pts',(16.7319486542021,3.17774782202826,11.3790059855559));
#60289=CARTESIAN_POINT('Ctrl Pts',(18.606042966971,0.308570934784431,11.2220058582037));
#60290=CARTESIAN_POINT('Ctrl Pts',(17.246562375271,-2.83758641060089,11.0650057308514));
#60291=CARTESIAN_POINT('Ctrl Pts',(13.8725685599584,-3.4391081414099,10.9080056034992));
#60292=CARTESIAN_POINT('Ctrl Pts',(11.5095529170344,-0.956822829736598,
10.7510054761469));
#60293=CARTESIAN_POINT('Ctrl Pts',(12.276454872669,2.38349277433771,10.5940053487947));
#60294=CARTESIAN_POINT('Ctrl Pts',(15.4855857629831,3.58648800243424,10.4370052214424));
#60295=CARTESIAN_POINT('Ctrl Pts',(18.2592872973176,1.57345505668517,10.2800050940901));
#60296=CARTESIAN_POINT('Ctrl Pts',(18.1103546151327,-1.85051527716861,10.1230049667379));
#60297=CARTESIAN_POINT('Ctrl Pts',(15.1723371249586,-3.61510816978504,9.96600483938563));
#60298=CARTESIAN_POINT('Ctrl Pts',(12.0797832739173,-2.13800023888626,9.80900471203338));
#60299=CARTESIAN_POINT('Ctrl Pts',(11.6058157803393,1.25627371203762,9.65200458468112));
#60300=CARTESIAN_POINT('Ctrl Pts',(14.1754458368614,3.52403461675767,9.49500445732887));
#60301=CARTESIAN_POINT('Ctrl Pts',(17.4844615229107,2.63176005547664,9.33800432997661));
#60302=CARTESIAN_POINT('Ctrl Pts',(18.565636725993,-0.620439089359897,9.18100420262437));
#60303=CARTESIAN_POINT('Ctrl Pts',(16.4494712699821,-3.31628450238807,9.0240040752721));
#60304=CARTESIAN_POINT('Ctrl Pts',(13.033551020433,-3.03838581184986,8.86700394791986));
#60305=CARTESIAN_POINT('Ctrl Pts',(11.3809644362075,-0.0359374021709085,
8.7100038205676));
#60306=CARTESIAN_POINT('Ctrl Pts',(12.9736017614192,2.99873641424856,8.55300369321535));
#60307=CARTESIAN_POINT('Ctrl Pts',(16.383329827636,3.34441452287188,8.39600356586309));
#60308=CARTESIAN_POINT('Ctrl Pts',(18.5526127662067,0.691124042072478,8.23900343851084));
#60309=CARTESIAN_POINT('Ctrl Pts',(17.5362337553543,-2.58190399634584,8.08200331115859));
#60310=CARTESIAN_POINT('Ctrl Pts',(14.2455896040548,-3.53971395275292,7.92500318380633));
#60311=CARTESIAN_POINT('Ctrl Pts',(11.6314324932481,-1.32342844760082,7.76800305645409));
#60312=CARTESIAN_POINT('Ctrl Pts',(12.0379021804438,2.07958804003338,7.61100292910183));
#60313=CARTESIAN_POINT('Ctrl Pts',(15.1005134031695,3.61781798694653,7.45400280174957));
#60314=CARTESIAN_POINT('Ctrl Pts',(18.0729932858696,1.91191582667314,7.29700267439733));
#60315=CARTESIAN_POINT('Ctrl Pts',(18.2898906220475,-1.50841957701434,7.14000254704506));
#60316=CARTESIAN_POINT('Ctrl Pts',(15.5567114486024,-3.57614071471203,6.98300241969282));
#60317=CARTESIAN_POINT('Ctrl Pts',(12.3243238310711,-2.43710208794826,6.82600229234056));
#60318=CARTESIAN_POINT('Ctrl Pts',(11.4912406007353,0.887309210265594,6.66900216498831));
#60319=CARTESIAN_POINT('Ctrl Pts',(13.8044957855091,3.41606212207931,6.51200203763605));
#60320=CARTESIAN_POINT('Ctrl Pts',(17.1897706782275,2.88159878204111,6.35500191028381));
#60321=CARTESIAN_POINT('Ctrl Pts',(18.6114579568395,-0.236820710438023,
6.19800178293155));
#60322=CARTESIAN_POINT('Ctrl Pts',(16.7947147560542,-3.14288298322814,6.04100165557929));
#60323=CARTESIAN_POINT('Ctrl Pts',(13.3686365056666,-3.23068767821543,5.88400152822705));
#60324=CARTESIAN_POINT('Ctrl Pts',(11.4054119188853,-0.421512031900586,
5.72700140087479));
#60325=CARTESIAN_POINT('Ctrl Pts',(12.6654999268314,2.7656536614089,5.57000127352253));
#60326=CARTESIAN_POINT('Ctrl Pts',(16.0189351514379,3.47279968000896,5.41300114617029));
#60327=CARTESIAN_POINT('Ctrl Pts',(18.4587231497003,1.06591431050395,5.25600101881802));
#60328=CARTESIAN_POINT('Ctrl Pts',(17.7969596462713,-2.29690631906584,5.09900089146578));
#60329=CARTESIAN_POINT('Ctrl Pts',(14.6272939950368,-3.59983577334609,4.94200076411352));
#60330=CARTESIAN_POINT('Ctrl Pts',(11.7915286647202,-1.67521257333708,4.78500063676127));
#60331=CARTESIAN_POINT('Ctrl Pts',(11.8334321551556,1.75247614491157,4.62800050940901));
#60332=CARTESIAN_POINT('Ctrl Pts',(14.713653685934,3.60697232347283,4.47100038205677));
#60333=CARTESIAN_POINT('Ctrl Pts',(17.8529409071999,2.23046453345384,4.3140002547045));
#60334=CARTESIAN_POINT('Ctrl Pts',(18.4294036968932,-1.15306868324745,4.15700012735226));
#60335=CARTESIAN_POINT('Ctrl Pts',(16.7701400584231,-2.7082056372685,4.05233337578409));
#60336=CARTESIAN_POINT('Ctrl Pts',(15.7937992825329,-2.9692229537457,4.));
#60337=CARTESIAN_POINT('Ctrl Pts',(16.9134659966651,1.63598720337493,12.));
#60338=CARTESIAN_POINT('Ctrl Pts',(16.9751046175812,1.57806203522303,12.));
#60339=CARTESIAN_POINT('Ctrl Pts',(17.0333781400082,1.51698823254714,12.));
#60340=CARTESIAN_POINT('Ctrl Pts',(17.0882869575319,1.45315007481724,12.));
#60341=CARTESIAN_POINT('Ctrl Pts',(17.144646063235,1.38762578124011,12.));
#60342=CARTESIAN_POINT('Ctrl Pts',(17.1974608152615,1.31918874417436,12.));
#60343=CARTESIAN_POINT('Ctrl Pts',(17.246706209466,1.24820595309377,12.));
#60344=CARTESIAN_POINT('Ctrl Pts',(17.2968789923958,1.17588641486748,12.));
#60345=CARTESIAN_POINT('Ctrl Pts',(17.3433471915708,1.10092373974675,12.));
#60346=CARTESIAN_POINT('Ctrl Pts',(17.3860513180704,1.02366428011772,12.));
#60347=CARTESIAN_POINT('Ctrl Pts',(17.4053930048836,0.988671683523578,12.));
#60348=CARTESIAN_POINT('Ctrl Pts',(17.4239620441889,0.953207420756028,12.));
#60349=CARTESIAN_POINT('Ctrl Pts',(17.4417503295423,0.917301461090561,12.));
#60350=CARTESIAN_POINT('Ctrl Pts',(17.4518550628932,0.896904883178727,12.));
#60351=CARTESIAN_POINT('Ctrl Pts',(17.4617078263978,0.876365752925188,12.));
#60352=CARTESIAN_POINT('Ctrl Pts',(17.4713068826732,0.855689404786285,12.));
#60353=CARTESIAN_POINT('Ctrl Pts',(17.4795241183999,0.837989495363037,12.));
#60354=CARTESIAN_POINT('Ctrl Pts',(17.4875575606575,0.820183889043797,12.));
#60355=CARTESIAN_POINT('Ctrl Pts',(17.4953933345483,0.802305631697034,12.));
#60356=CARTESIAN_POINT('Ctrl Pts',(17.5320009593848,0.718780947752926,12.));
#60357=CARTESIAN_POINT('Ctrl Pts',(17.5643466650844,0.633572893252199,12.));
#60358=CARTESIAN_POINT('Ctrl Pts',(17.5924032599934,0.547079296293481,12.));
#60359=CARTESIAN_POINT('Ctrl Pts',(17.6209190605514,0.45917004827483,12.));
#60360=CARTESIAN_POINT('Ctrl Pts',(17.6450046970528,0.369932078122487,12.));
#60361=CARTESIAN_POINT('Ctrl Pts',(17.6645925974806,0.27974597155399,12.));
#60362=CARTESIAN_POINT('Ctrl Pts',(17.6832979692358,0.193623180766213,12.));
#60363=CARTESIAN_POINT('Ctrl Pts',(17.6979018128389,0.106634841931331,12.));
#60364=CARTESIAN_POINT('Ctrl Pts',(17.7083066964275,0.0190916104279826,
12.));
#60365=CARTESIAN_POINT('Ctrl Pts',(17.7128967523775,-0.0195275944118574,
12.));
#60366=CARTESIAN_POINT('Ctrl Pts',(17.7166691326112,-0.0582549851430788,
12.));
#60367=CARTESIAN_POINT('Ctrl Pts',(17.7196128778618,-0.0970645844891166,
12.));
#60368=CARTESIAN_POINT('Ctrl Pts',(17.720985220376,-0.115157204130783,12.));
#60369=CARTESIAN_POINT('Ctrl Pts',(17.7221774501012,-0.13326769426837,12.));
#60370=CARTESIAN_POINT('Ctrl Pts',(17.7231883308136,-0.151393437782305,
12.));
#60371=CARTESIAN_POINT('Ctrl Pts',(17.724162595519,-0.168862632662539,12.));
#60372=CARTESIAN_POINT('Ctrl Pts',(17.7249684090533,-0.186348823197974,
12.));
#60373=CARTESIAN_POINT('Ctrl Pts',(17.7256040109254,-0.203825085573831,
12.));
#60374=CARTESIAN_POINT('Ctrl Pts',(17.7290683171088,-0.299078303780242,
12.));
#60375=CARTESIAN_POINT('Ctrl Pts',(17.7274898676139,-0.394183686637061,
12.));
#60376=CARTESIAN_POINT('Ctrl Pts',(17.7208064378308,-0.488742644592356,
12.));
#60377=CARTESIAN_POINT('Ctrl Pts',(17.71415791669,-0.582807705707687,12.));
#60378=CARTESIAN_POINT('Ctrl Pts',(17.7024579548962,-0.676332990245415,
12.));
#60379=CARTESIAN_POINT('Ctrl Pts',(17.6855973100545,-0.768943912339204,
12.));
#60380=CARTESIAN_POINT('Ctrl Pts',(17.6690987547922,-0.859565975160523,
12.));
#60381=CARTESIAN_POINT('Ctrl Pts',(17.6476591367551,-0.949313458601225,
12.));
#60382=CARTESIAN_POINT('Ctrl Pts',(17.6215530748909,-1.03794459575461,12.));
#60383=CARTESIAN_POINT('Ctrl Pts',(17.6062284518588,-1.08997231149527,12.));
#60384=CARTESIAN_POINT('Ctrl Pts',(17.5892948213721,-1.14161533429799,12.));
#60385=CARTESIAN_POINT('Ctrl Pts',(17.5707996132467,-1.19282361176805,12.));
#60386=CARTESIAN_POINT('Ctrl Pts',(17.5660385338913,-1.20600576527691,12.));
#60387=CARTESIAN_POINT('Ctrl Pts',(17.5611731178881,-1.21916127939291,12.));
#60388=CARTESIAN_POINT('Ctrl Pts',(17.5562068240413,-1.23228215182306,12.));
#60389=CARTESIAN_POINT('Ctrl Pts',(17.5231582789659,-1.31959590274395,12.));
#60390=CARTESIAN_POINT('Ctrl Pts',(17.4857269461903,-1.40516846103908,12.));
#60391=CARTESIAN_POINT('Ctrl Pts',(17.4442438276358,-1.48876399852657,12.));
#60392=CARTESIAN_POINT('Ctrl Pts',(17.4011939593262,-1.57551680317371,12.));
#60393=CARTESIAN_POINT('Ctrl Pts',(17.3537803586004,-1.6601411473433,12.));
#60394=CARTESIAN_POINT('Ctrl Pts',(17.302316868041,-1.74237153203792,12.));
#60395=CARTESIAN_POINT('Ctrl Pts',(17.2502282381553,-1.82560078887907,12.));
#60396=CARTESIAN_POINT('Ctrl Pts',(17.1939903374979,-1.90637839472423,12.));
#60397=CARTESIAN_POINT('Ctrl Pts',(17.133876364298,-1.98441530832993,12.));
#60398=CARTESIAN_POINT('Ctrl Pts',(17.0944014617075,-2.03565962639887,12.));
#60399=CARTESIAN_POINT('Ctrl Pts',(17.0532540884055,-2.08572182092047,12.));
#60400=CARTESIAN_POINT('Ctrl Pts',(17.0105008848643,-2.13451422415292,12.));
#60401=CARTESIAN_POINT('Ctrl Pts',(16.9990423392555,-2.14759137233113,12.));
#60402=CARTESIAN_POINT('Ctrl Pts',(16.9874683992165,-2.16057727630897,12.));
#60403=CARTESIAN_POINT('Ctrl Pts',(16.9757802548447,-2.17347017426791,12.));
#60404=CARTESIAN_POINT('Ctrl Pts',(16.9646250327531,-2.18577521906894,12.));
#60405=CARTESIAN_POINT('Ctrl Pts',(16.953371454143,-2.19798925370335,12.));
#60406=CARTESIAN_POINT('Ctrl Pts',(16.942023959817,-2.2101077517839,12.));
#60407=CARTESIAN_POINT('Ctrl Pts',(16.8702005619852,-2.28681117932109,12.));
#60408=CARTESIAN_POINT('Ctrl Pts',(16.7945813632066,-2.35973107336475,12.));
#60409=CARTESIAN_POINT('Ctrl Pts',(16.7155099454751,-2.42853427108366,12.));
#60410=CARTESIAN_POINT('Ctrl Pts',(16.6562063821765,-2.48013666937285,12.));
#60411=CARTESIAN_POINT('Ctrl Pts',(16.5949596324728,-2.52942316838901,12.));
#60412=CARTESIAN_POINT('Ctrl Pts',(16.5318955908763,-2.57624166180053,12.));
#60413=CARTESIAN_POINT('Ctrl Pts',(16.509253132243,-2.59305133294597,12.));
#60414=CARTESIAN_POINT('Ctrl Pts',(16.4863762692883,-2.60954274193113,12.));
#60415=CARTESIAN_POINT('Ctrl Pts',(16.4632703841368,-2.62570843265804,12.));
#60416=CARTESIAN_POINT('Ctrl Pts',(16.4439550552025,-2.63922211680365,12.));
#60417=CARTESIAN_POINT('Ctrl Pts',(16.4244771453842,-2.65250971655999,12.));
#60418=CARTESIAN_POINT('Ctrl Pts',(16.4048604457735,-2.66555338685653,12.));
#60419=CARTESIAN_POINT('Ctrl Pts',(16.3198883986288,-2.72205358257614,12.));
#60420=CARTESIAN_POINT('Ctrl Pts',(16.2322397460524,-2.7740341002851,12.));
#60421=CARTESIAN_POINT('Ctrl Pts',(16.1422018474634,-2.82118285115376,12.));
#60422=CARTESIAN_POINT('Ctrl Pts',(16.0701250286698,-2.85892620174232,12.));
#60423=CARTESIAN_POINT('Ctrl Pts',(15.9965161480314,-2.89357290485328,12.));
#60424=CARTESIAN_POINT('Ctrl Pts',(15.9215058272316,-2.92494553699154,12.));
#60425=CARTESIAN_POINT('Ctrl Pts',(15.8800022019638,-2.94230418782848,12.));
#60426=CARTESIAN_POINT('Ctrl Pts',(15.8380692864041,-2.95866019100725,12.));
#60427=CARTESIAN_POINT('Ctrl Pts',(15.795740524146,-2.97402278592473,12.));
#60428=CARTESIAN_POINT('Ctrl Pts',(12.4833920687165,-0.00213593309729046,
10.387416697508));
#60429=CARTESIAN_POINT('Ctrl Pts',(12.4814996767346,-0.226800666605093,
10.4016107071645));
#60430=CARTESIAN_POINT('Ctrl Pts',(12.5091661046464,-0.451007239373056,
10.415804716821));
#60431=CARTESIAN_POINT('Ctrl Pts',(12.5682644306803,-0.666597124996037,
10.4299987264775));
#60432=CARTESIAN_POINT('Ctrl Pts',(12.7861602176632,-1.46147797773692,10.4823321022615));
#60433=CARTESIAN_POINT('Ctrl Pts',(13.4313412686974,-2.13922357419454,10.5346654780456));
#60434=CARTESIAN_POINT('Ctrl Pts',(14.2145374788331,-2.39597875638779,10.5869988538297));
#60435=CARTESIAN_POINT('Ctrl Pts',(14.9977336889687,-2.65273393858105,10.6393322296138));
#60436=CARTESIAN_POINT('Ctrl Pts',(15.9189450582056,-2.48849870650994,10.6916656053979));
#60437=CARTESIAN_POINT('Ctrl Pts',(16.5651422177769,-1.97687883370916,10.743998981182));
#60438=CARTESIAN_POINT('Ctrl Pts',(17.2113393773482,-1.46525896090837,10.7963323569661));
#60439=CARTESIAN_POINT('Ctrl Pts',(17.5825223272538,-0.60625444737792,10.8486657327501));
#60440=CARTESIAN_POINT('Ctrl Pts',(17.5122690848705,0.214937675101548,10.9009991085342));
#60441=CARTESIAN_POINT('Ctrl Pts',(17.4420158424871,1.03612979758102,10.9533324843183));
#60442=CARTESIAN_POINT('Ctrl Pts',(16.9303264078149,1.8195095290095,11.0056658601024));
#60443=CARTESIAN_POINT('Ctrl Pts',(16.206619831127,2.2139583184471,11.0579992358865));
#60444=CARTESIAN_POINT('Ctrl Pts',(15.4829132544392,2.60840710788471,11.1103326116706));
#60445=CARTESIAN_POINT('Ctrl Pts',(14.5471895357358,2.61392495533142,11.1626659874547));
#60446=CARTESIAN_POINT('Ctrl Pts',(13.8189836358921,2.22781663625852,11.2149993632387));
#60447=CARTESIAN_POINT('Ctrl Pts',(13.0907777360484,1.84170831718561,11.2673327390228));
#60448=CARTESIAN_POINT('Ctrl Pts',(12.5700896550643,1.06397383159308,11.3196661148069));
#60449=CARTESIAN_POINT('Ctrl Pts',(12.4903749854216,0.243745852972027,11.371999490591));
#60450=CARTESIAN_POINT('Ctrl Pts',(12.4825471092477,0.163200539545801,11.3771385595633));
#60451=CARTESIAN_POINT('Ctrl Pts',(12.4789715321031,0.0822454620963692,
11.3822776285357));
#60452=CARTESIAN_POINT('Ctrl Pts',(12.4794948718273,0.00124609658704006,
11.387416697508));
#60453=CARTESIAN_POINT('Ctrl Pts',(14.2062007174671,-2.96922295374568,12.));
#60454=CARTESIAN_POINT('Ctrl Pts',(13.2298599415769,-2.70820563726846,11.9476666242159));
#60455=CARTESIAN_POINT('Ctrl Pts',(11.5705939465555,-1.15308308242658,11.8429998726477));
#60456=CARTESIAN_POINT('Ctrl Pts',(12.1470611574329,2.23047193499529,11.6859997452955));
#60457=CARTESIAN_POINT('Ctrl Pts',(15.2863460006058,3.60696666543133,11.5289996179432));
#60458=CARTESIAN_POINT('Ctrl Pts',(18.1665668486981,1.75247841941832,11.371999490591));
#60459=CARTESIAN_POINT('Ctrl Pts',(18.2084706556688,-1.6752137223659,11.2149993632387));
#60460=CARTESIAN_POINT('Ctrl Pts',(15.3727057323674,-3.59983386165072,11.0579992358865));
#60461=CARTESIAN_POINT('Ctrl Pts',(12.2030412422492,-2.29690621757914,10.9009991085342));
#60462=CARTESIAN_POINT('Ctrl Pts',(11.5412777161188,1.06591431606771,10.743998981182));
#60463=CARTESIAN_POINT('Ctrl Pts',(13.9810651784412,3.47279856287599,10.5869988538297));
#60464=CARTESIAN_POINT('Ctrl Pts',(17.3344994031312,2.76565299665532,10.4299987264775));
#60465=CARTESIAN_POINT('Ctrl Pts',(18.5945871152999,-0.421511967551375,
10.2729985991252));
#60466=CARTESIAN_POINT('Ctrl Pts',(16.6313630370479,-3.23068676566348,10.115998471773));
#60467=CARTESIAN_POINT('Ctrl Pts',(13.205285741413,-3.14288213812672,9.9589983444207));
#60468=CARTESIAN_POINT('Ctrl Pts',(11.388543028433,-0.236820637232293,9.80199821706845));
#60469=CARTESIAN_POINT('Ctrl Pts',(12.8102299232355,2.88159798857394,9.6449980897162));
#60470=CARTESIAN_POINT('Ctrl Pts',(16.1955038860992,3.41606118929613,9.48799796236394));
#60471=CARTESIAN_POINT('Ctrl Pts',(18.5087584392439,0.887308966009096,9.3309978350117));
#60472=CARTESIAN_POINT('Ctrl Pts',(17.6756754360527,-2.43710142000481,9.17399770765943));
#60473=CARTESIAN_POINT('Ctrl Pts',(14.4432887039958,-3.57613973602564,9.0169975803072));
#60474=CARTESIAN_POINT('Ctrl Pts',(11.7101102785552,-1.50841916383422,8.85999745295492));
#60475=CARTESIAN_POINT('Ctrl Pts',(11.9270075555053,1.91191530312036,8.70299732560268));
#60476=CARTESIAN_POINT('Ctrl Pts',(14.8994866243195,3.61781699652394,8.54599719825042));
#60477=CARTESIAN_POINT('Ctrl Pts',(17.9620970086125,2.07958747065415,8.38899707089818));
#60478=CARTESIAN_POINT('Ctrl Pts',(18.3685665845007,-1.32342808525659,8.23199694354591));
#60479=CARTESIAN_POINT('Ctrl Pts',(15.7544101894084,-3.53971298366467,8.07499681619367));
#60480=CARTESIAN_POINT('Ctrl Pts',(12.4637669390099,-2.58190328946754,7.91799668884141));
#60481=CARTESIAN_POINT('Ctrl Pts',(11.4473882064255,0.691123852849571,7.76099656148916));
#60482=CARTESIAN_POINT('Ctrl Pts',(13.6166705510885,3.34441360725337,7.60399643413689));
#60483=CARTESIAN_POINT('Ctrl Pts',(17.0263976837988,2.99873559323853,7.44699630678466));
#60484=CARTESIAN_POINT('Ctrl Pts',(18.6190345729722,-0.0359373922966709,
7.2899961794324));
#60485=CARTESIAN_POINT('Ctrl Pts',(16.9664484412042,-3.03838498006983,7.13299605208014));
#60486=CARTESIAN_POINT('Ctrl Pts',(13.5505291268344,-3.3162835943375,6.97599592472789));
#60487=CARTESIAN_POINT('Ctrl Pts',(11.4343642502377,-0.620438919723572,
6.81899579737564));
#60488=CARTESIAN_POINT('Ctrl Pts',(12.5155391572145,2.63175933537736,6.66199567002338));
#60489=CARTESIAN_POINT('Ctrl Pts',(15.824553937525,3.52403365117268,6.50499554267113));
#60490=CARTESIAN_POINT('Ctrl Pts',(18.3941832901488,1.25627336953411,6.34799541531888));
#60491=CARTESIAN_POINT('Ctrl Pts',(17.9202159270872,-2.13799965619268,6.19099528796662));
#60492=CARTESIAN_POINT('Ctrl Pts',(14.8276629212552,-3.61510717519363,6.03399516061437));
#60493=CARTESIAN_POINT('Ctrl Pts',(11.889646238299,-1.85051477939823,5.87699503326212));
#60494=CARTESIAN_POINT('Ctrl Pts',(11.7407135913467,1.57345464202167,5.71999490590987));
#60495=CARTESIAN_POINT('Ctrl Pts',(14.5144143770745,3.58648699137295,5.56299477855761));
#60496=CARTESIAN_POINT('Ctrl Pts',(17.7235443678513,2.3834921742297,5.40599465120536));
#60497=CARTESIAN_POINT('Ctrl Pts',(18.4904461542425,-0.956822661448993,
5.2489945238531));
#60498=CARTESIAN_POINT('Ctrl Pts',(16.1274310791049,-3.43910703392132,5.09199439650085));
#60499=CARTESIAN_POINT('Ctrl Pts',(12.7534383414036,-2.83758592474999,4.9349942691486));
#60500=CARTESIAN_POINT('Ctrl Pts',(11.3939578227468,0.308571354444121,4.77799414179634));
#60501=CARTESIAN_POINT('Ctrl Pts',(13.2680522040149,3.17774609218688,4.62099401444409));
#60502=CARTESIAN_POINT('Ctrl Pts',(16.6951963308219,3.19795784272698,4.46399388709183));
#60503=CARTESIAN_POINT('Ctrl Pts',(18.6022504225887,0.349454018091392,4.30699375973959));
#60504=CARTESIAN_POINT('Ctrl Pts',(17.2791139286761,-2.8103099931699,4.14999363238733));
#60505=CARTESIAN_POINT('Ctrl Pts',(13.9123194271849,-3.45415924122653,3.99299350503508));
#60506=CARTESIAN_POINT('Ctrl Pts',(11.5206656746196,-0.992299917670973,
3.83599337768282));
#60507=CARTESIAN_POINT('Ctrl Pts',(12.0071840495542,1.22915673814367,3.73132662611465));
#60508=CARTESIAN_POINT('Ctrl Pts',(12.6639373423039,1.99730155693067,3.67899325033057));
#60509=CARTESIAN_POINT('Ctrl Pts',(14.254067145653,-2.79017756984214,12.1070022498898));
#60510=CARTESIAN_POINT('Ctrl Pts',(13.336600126218,-2.54489970653572,12.0546688741057));
#60511=CARTESIAN_POINT('Ctrl Pts',(11.7773885635194,-1.08355169108889,11.9500021225376));
#60512=CARTESIAN_POINT('Ctrl Pts',(12.3190945608781,2.0959735459863,11.7930019951853));
#60513=CARTESIAN_POINT('Ctrl Pts',(15.2690792172061,3.38946506942463,11.636001867833));
#60514=CARTESIAN_POINT('Ctrl Pts',(17.9756215455284,1.64680323898379,11.4790017404808));
#60515=CARTESIAN_POINT('Ctrl Pts',(18.014998535442,-1.57419763542533,11.3220016131285));
#60516=CARTESIAN_POINT('Ctrl Pts',(15.3502314210832,-3.38276237669027,11.1650014857763));
#60517=CARTESIAN_POINT('Ctrl Pts',(12.3716990232057,-2.15840181359085,11.008001358424));
#60518=CARTESIAN_POINT('Ctrl Pts',(11.7498401140189,1.00163923773859,10.8510012310718));
#60519=CARTESIAN_POINT('Ctrl Pts',(14.0425073736352,3.26338735947497,10.6940011037195));
#60520=CARTESIAN_POINT('Ctrl Pts',(17.1937281143572,2.59888296616453,10.5370009763673));
#60521=CARTESIAN_POINT('Ctrl Pts',(18.3778320113351,-0.396094619906611,
10.380000849015));
#60522=CARTESIAN_POINT('Ctrl Pts',(16.5329911647418,-3.03587500472764,10.2230007216628));
#60523=CARTESIAN_POINT('Ctrl Pts',(13.3135077605849,-2.95336503289398,10.0660005943105));
#60524=CARTESIAN_POINT('Ctrl Pts',(11.6063153917746,-0.222540253923235,
9.90900046695825));
#60525=CARTESIAN_POINT('Ctrl Pts',(12.9422739731982,2.70783642665787,9.75200033960602));
#60526=CARTESIAN_POINT('Ctrl Pts',(16.1234145025873,3.21007127321255,9.59500021225374));
#60527=CARTESIAN_POINT('Ctrl Pts',(18.297178840283,0.83380386486479,9.43800008490151));
#60528=CARTESIAN_POINT('Ctrl Pts',(17.5143310900362,-2.29014318677205,9.28099995754924));
#60529=CARTESIAN_POINT('Ctrl Pts',(14.4768586275985,-3.36049701673381,9.12399983019701));
#60530=CARTESIAN_POINT('Ctrl Pts',(11.9084920024447,-1.41746085841783,8.96699970284473));
#60531=CARTESIAN_POINT('Ctrl Pts',(12.1123102830297,1.79662601202607,8.8099995754925));
#60532=CARTESIAN_POINT('Ctrl Pts',(14.9055476228422,3.39966112102182,8.65299944814023));
#60533=CARTESIAN_POINT('Ctrl Pts',(17.7834813221759,1.95418747784641,8.49599932078799));
#60534=CARTESIAN_POINT('Ctrl Pts',(18.1654406129175,-1.24362481912106,8.33899919343572));
#60535=CARTESIAN_POINT('Ctrl Pts',(15.7089189399847,-3.32626681275013,8.18199906608348));
#60536=CARTESIAN_POINT('Ctrl Pts',(12.6167028515863,-2.42621344304447,8.02499893873122));
#60537=CARTESIAN_POINT('Ctrl Pts',(11.6616121809635,0.649448795945457,7.86799881137897));
#60538=CARTESIAN_POINT('Ctrl Pts',(13.7000858944641,3.14274407028327,7.71099868402671));
#60539=CARTESIAN_POINT('Ctrl Pts',(16.9042050573477,2.81791058485063,7.55399855667447));
#60540=CARTESIAN_POINT('Ctrl Pts',(18.4008052771018,-0.033770352535599,
7.3969984293222));
#60541=CARTESIAN_POINT('Ctrl Pts',(16.8478707791132,-2.85516909710049,7.23999830196996));
#60542=CARTESIAN_POINT('Ctrl Pts',(13.6379328257098,-3.11631030889185,7.08299817461769));
#60543=CARTESIAN_POINT('Ctrl Pts',(11.6493735747719,-0.583026193801301,
6.92599804726545));
#60544=CARTESIAN_POINT('Ctrl Pts',(12.6653531834158,2.47306314856864,6.76899791991319));
#60545=CARTESIAN_POINT('Ctrl Pts',(15.7748329908015,3.31153295055427,6.61199779256095));
#60546=CARTESIAN_POINT('Ctrl Pts',(18.1895126205188,1.18051956079695,6.45499766520868));
#60547=CARTESIAN_POINT('Ctrl Pts',(17.7441256873539,-2.00907738420709,6.29799753785643));
#60548=CARTESIAN_POINT('Ctrl Pts',(14.8380549190625,-3.39711470304921,6.14099741050418));
#60549=CARTESIAN_POINT('Ctrl Pts',(12.0772018688511,-1.73892796552204,5.98399728315193));
#60550=CARTESIAN_POINT('Ctrl Pts',(11.9372499226966,1.47857467011516,5.82699715579967));
#60551=CARTESIAN_POINT('Ctrl Pts',(14.5436953928922,3.3702203282632,5.66999702844742));
#60552=CARTESIAN_POINT('Ctrl Pts',(17.5593135052598,2.2397666009016,5.51299690109516));
#60553=CARTESIAN_POINT('Ctrl Pts',(18.2799707937134,-0.89912585544437,5.35599677374292));
#60554=CARTESIAN_POINT('Ctrl Pts',(16.0594465142784,-3.23172744378409,5.19899664639066));
#60555=CARTESIAN_POINT('Ctrl Pts',(12.888906947464,-2.66647830865965,5.04199651903841));
#60556=CARTESIAN_POINT('Ctrl Pts',(11.6114036717303,0.289964372927834,4.88499639168615));
#60557=CARTESIAN_POINT('Ctrl Pts',(13.3724893792839,2.98612667596695,4.72799626433391));
#60558=CARTESIAN_POINT('Ctrl Pts',(16.5929752842478,3.0051196495101,4.57099613698165));
#60559=CARTESIAN_POINT('Ctrl Pts',(18.3850332179946,0.328381794886706,4.41399600962939));
#60560=CARTESIAN_POINT('Ctrl Pts',(17.1416824071377,-2.64084712714285,4.25699588227714));
#60561=CARTESIAN_POINT('Ctrl Pts',(13.9779070198844,-3.24587199670379,4.09999575492489));
#60562=CARTESIAN_POINT('Ctrl Pts',(11.7304709872286,-0.932463818302713,
3.94299562757263));
#60563=CARTESIAN_POINT('Ctrl Pts',(12.1876521010099,1.15503807360185,3.83832887600446));
#60564=CARTESIAN_POINT('Ctrl Pts',(12.8048028959809,1.87686343907877,3.78599550022038));
#60565=CARTESIAN_POINT('Ctrl Pts',(14.3019335738389,-2.6111321859386,12.2140044997796));
#60566=CARTESIAN_POINT('Ctrl Pts',(13.4433403108591,-2.38159377580297,12.1616711239955));
#60567=CARTESIAN_POINT('Ctrl Pts',(11.9841831804832,-1.0140202997512,12.0570043724274));
#60568=CARTESIAN_POINT('Ctrl Pts',(12.4911279643235,1.96147515697731,11.9000042450751));
#60569=CARTESIAN_POINT('Ctrl Pts',(15.2518124338064,3.17196347341793,11.7430041177229));
#60570=CARTESIAN_POINT('Ctrl Pts',(17.7846762423587,1.54112805854926,11.5860039903706));
#60571=CARTESIAN_POINT('Ctrl Pts',(17.8215264152151,-1.47318154848477,11.4290038630184));
#60572=CARTESIAN_POINT('Ctrl Pts',(15.3277571097989,-3.16569089172983,11.2720037356661));
#60573=CARTESIAN_POINT('Ctrl Pts',(12.5403568041622,-2.01989740960257,11.1150036083138));
#60574=CARTESIAN_POINT('Ctrl Pts',(11.958402511919,0.937364159409468,10.9580034809616));
#60575=CARTESIAN_POINT('Ctrl Pts',(14.1039495688293,3.05397615607396,10.8010033536093));
#60576=CARTESIAN_POINT('Ctrl Pts',(17.0529568255832,2.43211293567374,10.6440032262571));
#60577=CARTESIAN_POINT('Ctrl Pts',(18.1610769073704,-0.370677272261844,
10.4870030989048));
#60578=CARTESIAN_POINT('Ctrl Pts',(16.4346192924356,-2.8410632437918,10.3300029715526));
#60579=CARTESIAN_POINT('Ctrl Pts',(13.4217297797568,-2.76384792766124,10.1730028442003));
#60580=CARTESIAN_POINT('Ctrl Pts',(11.8240877551162,-0.208259870614178,
10.0160027168481));
#60581=CARTESIAN_POINT('Ctrl Pts',(13.0743180231609,2.5340748647418,9.85900258949582));
#60582=CARTESIAN_POINT('Ctrl Pts',(16.0513251190755,3.00408135712897,9.70200246214356));
#60583=CARTESIAN_POINT('Ctrl Pts',(18.085599241322,0.780298763720488,9.54500233479132));
#60584=CARTESIAN_POINT('Ctrl Pts',(17.3529867440197,-2.14318495353929,9.38800220743906));
#60585=CARTESIAN_POINT('Ctrl Pts',(14.5104285512012,-3.14485429744199,9.23100208008681));
#60586=CARTESIAN_POINT('Ctrl Pts',(12.1068737263342,-1.32650255300144,9.07400195273456));
#60587=CARTESIAN_POINT('Ctrl Pts',(12.2976130105542,1.68133672093178,8.9170018253823));
#60588=CARTESIAN_POINT('Ctrl Pts',(14.9116086213649,3.1815052455197,8.76000169803005));
#60589=CARTESIAN_POINT('Ctrl Pts',(17.6048656357394,1.82878748503868,8.60300157067779));
#60590=CARTESIAN_POINT('Ctrl Pts',(17.9623146413344,-1.16382155298553,8.44600144332554));
#60591=CARTESIAN_POINT('Ctrl Pts',(15.663427690561,-3.11282064183558,8.28900131597329));
#60592=CARTESIAN_POINT('Ctrl Pts',(12.7696387641627,-2.27052359662139,8.13200118862103));
#60593=CARTESIAN_POINT('Ctrl Pts',(11.8758361555014,0.607773739041346,7.97500106126878));
#60594=CARTESIAN_POINT('Ctrl Pts',(13.7835012378397,2.94107453331316,7.81800093391652));
#60595=CARTESIAN_POINT('Ctrl Pts',(16.7820124308966,2.63708557646273,7.66100080656428));
#60596=CARTESIAN_POINT('Ctrl Pts',(18.1825759812315,-0.031603312774529,
7.50400067921202));
#60597=CARTESIAN_POINT('Ctrl Pts',(16.7292931170223,-2.67195321413115,7.34700055185977));
#60598=CARTESIAN_POINT('Ctrl Pts',(13.7253365245851,-2.9163370234462,7.1900004245075));
#60599=CARTESIAN_POINT('Ctrl Pts',(11.8643828993062,-0.545613467879027,
7.03300029715527));
#60600=CARTESIAN_POINT('Ctrl Pts',(12.8151672096171,2.31436696175991,6.876000169803));
#60601=CARTESIAN_POINT('Ctrl Pts',(15.725112044078,3.09903224993587,6.71900004245076));
#60602=CARTESIAN_POINT('Ctrl Pts',(17.9848419508889,1.10476575205979,6.56199991509849));
#60603=CARTESIAN_POINT('Ctrl Pts',(17.5680354476207,-1.8801551122215,6.40499978774625));
#60604=CARTESIAN_POINT('Ctrl Pts',(14.8484469168698,-3.17912223090478,6.24799966039399));
#60605=CARTESIAN_POINT('Ctrl Pts',(12.2647574994032,-1.62734115164585,6.09099953304174));
#60606=CARTESIAN_POINT('Ctrl Pts',(12.1337862540464,1.38369469820864,5.93399940568949));
#60607=CARTESIAN_POINT('Ctrl Pts',(14.5729764087098,3.15395366515346,5.77699927833723));
#60608=CARTESIAN_POINT('Ctrl Pts',(17.3950826426682,2.0960410275735,5.61999915098498));
#60609=CARTESIAN_POINT('Ctrl Pts',(18.0694954331843,-0.841429049439745,
5.46299902363272));
#60610=CARTESIAN_POINT('Ctrl Pts',(15.991461949452,-3.02434785364687,5.30599889628047));
#60611=CARTESIAN_POINT('Ctrl Pts',(13.0243755535244,-2.49537069256931,5.14899876892822));
#60612=CARTESIAN_POINT('Ctrl Pts',(11.8288495207139,0.271357391411547,4.99199864157596));
#60613=CARTESIAN_POINT('Ctrl Pts',(13.4769265545529,2.79450725974701,4.83499851422372));
#60614=CARTESIAN_POINT('Ctrl Pts',(16.4907542376736,2.81228145629323,4.67799838687145));
#60615=CARTESIAN_POINT('Ctrl Pts',(18.1678160134006,0.307309571682018,4.52099825951921));
#60616=CARTESIAN_POINT('Ctrl Pts',(17.0042508855994,-2.47138426111579,4.36399813216695));
#60617=CARTESIAN_POINT('Ctrl Pts',(14.0434946125838,-3.03758475218105,4.2069980048147));
#60618=CARTESIAN_POINT('Ctrl Pts',(11.9402762998377,-0.872627718934448,
4.04999787746244));
#60619=CARTESIAN_POINT('Ctrl Pts',(12.3681201524657,1.08091940906002,3.94533112589428));
#60620=CARTESIAN_POINT('Ctrl Pts',(12.9456684496579,1.75642532122687,3.89299775011019));
#60621=CARTESIAN_POINT('Ctrl Pts',(14.3498000020249,-2.43208680203506,12.3210067496694));
#60622=CARTESIAN_POINT('Ctrl Pts',(13.5500804955002,-2.21828784507023,12.2686733738853));
#60623=CARTESIAN_POINT('Ctrl Pts',(12.1909777974471,-0.944488908413503,
12.1640066223172));
#60624=CARTESIAN_POINT('Ctrl Pts',(12.6631613677687,1.82697676796832,12.0070064949649));
#60625=CARTESIAN_POINT('Ctrl Pts',(15.2345456504068,2.95446187741122,11.8500063676127));
#60626=CARTESIAN_POINT('Ctrl Pts',(17.593730939189,1.43545287811473,11.6930062402604));
#60627=CARTESIAN_POINT('Ctrl Pts',(17.6280542949882,-1.37216546154421,11.5360061129082));
#60628=CARTESIAN_POINT('Ctrl Pts',(15.3052827985147,-2.94861940676938,11.3790059855559));
#60629=CARTESIAN_POINT('Ctrl Pts',(12.7090145851187,-1.88139300561428,11.2220058582036));
#60630=CARTESIAN_POINT('Ctrl Pts',(12.1669649098191,0.873089081080348,11.0650057308514));
#60631=CARTESIAN_POINT('Ctrl Pts',(14.1653917640233,2.84456495267294,10.9080056034991));
#60632=CARTESIAN_POINT('Ctrl Pts',(16.9121855368091,2.26534290518294,10.7510054761469));
#60633=CARTESIAN_POINT('Ctrl Pts',(17.9443218034057,-0.345259924617078,
10.5940053487946));
#60634=CARTESIAN_POINT('Ctrl Pts',(16.3362474201295,-2.64625148285596,10.4370052214424));
#60635=CARTESIAN_POINT('Ctrl Pts',(13.5299517989286,-2.57433082242851,10.2800050940901));
#60636=CARTESIAN_POINT('Ctrl Pts',(12.0418601184578,-0.193979487305122,
10.1230049667379));
#60637=CARTESIAN_POINT('Ctrl Pts',(13.2063620731236,2.36031330282573,9.96600483938562));
#60638=CARTESIAN_POINT('Ctrl Pts',(15.9792357355636,2.79809144104539,9.80900471203338));
#60639=CARTESIAN_POINT('Ctrl Pts',(17.874019642361,0.726793662576183,9.65200458468112));
#60640=CARTESIAN_POINT('Ctrl Pts',(17.1916423980032,-1.99622672030653,9.49500445732887));
#60641=CARTESIAN_POINT('Ctrl Pts',(14.5439984748038,-2.92921157815017,9.33800432997662));
#60642=CARTESIAN_POINT('Ctrl Pts',(12.3052554502237,-1.23554424758505,9.18100420262436));
#60643=CARTESIAN_POINT('Ctrl Pts',(12.4829157380786,1.56604742983749,9.02400407527211));
#60644=CARTESIAN_POINT('Ctrl Pts',(14.9176696198875,2.96334937001758,8.86700394791986));
#60645=CARTESIAN_POINT('Ctrl Pts',(17.4262499493028,1.70338749223094,8.7100038205676));
#60646=CARTESIAN_POINT('Ctrl Pts',(17.7591886697512,-1.08401828684999,8.55300369321535));
#60647=CARTESIAN_POINT('Ctrl Pts',(15.6179364411373,-2.89937447092104,8.3960035658631));
#60648=CARTESIAN_POINT('Ctrl Pts',(12.922574676739,-2.11483375019832,8.23900343851085));
#60649=CARTESIAN_POINT('Ctrl Pts',(12.0900601300394,0.566098682137233,8.08200331115859));
#60650=CARTESIAN_POINT('Ctrl Pts',(13.8669165812153,2.73940499634305,7.92500318380633));
#60651=CARTESIAN_POINT('Ctrl Pts',(16.6598198044455,2.45626056807483,7.76800305645408));
#60652=CARTESIAN_POINT('Ctrl Pts',(17.9643466853611,-0.029436273013457,
7.61100292910183));
#60653=CARTESIAN_POINT('Ctrl Pts',(16.6107154549314,-2.4887373311618,7.45400280174958));
#60654=CARTESIAN_POINT('Ctrl Pts',(13.8127402234604,-2.71636373800054,7.29700267439732));
#60655=CARTESIAN_POINT('Ctrl Pts',(12.0793922238404,-0.508200741956758,
7.14000254704508));
#60656=CARTESIAN_POINT('Ctrl Pts',(12.9649812358183,2.15567077495119,6.98300241969281));
#60657=CARTESIAN_POINT('Ctrl Pts',(15.6753910973545,2.88653154931746,6.82600229234056));
#60658=CARTESIAN_POINT('Ctrl Pts',(17.780171281259,1.02901194332264,6.66900216498831));
#60659=CARTESIAN_POINT('Ctrl Pts',(17.3919452078874,-1.75123284023591,6.51200203763606));
#60660=CARTESIAN_POINT('Ctrl Pts',(14.8588389146771,-2.96112975876036,6.3550019102838));
#60661=CARTESIAN_POINT('Ctrl Pts',(12.4523131299553,-1.51575433776966,6.19800178293155));
#60662=CARTESIAN_POINT('Ctrl Pts',(12.3303225853962,1.28881472630212,6.04100165557929));
#60663=CARTESIAN_POINT('Ctrl Pts',(14.6022574245275,2.93768700204372,5.88400152822705));
#60664=CARTESIAN_POINT('Ctrl Pts',(17.2308517800767,1.95231545424541,5.72700140087478));
#60665=CARTESIAN_POINT('Ctrl Pts',(17.8590200726551,-0.783732243435121,
5.57000127352254));
#60666=CARTESIAN_POINT('Ctrl Pts',(15.9234773846255,-2.81696826350965,5.41300114617029));
#60667=CARTESIAN_POINT('Ctrl Pts',(13.1598441595847,-2.32426307647897,5.25600101881803));
#60668=CARTESIAN_POINT('Ctrl Pts',(12.0462953696974,0.252750409895257,5.09900089146578));
#60669=CARTESIAN_POINT('Ctrl Pts',(13.5813637298219,2.60288784352708,4.94200076411352));
#60670=CARTESIAN_POINT('Ctrl Pts',(16.3885331910994,2.61944326307635,4.78500063676127));
#60671=CARTESIAN_POINT('Ctrl Pts',(17.9505988088066,0.286237348477332,4.62800050940901));
#60672=CARTESIAN_POINT('Ctrl Pts',(16.8668193640612,-2.30192139508873,4.47100038205677));
#60673=CARTESIAN_POINT('Ctrl Pts',(14.1090822052833,-2.82929750765831,4.3140002547045));
#60674=CARTESIAN_POINT('Ctrl Pts',(12.1500816124467,-0.812791619566185,
4.15700012735226));
#60675=CARTESIAN_POINT('Ctrl Pts',(12.5485882039215,1.0068007445182,4.05233337578409));
#60676=CARTESIAN_POINT('Ctrl Pts',(13.086534003335,1.63598720337497,4.));
#60677=CARTESIAN_POINT('Ctrl Pts',(12.4841021658346,0.00201143405015815,
11.112583302492));
#60678=CARTESIAN_POINT('Ctrl Pts',(12.4821471482924,0.253216278985343,11.0967241119451));
#60679=CARTESIAN_POINT('Ctrl Pts',(12.5168205167969,0.503894392425629,11.0808649213983));
#60680=CARTESIAN_POINT('Ctrl Pts',(12.5903776647364,0.742588045230009,11.0650057308514));
#60681=CARTESIAN_POINT('Ctrl Pts',(12.8331071945538,1.53024770494455,11.0126723550673));
#60682=CARTESIAN_POINT('Ctrl Pts',(13.4992494792886,2.18740632880874,10.9603389792832));
#60683=CARTESIAN_POINT('Ctrl Pts',(14.2901195837869,2.41944863282584,10.9080056034991));
#60684=CARTESIAN_POINT('Ctrl Pts',(15.0809896882853,2.65149093684294,10.8556722277151));
#60685=CARTESIAN_POINT('Ctrl Pts',(15.9965876125472,2.45841692101294,10.803338851931));
#60686=CARTESIAN_POINT('Ctrl Pts',(16.6264092857776,1.92677944146461,10.7510054761469));
#60687=CARTESIAN_POINT('Ctrl Pts',(17.256230959008,1.39514196191627,10.6986721003628));
#60688=CARTESIAN_POINT('Ctrl Pts',(17.6002763812068,0.524941018649596,10.6463387245787));
#60689=CARTESIAN_POINT('Ctrl Pts',(17.5042866950936,-0.293658046023555,
10.5940053487946));
#60690=CARTESIAN_POINT('Ctrl Pts',(17.4082970089803,-1.11225711069671,10.5416719730106));
#60691=CARTESIAN_POINT('Ctrl Pts',(16.8722722145549,-1.87925429677634,10.4893385972265));
#60692=CARTESIAN_POINT('Ctrl Pts',(16.1365438804754,-2.25076611307824,10.4370052214424));
#60693=CARTESIAN_POINT('Ctrl Pts',(15.4008155463959,-2.62227792938014,10.3846718456583));
#60694=CARTESIAN_POINT('Ctrl Pts',(14.4653836726623,-2.59830437590432,10.3323384698742));
#60695=CARTESIAN_POINT('Ctrl Pts',(13.749652455717,-2.18959237664585,10.2800050940901));
#60696=CARTESIAN_POINT('Ctrl Pts',(13.0339212387717,-1.78088037738738,10.2276717183061));
#60697=CARTESIAN_POINT('Ctrl Pts',(12.5378906786147,-0.98742993234625,10.175338342522));
#60698=CARTESIAN_POINT('Ctrl Pts',(12.4839590576472,-0.164989244803877,
10.1230049667379));
#60699=CARTESIAN_POINT('Ctrl Pts',(12.4803790780928,-0.110395654006944,
10.1195310786559));
#60700=CARTESIAN_POINT('Ctrl Pts',(12.4787471194664,-0.0556743234800699,
10.1160571905739));
#60701=CARTESIAN_POINT('Ctrl Pts',(12.4790122776664,-0.000936909191352325,
10.112583302492));
#60702=CARTESIAN_POINT('Ctrl Pts',(14.2062007174671,-2.96922295374568,12.));
#60703=CARTESIAN_POINT('Ctrl Pts',(14.1131167498864,-2.9351724226013,12.));
#60704=CARTESIAN_POINT('Ctrl Pts',(14.0220959175279,-2.89635937351053,12.));
#60705=CARTESIAN_POINT('Ctrl Pts',(13.9333480734334,-2.85311020134011,12.));
#60706=CARTESIAN_POINT('Ctrl Pts',(13.8426550828426,-2.80891310782501,12.));
#60707=CARTESIAN_POINT('Ctrl Pts',(13.7543351402525,-2.76008268621842,12.));
#60708=CARTESIAN_POINT('Ctrl Pts',(13.6686411145779,-2.7069217762808,12.));
#60709=CARTESIAN_POINT('Ctrl Pts',(13.5868027530609,-2.65615275554924,12.));
#60710=CARTESIAN_POINT('Ctrl Pts',(13.5073590893475,-2.60143327816087,12.));
#60711=CARTESIAN_POINT('Ctrl Pts',(13.4305625059366,-2.54299781905995,12.));
#60712=CARTESIAN_POINT('Ctrl Pts',(13.3633654954521,-2.49186679234665,12.));
#60713=CARTESIAN_POINT('Ctrl Pts',(13.298195438544,-2.43789004325195,12.));
#60714=CARTESIAN_POINT('Ctrl Pts',(13.235245315039,-2.38121225533745,12.));
#60715=CARTESIAN_POINT('Ctrl Pts',(13.2201383978307,-2.36761058782836,12.));
#60716=CARTESIAN_POINT('Ctrl Pts',(13.2051557596309,-2.35384973663533,12.));
#60717=CARTESIAN_POINT('Ctrl Pts',(13.1903225084953,-2.33995287271397,12.));
#60718=CARTESIAN_POINT('Ctrl Pts',(13.1178922144325,-2.27209492767057,12.));
#60719=CARTESIAN_POINT('Ctrl Pts',(13.0489277577742,-2.20091637429481,12.));
#60720=CARTESIAN_POINT('Ctrl Pts',(12.9836701413723,-2.12670552844038,12.));
#60721=CARTESIAN_POINT('Ctrl Pts',(12.9187777778625,-2.05291004752833,12.));
#60722=CARTESIAN_POINT('Ctrl Pts',(12.8575503884276,-1.97611533073339,12.));
#60723=CARTESIAN_POINT('Ctrl Pts',(12.800268550456,-1.89657810132058,12.));
#60724=CARTESIAN_POINT('Ctrl Pts',(12.7459133734412,-1.82110461204208,12.));
#60725=CARTESIAN_POINT('Ctrl Pts',(12.6951108248742,-1.74316096291563,12.));
#60726=CARTESIAN_POINT('Ctrl Pts',(12.6481432361601,-1.66295348615981,12.));
#60727=CARTESIAN_POINT('Ctrl Pts',(12.6107661639977,-1.59912392350293,12.));
#60728=CARTESIAN_POINT('Ctrl Pts',(12.5758185286433,-1.533860318552,12.));
#60729=CARTESIAN_POINT('Ctrl Pts',(12.5434639629309,-1.46726456665475,12.));
#60730=CARTESIAN_POINT('Ctrl Pts',(12.5375614518629,-1.45511536440159,12.));
#60731=CARTESIAN_POINT('Ctrl Pts',(12.5317470084536,-1.4429252625298,12.));
#60732=CARTESIAN_POINT('Ctrl Pts',(12.5260248255016,-1.43070222232707,12.));
#60733=CARTESIAN_POINT('Ctrl Pts',(12.4854475610481,-1.34402594180728,12.));
#60734=CARTESIAN_POINT('Ctrl Pts',(12.4494522312093,-1.25558570069036,12.));
#60735=CARTESIAN_POINT('Ctrl Pts',(12.4183023908741,-1.16562505800954,12.));
#60736=CARTESIAN_POINT('Ctrl Pts',(12.3871525505389,-1.07566441532873,12.));
#60737=CARTESIAN_POINT('Ctrl Pts',(12.3608477335802,-0.984182637916221,
12.));
#60738=CARTESIAN_POINT('Ctrl Pts',(12.3397077040223,-0.891413467157708,
12.));
#60739=CARTESIAN_POINT('Ctrl Pts',(12.3185427547458,-0.798534940751147,
12.));
#60740=CARTESIAN_POINT('Ctrl Pts',(12.3025555503081,-0.704364799779564,
12.));
#60741=CARTESIAN_POINT('Ctrl Pts',(12.2916706351494,-0.609311329981899,
12.));
#60742=CARTESIAN_POINT('Ctrl Pts',(12.2861036872675,-0.560697472671795,
12.));
#60743=CARTESIAN_POINT('Ctrl Pts',(12.2818721595795,-0.511852737800975,
12.));
#60744=CARTESIAN_POINT('Ctrl Pts',(12.2789708979829,-0.462833545994333,
12.));
#60745=CARTESIAN_POINT('Ctrl Pts',(12.2781343831999,-0.448699943341852,
12.));
#60746=CARTESIAN_POINT('Ctrl Pts',(12.277408477694,-0.434551848133338,12.));
#60747=CARTESIAN_POINT('Ctrl Pts',(12.2767931065317,-0.42039064034991,12.));
#60748=CARTESIAN_POINT('Ctrl Pts',(12.2761719502385,-0.406096302442059,
12.));
#60749=CARTESIAN_POINT('Ctrl Pts',(12.2756638189297,-0.391797511344244,
12.));
#60750=CARTESIAN_POINT('Ctrl Pts',(12.2752682723578,-0.377498729044968,
12.));
#60751=CARTESIAN_POINT('Ctrl Pts',(12.2726875200461,-0.28420600930709,12.));
#60752=CARTESIAN_POINT('Ctrl Pts',(12.2748931639065,-0.190870392884388,
12.));
#60753=CARTESIAN_POINT('Ctrl Pts',(12.2817566653744,-0.0978690578159151,
12.));
#60754=CARTESIAN_POINT('Ctrl Pts',(12.2886243750566,-0.004810700899435,
12.));
#60755=CARTESIAN_POINT('Ctrl Pts',(12.3001560328895,0.0879139420894839,
12.));
#60756=CARTESIAN_POINT('Ctrl Pts',(12.3162734180046,0.179914286846824,12.));
#60757=CARTESIAN_POINT('Ctrl Pts',(12.3321476400437,0.270526621907842,12.));
#60758=CARTESIAN_POINT('Ctrl Pts',(12.3524707190227,0.360437184721369,12.));
#60759=CARTESIAN_POINT('Ctrl Pts',(12.3772105840448,0.449247114668589,12.));
#60760=CARTESIAN_POINT('Ctrl Pts',(12.387089561874,0.484710175124557,12.));
#60761=CARTESIAN_POINT('Ctrl Pts',(12.3976732487818,0.519997379566271,12.));
#60762=CARTESIAN_POINT('Ctrl Pts',(12.4089613041164,0.555081714039806,12.));
#60763=CARTESIAN_POINT('Ctrl Pts',(12.4149082466012,0.573565368933964,12.));
#60764=CARTESIAN_POINT('Ctrl Pts',(12.4210507056737,0.591992698996559,12.));
#60765=CARTESIAN_POINT('Ctrl Pts',(12.427388732547,0.610359631690939,12.));
#60766=CARTESIAN_POINT('Ctrl Pts',(12.4327450955641,0.62588180617673,12.));
#60767=CARTESIAN_POINT('Ctrl Pts',(12.4382385696775,0.641353302839583,12.));
#60768=CARTESIAN_POINT('Ctrl Pts',(12.4438669442654,0.656766888688516,12.));
#60769=CARTESIAN_POINT('Ctrl Pts',(12.4746822935363,0.741156266835812,12.));
#60770=CARTESIAN_POINT('Ctrl Pts',(12.5095548332415,0.823860554446091,12.));
#60771=CARTESIAN_POINT('Ctrl Pts',(12.5484325218527,0.904509504080283,12.));
#60772=CARTESIAN_POINT('Ctrl Pts',(12.5775387438767,0.964888253895875,12.));
#60773=CARTESIAN_POINT('Ctrl Pts',(12.6088907149234,1.02411455960934,12.));
#60774=CARTESIAN_POINT('Ctrl Pts',(12.6424801735134,1.08201977519688,12.));
#60775=CARTESIAN_POINT('Ctrl Pts',(12.6553986892758,1.10429013833142,12.));
#60776=CARTESIAN_POINT('Ctrl Pts',(12.6686482828058,1.12636495172308,12.));
#60777=CARTESIAN_POINT('Ctrl Pts',(12.6822288987083,1.1482340709878,12.));
#60778=CARTESIAN_POINT('Ctrl Pts',(12.6939913183076,1.16717531480961,12.));
#60779=CARTESIAN_POINT('Ctrl Pts',(12.706004041963,1.18596501264398,12.));
#60780=CARTESIAN_POINT('Ctrl Pts',(12.7182527989854,1.20457528100954,12.));
#60781=CARTESIAN_POINT('Ctrl Pts',(12.765524404259,1.27639785521913,12.));
#60782=CARTESIAN_POINT('Ctrl Pts',(12.8163473248132,1.34561526270953,12.));
#60783=CARTESIAN_POINT('Ctrl Pts',(12.8706925767079,1.41187353983322,12.));
#60784=CARTESIAN_POINT('Ctrl Pts',(12.9128273378038,1.46324466389474,12.));
#60785=CARTESIAN_POINT('Ctrl Pts',(12.9570801591186,1.51283644006015,12.));
#60786=CARTESIAN_POINT('Ctrl Pts',(13.0034499581199,1.56046614478315,12.));
#60787=CARTESIAN_POINT('Ctrl Pts',(13.0293158880168,1.58703487335031,12.));
#60788=CARTESIAN_POINT('Ctrl Pts',(13.0558407610521,1.61299275362867,12.));
#60789=CARTESIAN_POINT('Ctrl Pts',(13.0829974340784,1.63832794503775,12.));
#60790=CARTESIAN_POINT('Origin',(15.,0.,7.5));
#60791=CARTESIAN_POINT('Origin',(-7.5,12.9903810567666,3.));
#60792=CARTESIAN_POINT('Origin',(15.,0.,3.));
#60793=CARTESIAN_POINT('Origin',(-7.50000000000001,-12.9903810567666,3.));
#60794=CARTESIAN_POINT('Origin',(5.55111512312578E-16,0.,14.));
#60795=CARTESIAN_POINT('',(-5.65685424949238,-6.92764844988394E-16,12.));
#60796=CARTESIAN_POINT('Origin',(5.55111512312578E-16,0.,12.));
#60797=CARTESIAN_POINT('',(1.87717472568372E-16,-4.49927934798557E-32,8.));
#60798=CARTESIAN_POINT('Origin',(5.55111512312578E-16,0.,14.));
#60799=CARTESIAN_POINT('Origin',(0.,0.,0.));
#60800=CARTESIAN_POINT('',(-30.,-3.67394039744206E-15,12.));
#60801=CARTESIAN_POINT('Origin',(0.,0.,12.));
#60802=CARTESIAN_POINT('',(-30.,-3.67394039744206E-15,0.));
#60803=CARTESIAN_POINT('',(-30.,-3.67394039744206E-15,0.));
#60804=CARTESIAN_POINT('Origin',(0.,0.,0.));
#60805=CARTESIAN_POINT('Origin',(0.,0.,12.));
#60806=CARTESIAN_POINT('Origin',(0.,0.,0.));
#97442=UNCERTAINTY_MEASURE_WITH_UNIT(LENGTH_MEASURE(0.01),#97476,
'DISTANCE_ACCURACY_VALUE',
'Maximum model space distance between geometric entities at asserted c
onnectivities');
#97452=UNCERTAINTY_MEASURE_WITH_UNIT(LENGTH_MEASURE(0.01),#97476,
'DISTANCE_ACCURACY_VALUE',
'Maximum model space distance between geometric entities at asserted c
onnectivities');
#97465=(
GEOMETRIC_REPRESENTATION_CONTEXT(3)
GLOBAL_UNCERTAINTY_ASSIGNED_CONTEXT((#97442))
GLOBAL_UNIT_ASSIGNED_CONTEXT((#97476,#97478,#97479))
REPRESENTATION_CONTEXT('','3D')
);
#97475=(
GEOMETRIC_REPRESENTATION_CONTEXT(3)
GLOBAL_UNCERTAINTY_ASSIGNED_CONTEXT((#97452))
GLOBAL_UNIT_ASSIGNED_CONTEXT((#97476,#97478,#97479))
REPRESENTATION_CONTEXT('','3D')
);
#97476=(
LENGTH_UNIT()
NAMED_UNIT(*)
SI_UNIT(.MILLI.,.METRE.)
);
#97478=(
NAMED_UNIT(*)
PLANE_ANGLE_UNIT()
SI_UNIT($,.RADIAN.)
);
#97479=(
NAMED_UNIT(*)
SI_UNIT($,.STERADIAN.)
SOLID_ANGLE_UNIT()
);
#97492=SHAPE_DEFINITION_REPRESENTATION(#97554,#97615);
#97554=PRODUCT_DEFINITION_SHAPE('',$,#97638);
#97615=SHAPE_REPRESENTATION('',(#22701),#97465);
#97625=PRODUCT_DEFINITION_CONTEXT('part definition',#97693,'design');
#97638=PRODUCT_DEFINITION('Swivel pad','Swivel pad',#97660,#97625);
#97660=PRODUCT_DEFINITION_FORMATION('',$,#97707);
#97693=APPLICATION_CONTEXT(
'Core Data for Automotive Mechanical Design Process');
#97694=PRODUCT_CONTEXT('part definition',#97693,'mechanical');
#97707=PRODUCT('Swivel pad','Swivel pad',$,(#97694));
#97722=PRESENTATION_STYLE_ASSIGNMENT((#97729));
#97729=SURFACE_STYLE_USAGE(.BOTH.,#97736);
#97736=SURFACE_SIDE_STYLE('',(#97743));
#97743=SURFACE_STYLE_FILL_AREA(#97750);
#97750=FILL_AREA_STYLE('Gray',(#97757));
#97757=FILL_AREA_STYLE_COLOUR('Gray',#97764);
#97764=COLOUR_RGB('Gray',0.407843137254902,0.447058823529412,0.498039215686275);
ENDSEC;
END-ISO-10303-21;
